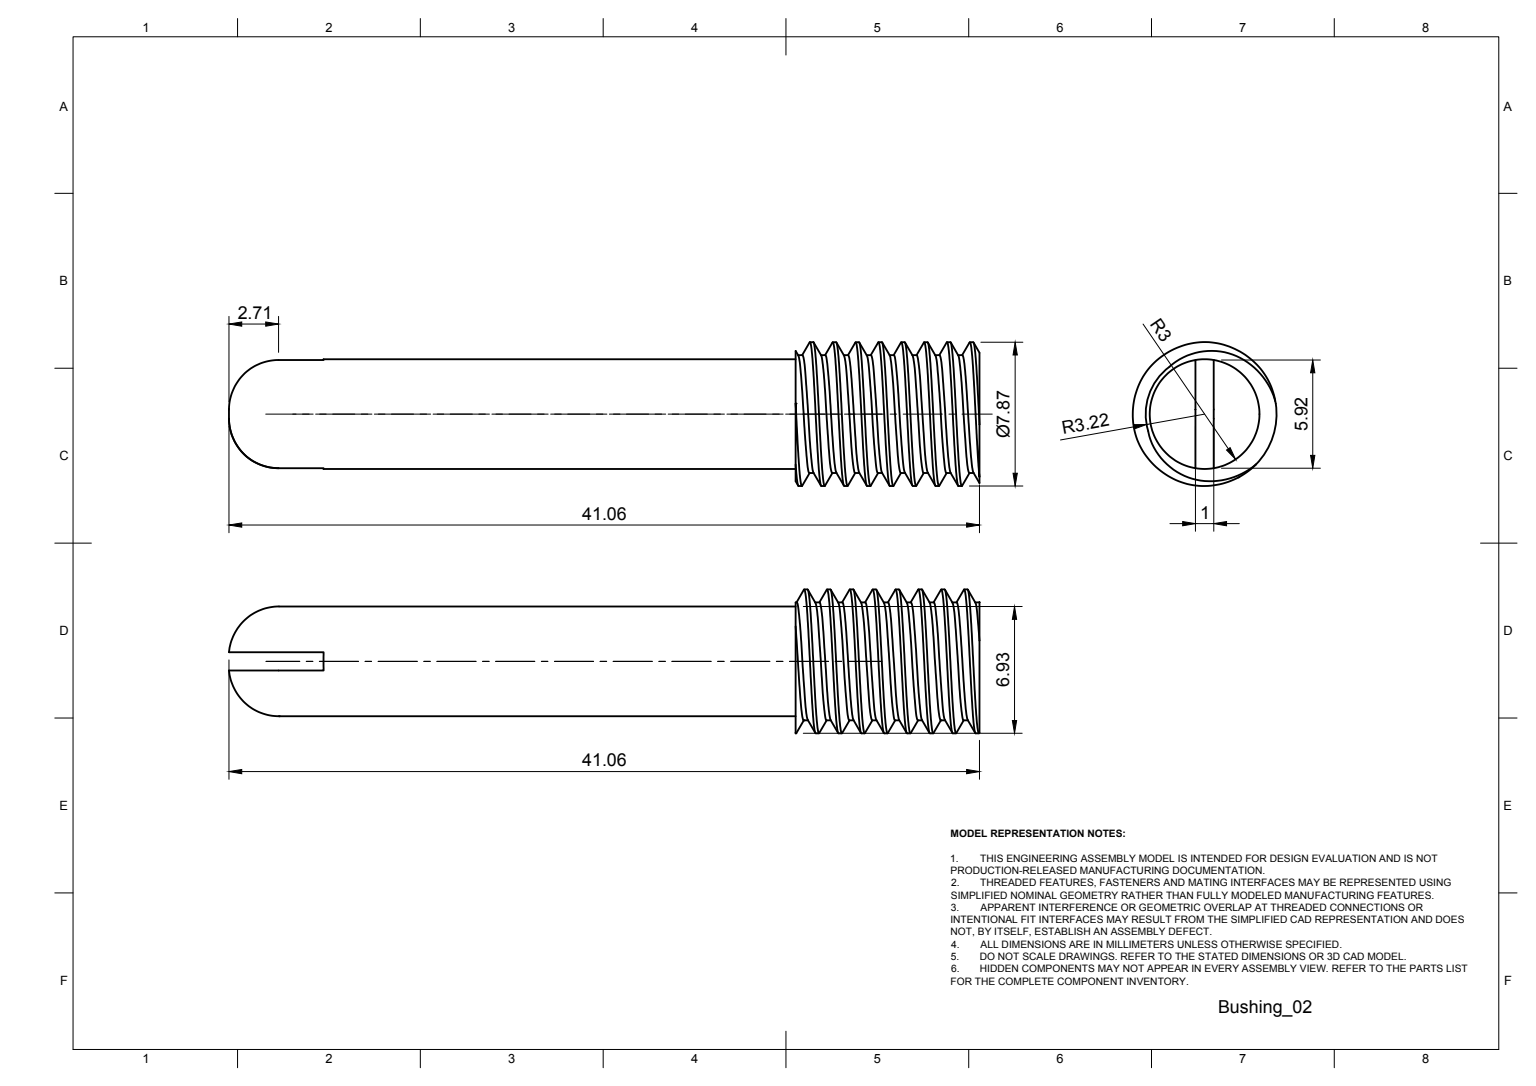
ISO-10303-21;
HEADER;
/* Generated by software containing ST-Developer
 * from STEP Tools, Inc. (www.steptools.com) 
 */

FILE_DESCRIPTION(
/* description */ (''),
/* implementation_level */ '2;1');

FILE_NAME(
/* name */ 'Bushing_02.step',
/* time_stamp */ '2026-10-06T12:52:28-07:00',
/* author */ (''),
/* organization */ (''),
/* preprocessor_version */ 'ST-DEVELOPER v20.2',
/* originating_system */ 'Autodesk Translation Framework v15.15.0.0',
/* authorisation */ '');

FILE_SCHEMA (('AUTOMOTIVE_DESIGN { 1 0 10303 214 3 1 1 }'));
ENDSEC;

DATA;
#10=MECHANICAL_DESIGN_GEOMETRIC_PRESENTATION_REPRESENTATION('',(#78),#34403);
#51=B_SPLINE_SURFACE_WITH_KNOTS('',3,3,((#24901,#24902,#24903,#24904,#24905,
#24906,#24907,#24908,#24909),(#24910,#24911,#24912,#24913,#24914,#24915,
#24916,#24917,#24918),(#24919,#24920,#24921,#24922,#24923,#24924,#24925,
#24926,#24927),(#24928,#24929,#24930,#24931,#24932,#24933,#24934,#24935,
#24936),(#24937,#24938,#24939,#24940,#24941,#24942,#24943,#24944,#24945)),
 .UNSPECIFIED.,.F.,.F.,.F.,(4,1,4),(4,1,1,1,1,1,4),(-2.3129491492736E-5,
0.571428571428571,1.),(-0.0392722361364195,-0.0280568820761978,-0.00562617395575443,
0.00558918010446727,0.016804534164689,0.0280198882249107,0.0392352422851324),
 .UNSPECIFIED.);
#52=B_SPLINE_SURFACE_WITH_KNOTS('',3,3,((#25116,#25117,#25118,#25119,#25120,
#25121,#25122,#25123,#25124,#25125),(#25126,#25127,#25128,#25129,#25130,
#25131,#25132,#25133,#25134,#25135),(#25136,#25137,#25138,#25139,#25140,
#25141,#25142,#25143,#25144,#25145),(#25146,#25147,#25148,#25149,#25150,
#25151,#25152,#25153,#25154,#25155),(#25156,#25157,#25158,#25159,#25160,
#25161,#25162,#25163,#25164,#25165)),.UNSPECIFIED.,.F.,.F.,.F.,(4,1,4),
(4,1,1,1,1,1,1,4),(-2.35337502838191E-5,0.571428571428571,1.),(-0.0392722361364195,
-0.0280568820761979,-0.0168415280159762,-0.00562617395575452,0.00558918010446715,
0.0168045341646888,0.0280198882249105,0.0392352422851322),.UNSPECIFIED.);
#53=B_SPLINE_SURFACE_WITH_KNOTS('',3,3,((#25200,#25201,#25202,#25203,#25204,
#25205,#25206,#25207,#25208,#25209,#25210,#25211,#25212,#25213,#25214,#25215,
#25216,#25217,#25218,#25219,#25220,#25221,#25222,#25223,#25224,#25225,#25226,
#25227,#25228,#25229,#25230,#25231,#25232,#25233,#25234,#25235,#25236,#25237,
#25238,#25239,#25240,#25241,#25242,#25243,#25244,#25245,#25246,#25247,#25248,
#25249,#25250,#25251,#25252,#25253,#25254,#25255),(#25256,#25257,#25258,
#25259,#25260,#25261,#25262,#25263,#25264,#25265,#25266,#25267,#25268,#25269,
#25270,#25271,#25272,#25273,#25274,#25275,#25276,#25277,#25278,#25279,#25280,
#25281,#25282,#25283,#25284,#25285,#25286,#25287,#25288,#25289,#25290,#25291,
#25292,#25293,#25294,#25295,#25296,#25297,#25298,#25299,#25300,#25301,#25302,
#25303,#25304,#25305,#25306,#25307,#25308,#25309,#25310,#25311),(#25312,
#25313,#25314,#25315,#25316,#25317,#25318,#25319,#25320,#25321,#25322,#25323,
#25324,#25325,#25326,#25327,#25328,#25329,#25330,#25331,#25332,#25333,#25334,
#25335,#25336,#25337,#25338,#25339,#25340,#25341,#25342,#25343,#25344,#25345,
#25346,#25347,#25348,#25349,#25350,#25351,#25352,#25353,#25354,#25355,#25356,
#25357,#25358,#25359,#25360,#25361,#25362,#25363,#25364,#25365,#25366,#25367),
(#25368,#25369,#25370,#25371,#25372,#25373,#25374,#25375,#25376,#25377,
#25378,#25379,#25380,#25381,#25382,#25383,#25384,#25385,#25386,#25387,#25388,
#25389,#25390,#25391,#25392,#25393,#25394,#25395,#25396,#25397,#25398,#25399,
#25400,#25401,#25402,#25403,#25404,#25405,#25406,#25407,#25408,#25409,#25410,
#25411,#25412,#25413,#25414,#25415,#25416,#25417,#25418,#25419,#25420,#25421,
#25422,#25423)),.UNSPECIFIED.,.F.,.F.,.F.,(4,4),(4,1,1,1,1,1,1,1,1,1,1,
1,1,1,1,1,1,1,1,1,1,1,1,1,1,1,1,1,1,1,1,1,1,1,1,1,1,1,1,1,1,1,1,1,1,1,1,
1,1,1,1,1,1,4),(-0.000662226835936772,0.0823162805313219),(-97.5343202090122,
-96.5415235325365,-95.5487268560609,-94.5559301795852,-93.5631335031096,
-92.570336826634,-91.5775401501583,-90.5847434736827,-89.591946797207,-88.5991501207314,
-87.6063534442557,-86.6135567677801,-85.6207600913045,-84.6279634148288,
-83.6351667383532,-82.6423700618775,-81.6495733854019,-80.6567767089262,
-79.6639800324506,-78.671183355975,-77.6783866794993,-76.6855900030237,
-75.692793326548,-74.6999966500724,-73.7071999735967,-72.7144032971211,
-71.7216066206455,-70.7288099441698,-69.7360132676942,-68.7432165912185,
-67.7504199147429,-66.7576232382672,-65.7648265617916,-64.772029885316,
-63.7792332088403,-62.7864365323647,-61.793639855889,-60.8008431794134,
-59.8080465029377,-58.8152498264621,-57.8224531499865,-56.8296564735108,
-55.8368597970352,-54.8440631205595,-53.8512664440839,-52.8584697676082,
-51.8656730911326,-50.872876414657,-49.8800797381813,-48.8872830617057,
-47.89448638523,-46.9016897087544,-45.9088930322787,-44.9154341289673),
 .UNSPECIFIED.);
#54=B_SPLINE_SURFACE_WITH_KNOTS('',3,3,((#25626,#25627,#25628,#25629,#25630,
#25631,#25632,#25633,#25634,#25635,#25636,#25637,#25638,#25639,#25640,#25641,
#25642,#25643,#25644,#25645,#25646,#25647,#25648,#25649,#25650,#25651,#25652,
#25653,#25654,#25655,#25656,#25657,#25658,#25659,#25660,#25661,#25662,#25663,
#25664,#25665,#25666,#25667,#25668,#25669,#25670,#25671,#25672,#25673,#25674,
#25675,#25676,#25677,#25678,#25679,#25680,#25681),(#25682,#25683,#25684,
#25685,#25686,#25687,#25688,#25689,#25690,#25691,#25692,#25693,#25694,#25695,
#25696,#25697,#25698,#25699,#25700,#25701,#25702,#25703,#25704,#25705,#25706,
#25707,#25708,#25709,#25710,#25711,#25712,#25713,#25714,#25715,#25716,#25717,
#25718,#25719,#25720,#25721,#25722,#25723,#25724,#25725,#25726,#25727,#25728,
#25729,#25730,#25731,#25732,#25733,#25734,#25735,#25736,#25737),(#25738,
#25739,#25740,#25741,#25742,#25743,#25744,#25745,#25746,#25747,#25748,#25749,
#25750,#25751,#25752,#25753,#25754,#25755,#25756,#25757,#25758,#25759,#25760,
#25761,#25762,#25763,#25764,#25765,#25766,#25767,#25768,#25769,#25770,#25771,
#25772,#25773,#25774,#25775,#25776,#25777,#25778,#25779,#25780,#25781,#25782,
#25783,#25784,#25785,#25786,#25787,#25788,#25789,#25790,#25791,#25792,#25793),
(#25794,#25795,#25796,#25797,#25798,#25799,#25800,#25801,#25802,#25803,
#25804,#25805,#25806,#25807,#25808,#25809,#25810,#25811,#25812,#25813,#25814,
#25815,#25816,#25817,#25818,#25819,#25820,#25821,#25822,#25823,#25824,#25825,
#25826,#25827,#25828,#25829,#25830,#25831,#25832,#25833,#25834,#25835,#25836,
#25837,#25838,#25839,#25840,#25841,#25842,#25843,#25844,#25845,#25846,#25847,
#25848,#25849)),.UNSPECIFIED.,.F.,.F.,.F.,(4,4),(4,1,1,1,1,1,1,1,1,1,1,
1,1,1,1,1,1,1,1,1,1,1,1,1,1,1,1,1,1,1,1,1,1,1,1,1,1,1,1,1,1,1,1,1,1,1,1,
1,1,1,1,1,1,4),(-0.000307057037193035,0.0826748885905267),(-94.2345010139676,
-93.2410420546399,-92.2482453781643,-91.2554487016887,-90.2626520252132,
-89.2698553487376,-88.277058672262,-87.2842619957864,-86.2914653193108,
-85.2986686428353,-84.3058719663597,-83.3130752898841,-82.3202786134085,
-81.327481936933,-80.3346852604574,-79.3418885839818,-78.3490919075062,
-77.3562952310307,-76.3634985545551,-75.3707018780795,-74.3779052016039,
-73.3851085251283,-72.3923118486528,-71.3995151721772,-70.4067184957016,
-69.413921819226,-68.4211251427505,-67.4283284662749,-66.4355317897993,
-65.4427351133237,-64.4499384368482,-63.4571417603726,-62.464345083897,
-61.4715484074214,-60.4787517309458,-59.4859550544703,-58.4931583779947,
-57.5003617015191,-56.5075650250435,-55.514768348568,-54.5219716720924,
-53.5291749956168,-52.5363783191412,-51.5435816426657,-50.5507849661901,
-49.5579882897145,-48.5651916132389,-47.5723949367633,-46.5795982602878,
-45.5868015838122,-44.5940049073366,-43.601208230861,-42.6084115543855,
-41.6156148779099),.UNSPECIFIED.);
#62=SHAPE_REPRESENTATION_RELATIONSHIP('SRR','None',#34440,#70);
#70=ADVANCED_BREP_SHAPE_REPRESENTATION('',(#86),#34400);
#78=STYLED_ITEM('',(#34484),#86);
#86=MANIFOLD_SOLID_BREP('Body1',#4387);
#101=FACE_BOUND('',#839,.T.);
#139=PLANE('',#4595);
#140=PLANE('',#4601);
#141=PLANE('',#4602);
#142=PLANE('',#4603);
#199=CIRCLE('',#4581,3.22275);
#200=CIRCLE('',#4590,3.933);
#201=CIRCLE('',#4591,3.94307276060078);
#202=CIRCLE('',#4592,3.933);
#203=CIRCLE('',#4594,3.22275);
#204=CIRCLE('',#4596,24.5);
#205=CIRCLE('',#4598,3.);
#206=CIRCLE('',#4600,24.5);
#577=FACE_OUTER_BOUND('',#820,.T.);
#578=FACE_OUTER_BOUND('',#821,.T.);
#579=FACE_OUTER_BOUND('',#822,.T.);
#580=FACE_OUTER_BOUND('',#823,.T.);
#581=FACE_OUTER_BOUND('',#824,.T.);
#582=FACE_OUTER_BOUND('',#825,.T.);
#583=FACE_OUTER_BOUND('',#826,.T.);
#584=FACE_OUTER_BOUND('',#827,.T.);
#585=FACE_OUTER_BOUND('',#828,.T.);
#586=FACE_OUTER_BOUND('',#829,.T.);
#587=FACE_OUTER_BOUND('',#830,.T.);
#588=FACE_OUTER_BOUND('',#831,.T.);
#589=FACE_OUTER_BOUND('',#832,.T.);
#590=FACE_OUTER_BOUND('',#833,.T.);
#591=FACE_OUTER_BOUND('',#834,.T.);
#592=FACE_OUTER_BOUND('',#835,.T.);
#593=FACE_OUTER_BOUND('',#836,.T.);
#594=FACE_OUTER_BOUND('',#837,.T.);
#595=FACE_OUTER_BOUND('',#838,.T.);
#596=FACE_OUTER_BOUND('',#840,.T.);
#820=EDGE_LOOP('',(#3083,#3084,#3085,#3086));
#821=EDGE_LOOP('',(#3087,#3088,#3089,#3090,#3091));
#822=EDGE_LOOP('',(#3092,#3093,#3094,#3095,#3096,#3097));
#823=EDGE_LOOP('',(#3098,#3099,#3100,#3101));
#824=EDGE_LOOP('',(#3102,#3103,#3104,#3105,#3106,#3107));
#825=EDGE_LOOP('',(#3108,#3109,#3110,#3111));
#826=EDGE_LOOP('',(#3112,#3113,#3114,#3115,#3116,#3117));
#827=EDGE_LOOP('',(#3118,#3119,#3120,#3121,#3122));
#828=EDGE_LOOP('',(#3123,#3124,#3125,#3126,#3127,#3128,#3129,#3130,#3131,
#3132,#3133,#3134,#3135,#3136,#3137,#3138,#3139,#3140,#3141,#3142,#3143));
#829=EDGE_LOOP('',(#3144,#3145,#3146,#3147,#3148));
#830=EDGE_LOOP('',(#3149,#3150,#3151,#3152));
#831=EDGE_LOOP('',(#3153,#3154,#3155,#3156,#3157,#3158));
#832=EDGE_LOOP('',(#3159,#3160,#3161,#3162,#3163,#3164,#3165,#3166,#3167,
#3168,#3169,#3170));
#833=EDGE_LOOP('',(#3171,#3172,#3173,#3174,#3175));
#834=EDGE_LOOP('',(#3176,#3177,#3178,#3179));
#835=EDGE_LOOP('',(#3180,#3181,#3182,#3183,#3184,#3185));
#836=EDGE_LOOP('',(#3186,#3187,#3188,#3189,#3190,#3191,#3192,#3193,#3194,
#3195,#3196,#3197,#3198,#3199,#3200,#3201,#3202,#3203,#3204,#3205,#3206,
#3207,#3208,#3209,#3210,#3211));
#837=EDGE_LOOP('',(#3212,#3213,#3214,#3215,#3216,#3217,#3218,#3219,#3220,
#3221,#3222,#3223,#3224,#3225,#3226,#3227,#3228,#3229,#3230,#3231,#3232,
#3233,#3234,#3235,#3236,#3237));
#838=EDGE_LOOP('',(#3238,#3239,#3240,#3241,#3242));
#839=EDGE_LOOP('',(#3243));
#840=EDGE_LOOP('',(#3244,#3245,#3246,#3247,#3248));
#1053=LINE('',#19195,#1190);
#1054=LINE('',#19338,#1191);
#1055=LINE('',#19566,#1192);
#1056=LINE('',#19867,#1193);
#1057=LINE('',#20213,#1194);
#1058=LINE('',#20565,#1195);
#1059=LINE('',#20897,#1196);
#1060=LINE('',#21274,#1197);
#1061=LINE('',#24987,#1198);
#1062=LINE('',#24990,#1199);
#1063=LINE('',#24993,#1200);
#1064=LINE('',#25047,#1201);
#1065=LINE('',#25063,#1202);
#1066=LINE('',#25114,#1203);
#1067=LINE('',#25196,#1204);
#1190=VECTOR('',#5246,3.22275);
#1191=VECTOR('',#5251,3.22275);
#1192=VECTOR('',#5254,3.22275);
#1193=VECTOR('',#5257,3.22275);
#1194=VECTOR('',#5260,3.22275);
#1195=VECTOR('',#5263,3.22275);
#1196=VECTOR('',#5266,3.22275);
#1197=VECTOR('',#5269,3.22275);
#1198=VECTOR('',#5282,10.);
#1199=VECTOR('',#5285,10.);
#1200=VECTOR('',#5288,10.);
#1201=VECTOR('',#5291,10.);
#1202=VECTOR('',#5292,10.);
#1203=VECTOR('',#5293,3.);
#1204=VECTOR('',#5296,10.);
#1410=B_SPLINE_CURVE_WITH_KNOTS('',3,(#19197,#19198,#19199,#19200,#19201,
#19202,#19203,#19204,#19205,#19206,#19207,#19208,#19209,#19210,#19211,#19212,
#19213,#19214,#19215,#19216,#19217,#19218,#19219,#19220,#19221,#19222,#19223,
#19224,#19225,#19226,#19227,#19228,#19229,#19230,#19231,#19232,#19233,#19234,
#19235,#19236,#19237,#19238,#19239,#19240,#19241,#19242,#19243,#19244,#19245,
#19246,#19247,#19248,#19249,#19250,#19251,#19252,#19253,#19254,#19255,#19256,
#19257,#19258,#19259,#19260,#19261,#19262,#19263,#19264,#19265,#19266,#19267,
#19268,#19269,#19270,#19271,#19272,#19273,#19274),.UNSPECIFIED.,.F.,.F.,
(4,2,2,2,2,2,2,2,2,2,2,2,2,2,2,2,2,2,2,2,2,2,2,2,2,2,2,2,2,2,2,2,2,2,2,
2,2,2,4),(-0.953586899306873,-0.946224083901339,-0.939681248602814,-0.933646614330381,
-0.924287213729251,-0.88833783922987,-0.804035161913967,-0.788327368237523,
-0.778740839088327,-0.768154224228326,-0.752801038121388,-0.691121741172027,
-0.635518435315854,-0.624462413541429,-0.618082999395715,-0.611911752838689,
-0.60200076655729,-0.589720784215698,-0.562242711762516,-0.486315971197755,
-0.46886052902349,-0.457800984209137,-0.447137732981836,-0.431855739492939,
-0.37573088153337,-0.313542424627404,-0.30302882313823,-0.296702133009702,
-0.290241676772455,-0.279315169359953,-0.265353516421564,-0.230988909071748,
-0.168154569303192,-0.151167359383941,-0.140141098841724,-0.129305786003328,
-0.11338295845748,-0.0538958793772908,-0.00526464879914939),
 .UNSPECIFIED.);
#1411=B_SPLINE_CURVE_WITH_KNOTS('',3,(#19277,#19278,#19279,#19280,#19281,
#19282,#19283,#19284,#19285,#19286,#19287,#19288,#19289,#19290,#19291,#19292,
#19293,#19294,#19295,#19296,#19297,#19298,#19299,#19300,#19301,#19302,#19303,
#19304,#19305,#19306,#19307,#19308,#19309,#19310,#19311,#19312,#19313,#19314,
#19315,#19316,#19317,#19318,#19319,#19320,#19321,#19322,#19323,#19324,#19325,
#19326,#19327,#19328,#19329,#19330,#19331,#19332,#19333,#19334),
 .UNSPECIFIED.,.F.,.F.,(4,3,3,3,3,3,3,3,3,3,3,3,3,3,3,3,3,3,3,4),(-94.2338387311155,
-94.1386227061935,-94.0434628204143,-93.9483368145334,-93.853196460553,
-93.7580426009854,-93.6628550280585,-93.567613507008,-93.4722330639492,
-93.376774672444,-93.2811517509658,-93.2410420546399,-93.1487193791218,
-93.0565224071019,-92.9644252665555,-92.8724021885971,-92.7804134444312,
-92.6884474321017,-92.5964417156794,-92.5246180830661),.UNSPECIFIED.);
#1412=B_SPLINE_CURVE_WITH_KNOTS('',3,(#19339,#19340,#19341,#19342,#19343,
#19344,#19345,#19346,#19347,#19348,#19349,#19350,#19351,#19352,#19353,#19354,
#19355,#19356,#19357,#19358,#19359,#19360,#19361,#19362,#19363,#19364,#19365,
#19366,#19367,#19368,#19369,#19370,#19371,#19372,#19373,#19374,#19375,#19376,
#19377,#19378,#19379,#19380,#19381,#19382,#19383,#19384,#19385,#19386,#19387,
#19388,#19389,#19390,#19391,#19392,#19393,#19394,#19395,#19396,#19397,#19398,
#19399,#19400,#19401,#19402,#19403,#19404,#19405,#19406,#19407,#19408,#19409,
#19410,#19411,#19412,#19413,#19414,#19415,#19416,#19417,#19418,#19419,#19420,
#19421,#19422,#19423,#19424,#19425,#19426,#19427,#19428,#19429,#19430,#19431,
#19432,#19433,#19434,#19435,#19436,#19437,#19438,#19439,#19440,#19441,#19442,
#19443,#19444,#19445,#19446,#19447,#19448,#19449,#19450,#19451,#19452,#19453,
#19454,#19455,#19456,#19457,#19458,#19459,#19460,#19461,#19462,#19463,#19464,
#19465,#19466,#19467,#19468,#19469,#19470,#19471,#19472,#19473,#19474,#19475,
#19476,#19477,#19478,#19479,#19480,#19481,#19482,#19483,#19484,#19485,#19486,
#19487,#19488,#19489,#19490,#19491,#19492,#19493,#19494,#19495,#19496,#19497,
#19498,#19499,#19500,#19501,#19502,#19503,#19504,#19505,#19506),
 .UNSPECIFIED.,.F.,.F.,(4,2,2,2,2,2,2,2,2,2,2,2,2,2,2,2,2,2,2,2,2,2,2,2,
2,2,2,2,2,2,2,2,2,2,2,2,2,2,2,2,2,2,2,2,2,2,2,2,2,2,2,2,2,2,2,2,2,2,2,2,
2,2,2,2,2,2,2,2,2,2,2,2,2,2,2,2,2,2,2,2,2,2,2,4),(-2.98314948647837,-2.92931927299001,
-2.87847831664238,-2.86854692686803,-2.86238048863821,-2.85598188384405,
-2.84491835823975,-2.78906969762543,-2.72775918925124,-2.71234213768023,
-2.70169927312789,-2.69075927697716,-2.67371484620561,-2.60849645012846,
-2.55783247712985,-2.54788253120033,-2.54171277534183,-2.53531903720203,
-2.52428009071603,-2.46776648675201,-2.42715250362434,-2.40830069600736,
-2.39233125418358,-2.38158948252091,-2.37076866644709,-2.35436708268367,
-2.28314135391068,-2.25155038995474,-2.23824842378604,-2.22773649064595,
-2.22145110781181,-2.21594582391548,-2.20632739871659,-2.16701154076078,
-2.11294395468491,-2.0912376827486,-2.07353264494282,-2.06246402564764,
-2.05201402271332,-2.0394863417041,-2.0061953134929,-1.99990582558898,-1.94050245591194,
-1.92231800668791,-1.90911550001101,-1.90229003981063,-1.89634126079205,
-1.88902652801476,-1.86895400933939,-1.80951506282857,-1.77897954822343,
-1.75649112348816,-1.74453409286566,-1.73422264512113,-1.72122725251755,
-1.69233732141656,-1.64649274907083,-1.59931226565268,-1.58749550650159,
-1.58094516716533,-1.57487942726118,-1.5654739075449,-1.52927851683261,
-1.44595504899421,-1.43008910319921,-1.42043269512404,-1.4097841233922,
-1.39436252007387,-1.33286583781343,-1.27719596698061,-1.26611968641952,
-1.25971350417248,-1.25352405459038,-1.24354070919542,-1.23113688245437,
-1.20315529593337,-1.12441168013372,-1.10911634905808,-1.09858349711662,
-1.08760467199154,-1.07043920126136,-1.02023819202142,-0.957986996023974,
-0.953586899306873),.UNSPECIFIED.);
#1413=B_SPLINE_CURVE_WITH_KNOTS('',3,(#19508,#19509,#19510,#19511,#19512,
#19513,#19514,#19515,#19516,#19517,#19518,#19519,#19520,#19521,#19522,#19523,
#19524,#19525,#19526,#19527,#19528,#19529,#19530,#19531,#19532,#19533,#19534,
#19535,#19536,#19537,#19538,#19539,#19540,#19541,#19542,#19543,#19544,#19545,
#19546,#19547,#19548,#19549,#19550,#19551,#19552,#19553),.UNSPECIFIED.,
 .F.,.F.,(4,3,3,3,3,3,3,3,3,3,3,3,3,3,3,4),(-92.5246180830661,-92.4325102353362,
-92.3402421939541,-92.2482453781643,-92.1550137134133,-92.0619070601935,
-91.9688980138682,-91.8759565736399,-91.78305006345,-91.6901538610218,-91.5972433592587,
-91.5042366896818,-91.4111786089953,-91.3179720140179,-91.2554487016887,
-91.106186954104),.UNSPECIFIED.);
#1414=B_SPLINE_CURVE_WITH_KNOTS('',3,(#19554,#19555,#19556,#19557,#19558,
#19559,#19560,#19561,#19562),.UNSPECIFIED.,.F.,.F.,(4,1,1,1,1,1,4),(-91.1061804086756,
-90.2626520252132,-89.2698553487376,-88.277058672262,-87.2842619957864,
-86.2914653193108,-86.2406734486321),.UNSPECIFIED.);
#1415=B_SPLINE_CURVE_WITH_KNOTS('',3,(#19568,#19569,#19570,#19571,#19572,
#19573,#19574,#19575,#19576,#19577,#19578,#19579,#19580,#19581,#19582,#19583,
#19584,#19585,#19586,#19587,#19588,#19589,#19590,#19591,#19592,#19593,#19594,
#19595,#19596,#19597,#19598,#19599,#19600,#19601,#19602,#19603,#19604,#19605,
#19606,#19607,#19608,#19609,#19610,#19611,#19612,#19613,#19614,#19615,#19616,
#19617,#19618,#19619,#19620,#19621,#19622,#19623,#19624,#19625,#19626,#19627,
#19628,#19629,#19630,#19631,#19632,#19633,#19634,#19635,#19636,#19637,#19638,
#19639,#19640,#19641,#19642,#19643,#19644,#19645,#19646,#19647,#19648,#19649,
#19650,#19651,#19652,#19653,#19654,#19655,#19656,#19657,#19658,#19659,#19660,
#19661,#19662,#19663,#19664,#19665,#19666,#19667,#19668,#19669,#19670,#19671,
#19672,#19673,#19674,#19675,#19676,#19677,#19678,#19679,#19680,#19681,#19682,
#19683,#19684,#19685,#19686,#19687,#19688,#19689,#19690,#19691,#19692,#19693,
#19694,#19695),.UNSPECIFIED.,.F.,.F.,(4,2,2,2,2,2,2,2,2,2,2,2,2,2,2,2,2,
2,2,2,2,2,2,2,2,2,2,2,2,2,2,2,2,2,2,2,2,2,2,2,2,2,2,2,2,2,2,2,2,2,2,2,2,
2,2,2,2,2,2,2,2,2,2,4),(-1.57226653739125,-1.5335777974379,-1.51749976800245,
-1.50781260533011,-1.49720443964807,-1.48199362716857,-1.4271100079384,
-1.36376233553656,-1.35299538353744,-1.34665765102371,-1.34044105870802,
-1.33026081848513,-1.28036678994184,-1.21482587221898,-1.19781359925106,
-1.18687887704712,-1.17623012667664,-1.16078436208362,-1.09877281757955,
-1.04367999968674,-1.03258103848034,-1.02617467754542,-1.02001319481398,
-1.01010791778992,-0.958953801785455,-0.894272784649096,-0.877190705715183,
-0.866242485531937,-0.855602583965498,-0.840209857332201,-0.778575631347056,
-0.722936048969459,-0.711861685957521,-0.70546020493503,-0.699294513098806,
-0.689369054767423,-0.677054035431794,-0.649392216624609,-0.572613580933394,
-0.555994727226221,-0.545133285484477,-0.53442622969633,-0.518652195275346,
-0.459429796640774,-0.402070705637716,-0.391076790872994,-0.384691797229376,
-0.378513281994944,-0.368523491494722,-0.356101632547016,-0.328031571970327,
-0.24906421527631,-0.233758461195957,-0.223238986692471,-0.212293433018225,
-0.195226494574182,-0.145648423230977,-0.0814618760384713,-0.070400689902343,
-0.0640018345987939,-0.0578339732759233,-0.0513639077985467,-0.0362287903919722,
-0.000931521656303621),.UNSPECIFIED.);
#1416=B_SPLINE_CURVE_WITH_KNOTS('',3,(#19696,#19697,#19698,#19699,#19700,
#19701,#19702,#19703,#19704,#19705,#19706,#19707,#19708,#19709,#19710,#19711,
#19712,#19713,#19714,#19715,#19716,#19717,#19718,#19719,#19720,#19721,#19722,
#19723,#19724,#19725,#19726,#19727,#19728,#19729,#19730,#19731,#19732,#19733),
 .UNSPECIFIED.,.F.,.F.,(4,2,2,2,2,2,2,2,2,2,2,2,2,2,2,2,2,2,4),(-3.44144283943813,
-3.36915521246843,-3.35372024630458,-3.34307352431673,-3.33213640148464,
-3.31511101176518,-3.24965355552941,-3.19915704516472,-3.18922333268155,
-3.18305637047153,-3.17665726842006,-3.1655942456309,-3.10972609818714,
-3.04842654583021,-3.03301632354937,-3.02237360197422,-3.01142989848601,
-2.99437110190186,-2.98314948647837),.UNSPECIFIED.);
#1417=B_SPLINE_CURVE_WITH_KNOTS('',3,(#19735,#19736,#19737,#19738,#19739),
 .UNSPECIFIED.,.F.,.F.,(4,1,4),(-86.2406734486321,-85.2986686428353,-84.8230031757796),
 .UNSPECIFIED.);
#1418=B_SPLINE_CURVE_WITH_KNOTS('',3,(#19740,#19741,#19742,#19743,#19744,
#19745,#19746,#19747,#19748,#19749,#19750,#19751,#19752,#19753,#19754,#19755,
#19756,#19757,#19758,#19759,#19760,#19761,#19762,#19763,#19764,#19765,#19766,
#19767,#19768,#19769,#19770,#19771,#19772,#19773,#19774,#19775,#19776,#19777,
#19778,#19779,#19780,#19781,#19782,#19783,#19784,#19785,#19786,#19787,#19788,
#19789,#19790,#19791,#19792,#19793,#19794,#19795,#19796,#19797,#19798,#19799,
#19800,#19801,#19802,#19803,#19804,#19805,#19806,#19807,#19808,#19809,#19810,
#19811,#19812,#19813,#19814,#19815,#19816,#19817,#19818,#19819,#19820,#19821,
#19822,#19823,#19824,#19825,#19826,#19827,#19828,#19829,#19830,#19831,#19832,
#19833,#19834,#19835,#19836,#19837,#19838,#19839,#19840,#19841,#19842,#19843,
#19844,#19845,#19846,#19847,#19848,#19849,#19850,#19851,#19852,#19853,#19854,
#19855,#19856,#19857,#19858,#19859,#19860,#19861,#19862,#19863),
 .UNSPECIFIED.,.F.,.F.,(4,2,2,2,2,2,2,2,2,2,2,2,2,2,2,2,2,2,2,2,2,2,2,2,
2,2,2,2,2,2,2,2,2,2,2,2,2,2,2,2,2,2,2,2,2,2,2,2,2,2,2,2,2,2,2,2,2,2,2,2,
2,4),(-4.05949121043388,-4.05121437145667,-4.04065847954402,-4.02381103819477,
-3.95897828953223,-3.90811934396657,-3.89820260742545,-3.8920396257056,
-3.88563807260872,-3.87455861457586,-3.81920431913373,-3.75742003728717,
-3.74201743687854,-3.7313777449435,-3.72043543181097,-3.70337527512879,
-3.63838157000884,-3.58749127890204,-3.5775671792347,-3.57140291795658,
-3.56500278009261,-3.55393200139329,-3.49833852441203,-3.4368258288365,
-3.42140106480513,-3.41075658377407,-3.39981778691892,-3.38278102810115,
-3.31749947334804,-3.26754902845121,-3.25726826635629,-3.25103138547184,
-3.24471713356767,-3.23406214171634,-3.17336971297882,-3.13494613533587,
-3.11665137224682,-3.10103194361361,-3.09035352395009,-3.07946036874197,
-3.06266587013177,-2.99480056759295,-2.94745285384507,-2.93689327516753,
-2.93059879932187,-2.92434353568057,-2.91397336918307,-2.85079466441326,
-2.81356101937502,-2.79557917663882,-2.78015734987967,-2.76951317962702,
-2.75857335392659,-2.74153221996127,-2.67627961911833,-2.62565067878737,
-2.61570117934235,-2.60953128798207,-2.60313694386948,-2.59209545593267,
-2.53566520876919,-2.48818497945327),.UNSPECIFIED.);
#1419=B_SPLINE_CURVE_WITH_KNOTS('',3,(#19868,#19869,#19870,#19871,#19872,
#19873,#19874,#19875,#19876,#19877,#19878,#19879,#19880,#19881,#19882,#19883,
#19884,#19885,#19886,#19887,#19888,#19889,#19890,#19891,#19892,#19893,#19894,
#19895,#19896,#19897,#19898,#19899,#19900,#19901,#19902,#19903,#19904,#19905,
#19906,#19907,#19908,#19909,#19910,#19911,#19912,#19913,#19914,#19915,#19916,
#19917,#19918,#19919,#19920,#19921,#19922,#19923,#19924,#19925,#19926,#19927,
#19928,#19929,#19930,#19931,#19932,#19933,#19934,#19935,#19936,#19937,#19938,
#19939,#19940,#19941,#19942,#19943,#19944,#19945,#19946,#19947,#19948,#19949,
#19950,#19951,#19952,#19953,#19954,#19955,#19956,#19957,#19958,#19959,#19960,
#19961,#19962,#19963,#19964,#19965,#19966,#19967,#19968,#19969,#19970,#19971,
#19972,#19973,#19974,#19975,#19976,#19977,#19978,#19979,#19980,#19981,#19982,
#19983,#19984,#19985,#19986,#19987,#19988,#19989,#19990,#19991,#19992,#19993,
#19994,#19995,#19996,#19997,#19998,#19999,#20000,#20001,#20002,#20003,#20004,
#20005,#20006,#20007,#20008,#20009,#20010,#20011,#20012,#20013,#20014,#20015,
#20016,#20017,#20018,#20019,#20020,#20021,#20022,#20023,#20024,#20025,#20026,
#20027,#20028,#20029,#20030,#20031,#20032,#20033,#20034,#20035,#20036,#20037,
#20038,#20039,#20040,#20041),.UNSPECIFIED.,.F.,.F.,(4,2,2,2,2,2,2,2,2,2,
2,2,2,2,2,2,2,2,2,2,2,2,2,2,2,2,2,2,2,2,2,2,2,2,2,2,2,2,2,2,2,2,2,2,2,2,
2,2,2,2,2,2,2,2,2,2,2,2,2,2,2,2,2,2,2,2,2,2,2,2,2,2,2,2,2,2,2,2,2,2,2,2,
2,2,2,2,4),(-3.60148803627134,-3.59726790795439,-3.59098685437188,-3.58471907313518,
-3.57428766404847,-3.51164348509371,-3.45559099116675,-3.44034678171266,
-3.42973359074539,-3.41875011562731,-3.40147579935169,-3.34043366880226,
-3.30310540362232,-3.28205654415774,-3.27398152357135,-3.26810771974208,
-3.26090656586411,-3.2456415178696,-3.18703553787276,-3.13855425810496,
-3.1216363120744,-3.11072040881662,-3.10018385387515,-3.0847683875459,-3.00651772233112,
-2.97812444519445,-2.96561919642675,-2.95558062126107,-2.94939320865812,
-2.94302219732592,-2.93209232466705,-2.87403556224324,-2.83428541792364,
-2.81565086864161,-2.79981791455114,-2.78910164548746,-2.77825485553291,
-2.76170816630454,-2.69166204680768,-2.65949146606953,-2.64605245758614,
-2.63546067061529,-2.6291595684875,-2.62291078291482,-2.61257177018778,
-2.54912091334469,-2.5120150754806,-2.49406737179312,-2.47866721537971,
-2.46802690006783,-2.45708201518327,-2.4400135557156,-2.37510334330683,
-2.32419385495604,-2.31423984884152,-2.30806912114555,-2.30167618897554,
-2.29064106146257,-2.22197476329415,-2.18871569735013,-2.16492129885298,
-2.15273109663306,-2.1424291067809,-2.12971584634897,-2.10273105378269,
-2.02998606678719,-2.0016293028606,-1.99260960515907,-1.98667066811743,
-1.97999954768792,-1.96758725489158,-1.95090337602745,-1.90211662187695,
-1.85194585632104,-1.8369121508399,-1.82643866908472,-1.81542316901591,
-1.79798287416363,-1.74547920414441,-1.68411033096761,-1.67352430836737,
-1.66722415648816,-1.66097373936419,-1.65062802104306,-1.63760890563595,
-1.60717731235625,-1.57226653739125),.UNSPECIFIED.);
#1420=B_SPLINE_CURVE_WITH_KNOTS('',3,(#20042,#20043,#20044,#20045,#20046,
#20047,#20048,#20049,#20050,#20051,#20052,#20053,#20054,#20055,#20056,#20057,
#20058,#20059,#20060,#20061,#20062,#20063,#20064,#20065,#20066,#20067,#20068,
#20069,#20070,#20071,#20072,#20073,#20074,#20075,#20076,#20077,#20078,#20079,
#20080,#20081,#20082,#20083,#20084,#20085,#20086,#20087,#20088,#20089,#20090,
#20091,#20092,#20093,#20094,#20095,#20096,#20097,#20098,#20099,#20100,#20101,
#20102,#20103,#20104,#20105,#20106,#20107,#20108,#20109,#20110,#20111,#20112,
#20113,#20114,#20115,#20116,#20117,#20118,#20119,#20120,#20121,#20122,#20123,
#20124,#20125,#20126,#20127,#20128,#20129,#20130,#20131,#20132,#20133,#20134,
#20135,#20136,#20137,#20138,#20139,#20140,#20141,#20142,#20143,#20144,#20145,
#20146,#20147,#20148,#20149,#20150,#20151,#20152,#20153,#20154,#20155,#20156,
#20157,#20158,#20159,#20160,#20161,#20162,#20163,#20164,#20165,#20166,#20167,
#20168,#20169,#20170,#20171,#20172,#20173,#20174,#20175,#20176,#20177,#20178,
#20179,#20180,#20181,#20182,#20183,#20184,#20185,#20186,#20187,#20188,#20189,
#20190,#20191,#20192,#20193,#20194,#20195,#20196,#20197,#20198,#20199,#20200,
#20201,#20202,#20203,#20204,#20205,#20206,#20207,#20208,#20209),
 .UNSPECIFIED.,.F.,.F.,(4,2,2,2,2,2,2,2,2,2,2,2,2,2,2,2,2,2,2,2,2,2,2,2,
2,2,2,2,2,2,2,2,2,2,2,2,2,2,2,2,2,2,2,2,2,2,2,2,2,2,2,2,2,2,2,2,2,2,2,2,
2,2,2,2,2,2,2,2,2,2,2,2,2,2,2,2,2,2,2,2,2,2,2,4),(-2.48818497945327,-2.47661569284377,
-2.46041249231985,-2.44962867574266,-2.43885292257533,-2.42269402150062,
-2.34963196044359,-2.31891957880817,-2.30583089242212,-2.29544489121947,
-2.28918621756621,-2.28289464564112,-2.27235029868863,-2.21067864367937,
-2.15559329660223,-2.13955930085061,-2.12880625929744,-2.11799874145444,
-2.10166705448592,-2.02990196306529,-1.98730851207629,-1.97573932437658,
-1.96923692158684,-1.96314080965402,-1.95357264272231,-1.91386818576171,
-1.83704171514185,-1.81996554507048,-1.80901875051122,-1.79837854665767,
-1.78298224522728,-1.76503910564669,-1.72795555566859,-1.66437608378914,
-1.6540447671092,-1.64779725241036,-1.64149351545674,-1.63089127738814,
-1.61743622842379,-1.58519570479033,-1.51535388396843,-1.49878885307633,
-1.48793790926569,-1.47722314628574,-1.46140326307786,-1.40103999361036,
-1.3450610657836,-1.33399883001431,-1.32760001200728,-1.32143274143006,
-1.31149835160373,-1.26082229040495,-1.19564760626722,-1.17860471563187,
-1.16766389105049,-1.15701870553694,-1.14159547110918,-1.1236100980696,
-1.08636972622046,-1.02311542409142,-1.01274592372879,-1.00649036762245,
-1.00019460847225,-0.989631608162483,-0.941721342655347,-0.874629750026393,
-0.857760383650131,-0.846852232066049,-0.836182940761279,-0.820621411802712,
-0.761154441683342,-0.703549270177194,-0.692574275383058,-0.686193266407756,
-0.680011710962549,-0.670006535853517,-0.657558990906142,-0.629389598384432,
-0.550666233097892,-0.535325340491625,-0.524799982685431,-0.513863175707245,
-0.496842297440668,-0.458703963070235),.UNSPECIFIED.);
#1421=B_SPLINE_CURVE_WITH_KNOTS('',3,(#20215,#20216,#20217,#20218,#20219,
#20220,#20221,#20222,#20223,#20224,#20225,#20226,#20227,#20228,#20229,#20230,
#20231,#20232,#20233,#20234,#20235,#20236,#20237,#20238,#20239,#20240,#20241,
#20242,#20243,#20244,#20245,#20246,#20247,#20248,#20249,#20250,#20251,#20252,
#20253,#20254,#20255,#20256,#20257,#20258,#20259,#20260,#20261,#20262,#20263,
#20264,#20265,#20266,#20267,#20268,#20269,#20270,#20271,#20272,#20273,#20274,
#20275,#20276,#20277,#20278,#20279,#20280,#20281,#20282,#20283,#20284,#20285,
#20286,#20287,#20288,#20289,#20290,#20291,#20292,#20293,#20294,#20295,#20296,
#20297,#20298,#20299,#20300,#20301,#20302,#20303,#20304,#20305,#20306,#20307,
#20308,#20309,#20310,#20311,#20312,#20313,#20314,#20315,#20316,#20317,#20318,
#20319,#20320,#20321,#20322,#20323,#20324,#20325,#20326,#20327,#20328,#20329,
#20330,#20331,#20332,#20333,#20334,#20335,#20336,#20337,#20338,#20339,#20340,
#20341,#20342,#20343,#20344,#20345,#20346,#20347,#20348),.UNSPECIFIED.,
 .F.,.F.,(4,2,2,2,2,2,2,2,2,2,2,2,2,2,2,2,2,2,2,2,2,2,2,2,2,2,2,2,2,2,2,
2,2,2,2,2,2,2,2,2,2,2,2,2,2,2,2,2,2,2,2,2,2,2,2,2,2,2,2,2,2,2,2,2,2,2,4),
(-1.57270504429441,-1.57198597895571,-1.53184015506289,-1.4744178950004,
-1.46342781057866,-1.45704342558984,-1.4508638651289,-1.44086999371776,
-1.42844156890585,-1.40034729366256,-1.32143087815656,-1.30611622816268,
-1.29559480540958,-1.28465062268848,-1.26759324916272,-1.21809184782572,
-1.15729158777298,-1.14419135132274,-1.13738539355418,-1.13142607440303,
-1.12265609486979,-1.09531100949502,-1.03125066260997,-0.997509615877714,
-0.98493246552515,-0.974472652709664,-0.963426589679085,-0.945834993848146,
-0.924318436015176,-0.871329842578893,-0.830426302826506,-0.820785203293156,
-0.815276889046202,-0.808998247382131,-0.798520016701879,-0.785277148103801,
-0.753931042657932,-0.682243191223101,-0.665904305115668,-0.655094053629165,
-0.64433973007818,-0.628306893505015,-0.574149269053255,-0.511174379321276,
-0.500769824530627,-0.494506480797386,-0.488217178586173,-0.477687892439614,
-0.428977275730074,-0.362775320398643,-0.345817247349719,-0.334891381242875,
-0.324232895492104,-0.308739200514757,-0.290643425545204,-0.252992014084021,
-0.190575699323686,-0.180106656871352,-0.173829923488554,-0.167554150248785,
-0.157090098128878,-0.109028173875831,-0.0418274175576785,-0.0252966452826552,
-0.0143328742967741,-0.00723065120931022,-0.000931044346426293),
 .UNSPECIFIED.);
#1422=B_SPLINE_CURVE_WITH_KNOTS('',3,(#20349,#20350,#20351,#20352,#20353,
#20354,#20355,#20356,#20357,#20358,#20359,#20360,#20361,#20362,#20363,#20364,
#20365,#20366,#20367,#20368,#20369,#20370,#20371,#20372,#20373,#20374,#20375,
#20376,#20377,#20378,#20379,#20380,#20381,#20382,#20383,#20384,#20385,#20386),
 .UNSPECIFIED.,.F.,.F.,(4,2,2,2,2,2,2,2,2,2,2,2,2,2,2,2,2,2,4),(-4.05940163546454,
-4.0513614597985,-4.03929124303463,-3.97799719175202,-3.92748437027949,
-3.91747126369622,-3.91128897983749,-3.90491163882794,-3.89395098991898,
-3.83625920142476,-3.7778835028167,-3.76189126289714,-3.75114653873282,
-3.74033227188704,-3.72395993843194,-3.6525226917305,-3.62103886952059,
-3.60776360891426,-3.60148803627134),.UNSPECIFIED.);
#1423=B_SPLINE_CURVE_WITH_KNOTS('',3,(#20388,#20389,#20390,#20391,#20392,
#20393,#20394,#20395,#20396,#20397,#20398,#20399,#20400,#20401,#20402,#20403,
#20404,#20405,#20406,#20407,#20408,#20409,#20410,#20411,#20412,#20413,#20414,
#20415,#20416,#20417,#20418,#20419,#20420,#20421,#20422,#20423,#20424,#20425,
#20426,#20427,#20428,#20429,#20430,#20431,#20432,#20433),.UNSPECIFIED.,
 .F.,.F.,(4,2,2,2,2,2,2,2,2,2,2,2,2,2,2,2,2,2,2,2,2,2,4),(-0.458703963070235,
-0.4476103789344,-0.387390603287348,-0.373726897302928,-0.36681426866366,
-0.36088624078785,-0.352333693779791,-0.32719823278997,-0.274608647504632,
-0.229055324726366,-0.214134235080965,-0.203677569512926,-0.19262737818266,
-0.175011958392165,-0.153454737042513,-0.140085221830007,-0.0719338954249617,
-0.0547956271046257,-0.0472815868163417,-0.0414267321571205,-0.0356813677969033,
-0.0279552207881814,-0.000930590274443855),.UNSPECIFIED.);
#1424=B_SPLINE_CURVE_WITH_KNOTS('',3,(#20434,#20435,#20436,#20437,#20438,
#20439,#20440,#20441,#20442,#20443,#20444,#20445,#20446,#20447,#20448,#20449,
#20450,#20451,#20452,#20453,#20454,#20455,#20456,#20457,#20458,#20459,#20460,
#20461,#20462,#20463,#20464,#20465,#20466,#20467,#20468,#20469,#20470,#20471,
#20472,#20473,#20474,#20475,#20476,#20477,#20478,#20479,#20480,#20481,#20482,
#20483,#20484,#20485,#20486,#20487,#20488,#20489,#20490,#20491,#20492,#20493,
#20494,#20495,#20496,#20497,#20498,#20499,#20500,#20501,#20502,#20503,#20504,
#20505,#20506,#20507,#20508,#20509,#20510,#20511,#20512,#20513,#20514,#20515,
#20516,#20517,#20518,#20519,#20520,#20521,#20522,#20523,#20524,#20525,#20526,
#20527,#20528,#20529,#20530,#20531,#20532,#20533,#20534,#20535,#20536,#20537,
#20538,#20539,#20540,#20541,#20542,#20543,#20544,#20545,#20546,#20547,#20548,
#20549,#20550,#20551,#20552,#20553,#20554,#20555,#20556,#20557,#20558,#20559,
#20560,#20561),.UNSPECIFIED.,.F.,.F.,(4,2,2,2,2,2,2,2,2,2,2,2,2,2,2,2,2,
2,2,2,2,2,2,2,2,2,2,2,2,2,2,2,2,2,2,2,2,2,2,2,2,2,2,2,2,2,2,2,2,2,2,2,2,
2,2,2,2,2,2,2,2,2,2,4),(-4.06048203363518,-4.03025455645395,-3.9691349538326,
-3.95369424520963,-3.94304683352945,-3.9321116200381,-3.91509476425701,
-3.84955218125704,-3.79933143232759,-3.78929737786332,-3.78311059686391,
-3.77673781623578,-3.76580068005654,-3.70782017083285,-3.64915364962081,
-3.63340707851152,-3.62270589410659,-3.61184022793493,-3.59519396745887,
-3.51842926964027,-3.49076501195105,-3.47844946162652,-3.46852477553194,
-3.46235979182168,-3.45595900217838,-3.44488608818992,-3.3893318418027,
-3.32767918035704,-3.31229691148376,-3.30165956012622,-3.29071002293352,
-3.27361754916669,-3.19683072234816,-3.16975298762487,-3.15243990351045,
-3.14489903546282,-3.13962441374937,-3.13230314338034,-3.11633927545952,
-3.05838609218079,-3.0101994379,-2.99332016806537,-2.98241057334082,-2.97186714936823,
-2.95641724351904,-2.87838180616511,-2.83655159525338,-2.82690302107234,
-2.82079166632169,-2.81431345858978,-2.80286356868832,-2.75024228454491,
-2.68747732350124,-2.67156813817421,-2.66083741428753,-2.65000483326521,
-2.63353877133443,-2.55649529326159,-2.52876569107145,-2.51643269276606,
-2.50649735215666,-2.50033001830562,-2.49393150688731,-2.48879418648611),
 .UNSPECIFIED.);
#1425=B_SPLINE_CURVE_WITH_KNOTS('',3,(#20566,#20567,#20568,#20569,#20570,
#20571,#20572,#20573,#20574,#20575,#20576,#20577,#20578,#20579,#20580,#20581,
#20582,#20583,#20584,#20585,#20586,#20587,#20588,#20589,#20590,#20591,#20592,
#20593,#20594,#20595,#20596,#20597,#20598,#20599,#20600,#20601,#20602,#20603,
#20604,#20605,#20606,#20607,#20608,#20609,#20610,#20611,#20612,#20613,#20614,
#20615,#20616,#20617,#20618,#20619,#20620,#20621,#20622,#20623,#20624,#20625,
#20626,#20627,#20628,#20629,#20630,#20631,#20632,#20633,#20634,#20635,#20636,
#20637,#20638,#20639,#20640,#20641,#20642,#20643,#20644,#20645,#20646,#20647,
#20648,#20649,#20650,#20651,#20652,#20653,#20654,#20655,#20656,#20657,#20658,
#20659,#20660,#20661,#20662,#20663,#20664,#20665,#20666,#20667,#20668,#20669,
#20670,#20671,#20672,#20673,#20674,#20675,#20676,#20677,#20678,#20679,#20680,
#20681,#20682,#20683,#20684,#20685,#20686,#20687,#20688,#20689,#20690,#20691,
#20692,#20693,#20694,#20695,#20696,#20697,#20698,#20699,#20700,#20701,#20702,
#20703,#20704,#20705,#20706,#20707,#20708,#20709,#20710,#20711,#20712,#20713,
#20714,#20715,#20716,#20717,#20718,#20719,#20720,#20721,#20722,#20723,#20724,
#20725,#20726,#20727),.UNSPECIFIED.,.F.,.F.,(4,2,2,2,2,2,2,2,2,2,2,2,2,
2,2,2,2,2,2,2,2,2,2,2,2,2,2,2,2,2,2,2,2,2,2,2,2,2,2,2,2,2,2,2,2,2,2,2,2,
2,2,2,2,2,2,2,2,2,2,2,2,2,2,2,2,2,2,2,2,2,2,2,2,2,2,2,2,2,2,2,4),(-3.60242287809638,
-3.56721784695233,-3.55156189813843,-3.54087604581589,-3.52998929297132,
-3.51323412204218,-3.44497013969903,-3.39791346110271,-3.38735473125302,
-3.38105987829509,-3.37480333375927,-3.36442970316565,-3.30125673265392,
-3.26400908284791,-3.2460223081981,-3.23059678410155,-3.21995088869975,
-3.20900998526235,-3.19196872439598,-3.12667495572608,-3.07633231876972,
-3.06624290939729,-3.060044392539,-3.05368405300464,-3.04281000897509,-2.98411981411094,
-2.92597258491712,-2.91024653188731,-2.89954788321163,-2.88867582073824,
-2.87200116277746,-2.79526113514378,-2.7676005695254,-2.75528520035583,
-2.74536024613777,-2.73919461687122,-2.73279268291657,-2.72171705169384,
-2.66617790190046,-2.6045148723875,-2.58911903845016,-2.5784782235403,-2.56752998187024,
-2.55045013455705,-2.4856433040347,-2.43459781081709,-2.42465866485077,
-2.4184902403953,-2.41209205800306,-2.40103454940899,-2.34495831573944,
-2.2838783420997,-2.26844777215121,-2.25780098835939,-2.24686128134125,
-2.22982643444661,-2.15269523980569,-2.11311651180288,-2.1035514946851,
-2.09745561068995,-2.09095128173895,-2.07937494247329,-2.03104486686402,
-1.96667113596343,-1.94956534772693,-1.93861223520825,-1.92797478084316,
-1.9125987156333,-1.84933732086722,-1.79562684674695,-1.78435791261974,
-1.77791627132938,-1.77177925894983,-1.76200059891485,-1.71521190961271,
-1.64467016553331,-1.62818656919652,-1.6173497828642,-1.60662021642605,
-1.59072325636642,-1.57270504429441),.UNSPECIFIED.);
#1426=B_SPLINE_CURVE_WITH_KNOTS('',3,(#20728,#20729,#20730,#20731,#20732,
#20733,#20734,#20735,#20736,#20737,#20738,#20739,#20740,#20741,#20742,#20743,
#20744,#20745,#20746,#20747,#20748,#20749,#20750,#20751,#20752,#20753,#20754,
#20755,#20756,#20757,#20758,#20759,#20760,#20761,#20762,#20763,#20764,#20765,
#20766,#20767,#20768,#20769,#20770,#20771,#20772,#20773,#20774,#20775,#20776,
#20777,#20778,#20779,#20780,#20781,#20782,#20783,#20784,#20785,#20786,#20787,
#20788,#20789,#20790,#20791,#20792,#20793,#20794,#20795,#20796,#20797,#20798,
#20799,#20800,#20801,#20802,#20803,#20804,#20805,#20806,#20807,#20808,#20809,
#20810,#20811,#20812,#20813,#20814,#20815,#20816,#20817,#20818,#20819,#20820,
#20821,#20822,#20823,#20824,#20825,#20826,#20827,#20828,#20829,#20830,#20831,
#20832,#20833,#20834,#20835,#20836,#20837,#20838,#20839,#20840,#20841,#20842,
#20843,#20844,#20845,#20846,#20847,#20848,#20849,#20850,#20851,#20852,#20853,
#20854,#20855,#20856,#20857,#20858,#20859,#20860,#20861,#20862,#20863,#20864,
#20865,#20866,#20867,#20868,#20869,#20870,#20871,#20872,#20873,#20874,#20875,
#20876,#20877,#20878,#20879,#20880,#20881,#20882,#20883,#20884,#20885,#20886,
#20887,#20888,#20889,#20890,#20891,#20892,#20893),.UNSPECIFIED.,.F.,.F.,
(4,2,2,2,2,2,2,2,2,2,2,2,2,2,2,2,2,2,2,2,2,2,2,2,2,2,2,2,2,2,2,2,2,2,2,
2,2,2,2,2,2,2,2,2,2,2,2,2,2,2,2,2,2,2,2,2,2,2,2,2,2,2,2,2,2,2,2,2,2,2,2,
2,2,2,2,2,2,2,2,2,2,2,4),(-2.48879418648611,-2.482870786226,-2.42692956343107,
-2.36600785850896,-2.35045675318813,-2.33978959585287,-2.33016094885262,
-2.31444582835103,-2.23821710940245,-2.19523975059826,-2.1855542992085,
-2.17943580816656,-2.17296831262753,-2.16157124617673,-2.11118827433854,
-2.06704068844034,-2.04734877497841,-2.0308590398503,-2.02002175028717,
-2.00929425375571,-1.99340524118733,-1.97468006647316,-1.93457908581669,
-1.87709109853615,-1.86610750722511,-1.85972480069881,-1.85354479225751,
-1.84354696670865,-1.79297932372389,-1.72782025145022,-1.71077564213425,
-1.69983433429665,-1.6891891139229,-1.67376662544518,-1.65578255957856,
-1.61854770167534,-1.55527893663139,-1.54491074496027,-1.53865537392209,
-1.53235915546231,-1.52179434822374,-1.47368194101312,-1.40684450290551,
-1.38994962777,-1.37903651957945,-1.36837058921596,-1.3528291953071,-1.29288180784992,
-1.2357731213652,-1.2247627523323,-1.21837436650977,-1.21219837856251,-1.20222149130216,
-1.18982109384957,-1.16183326387008,-1.08267697612122,-1.06740015276224,
-1.05688543352747,-1.0459323793008,-1.02882628372556,-0.978950224072073,
-0.917329280997904,-0.905017534155332,-0.898365664895021,-0.892347412696423,
-0.883212145366521,-0.851369147050279,-0.8063673714056,-0.761177170046655,
-0.74626846473054,-0.735813488995268,-0.724759123042586,-0.707123289176841,
-0.685531949518534,-0.632133201827475,-0.591798795701873,-0.582163133943164,
-0.576655828465875,-0.570375876223591,-0.559890990576539,-0.546636681512379,
-0.51524224622991,-0.45931701754657),.UNSPECIFIED.);
#1427=B_SPLINE_CURVE_WITH_KNOTS('',3,(#20899,#20900,#20901,#20902,#20903,
#20904,#20905,#20906,#20907,#20908,#20909,#20910,#20911,#20912,#20913,#20914,
#20915,#20916,#20917,#20918,#20919,#20920,#20921,#20922,#20923,#20924,#20925,
#20926,#20927,#20928,#20929,#20930,#20931,#20932,#20933,#20934,#20935,#20936,
#20937,#20938,#20939,#20940,#20941,#20942,#20943,#20944,#20945,#20946,#20947,
#20948,#20949,#20950,#20951,#20952,#20953,#20954,#20955,#20956,#20957,#20958,
#20959,#20960,#20961,#20962,#20963,#20964,#20965,#20966,#20967,#20968,#20969,
#20970,#20971,#20972,#20973,#20974,#20975,#20976,#20977,#20978,#20979,#20980,
#20981,#20982,#20983,#20984,#20985,#20986,#20987,#20988,#20989,#20990,#20991,
#20992,#20993,#20994,#20995,#20996,#20997,#20998,#20999,#21000,#21001,#21002,
#21003,#21004,#21005,#21006,#21007,#21008,#21009,#21010,#21011,#21012,#21013,
#21014,#21015,#21016,#21017,#21018,#21019,#21020,#21021,#21022,#21023,#21024),
 .UNSPECIFIED.,.F.,.F.,(4,2,2,2,2,2,2,2,2,2,2,2,2,2,2,2,2,2,2,2,2,2,2,2,
2,2,2,2,2,2,2,2,2,2,2,2,2,2,2,2,2,2,2,2,2,2,2,2,2,2,2,2,2,2,2,2,2,2,2,2,
2,2,4),(-1.57273988019061,-1.56691346024312,-1.56072898385932,-1.55070573887629,
-1.50842406317083,-1.43222502173132,-1.41651494897745,-1.4068881047619,
-1.39622185106329,-1.38067029519754,-1.31828553824896,-1.26392823496632,
-1.25275991015442,-1.24633978848889,-1.24018924744267,-1.23033879598207,
-1.1760008817155,-1.11477371714702,-1.09750587349208,-1.08652241989586,
-1.07590625961537,-1.06065247806019,-1.00441058913554,-0.941945479199864,
-0.931484916050102,-0.925210316360724,-0.918933749330253,-0.90846320995488,
-0.895232867586938,-0.863935841053784,-0.792164412777069,-0.775839821530913,
-0.765033207159675,-0.754278155395765,-0.738235749766936,-0.682680727504737,
-0.621535654361532,-0.610922418914989,-0.604616329925545,-0.598370659077198,
-0.588049362231943,-0.575071819605588,-0.544810450900195,-0.470830069515804,
-0.454802593626465,-0.445123229273891,-0.434506544974243,-0.419248850028895,
-0.362877812031364,-0.300576688829507,-0.290096385595649,-0.283817819462706,
-0.277545348773213,-0.26709499646107,-0.253899067128589,-0.222745178504822,
-0.150669428219029,-0.134383624062453,-0.123583848906434,-0.112821487766765,
-0.0967404810140852,-0.0777076763684024,-0.000936417546807567),
 .UNSPECIFIED.);
#1428=B_SPLINE_CURVE_WITH_KNOTS('',3,(#21025,#21026,#21027,#21028,#21029,
#21030,#21031,#21032,#21033,#21034,#21035,#21036,#21037,#21038,#21039,#21040,
#21041,#21042,#21043,#21044,#21045,#21046,#21047,#21048,#21049,#21050,#21051,
#21052,#21053,#21054,#21055,#21056,#21057,#21058,#21059,#21060,#21061,#21062,
#21063,#21064,#21065,#21066),.UNSPECIFIED.,.F.,.F.,(4,2,2,2,2,2,2,2,2,2,
2,2,2,2,2,2,2,2,2,2,4),(-4.06024511832612,-4.04416917649443,-4.03341342658371,
-4.02723973391658,-4.02172518011229,-4.01522137623075,-4.00364660759717,
-3.94883815801512,-3.88741519438322,-3.87198632035072,-3.86134018065844,
-3.85040070853188,-3.83336531020972,-3.76801068386381,-3.71745087900611,
-3.70750155272622,-3.70133131022163,-3.69493621368035,-3.68389271615082,
-3.62747426988344,-3.60242287809638),.UNSPECIFIED.);
#1429=B_SPLINE_CURVE_WITH_KNOTS('',3,(#21068,#21069,#21070,#21071,#21072,
#21073,#21074,#21075,#21076,#21077,#21078,#21079,#21080,#21081,#21082,#21083,
#21084,#21085,#21086,#21087,#21088,#21089,#21090,#21091,#21092,#21093,#21094,
#21095,#21096,#21097,#21098,#21099,#21100,#21101,#21102,#21103,#21104,#21105,
#21106,#21107),.UNSPECIFIED.,.F.,.F.,(4,2,2,2,2,2,2,2,2,2,2,2,2,2,2,2,2,
2,2,4),(-0.45931701754657,-0.443662955116037,-0.427311208082828,-0.416498713796264,
-0.405746798310332,-0.389726540866301,-0.331854426135855,-0.273525442235887,
-0.262610494918398,-0.256241478612075,-0.250049205834386,-0.239992621745995,
-0.227459807822531,-0.198962724177927,-0.121968714348891,-0.106068905204749,
-0.0964095104727434,-0.0857712360881861,-0.0703931358704458,-0.000931723441433497),
 .UNSPECIFIED.);
#1430=B_SPLINE_CURVE_WITH_KNOTS('',3,(#21108,#21109,#21110,#21111,#21112,
#21113,#21114,#21115,#21116,#21117,#21118,#21119,#21120,#21121,#21122,#21123,
#21124,#21125,#21126,#21127,#21128,#21129,#21130,#21131,#21132,#21133,#21134,
#21135,#21136,#21137,#21138,#21139,#21140,#21141,#21142,#21143,#21144,#21145,
#21146,#21147,#21148,#21149,#21150,#21151,#21152,#21153,#21154,#21155,#21156,
#21157,#21158,#21159,#21160,#21161,#21162,#21163,#21164,#21165,#21166,#21167,
#21168,#21169,#21170,#21171,#21172,#21173,#21174,#21175,#21176,#21177,#21178,
#21179,#21180,#21181,#21182,#21183,#21184,#21185,#21186,#21187,#21188,#21189,
#21190,#21191,#21192,#21193,#21194,#21195,#21196,#21197,#21198,#21199,#21200,
#21201,#21202,#21203,#21204,#21205,#21206,#21207,#21208,#21209,#21210,#21211,
#21212,#21213,#21214,#21215,#21216,#21217,#21218,#21219,#21220,#21221,#21222,
#21223,#21224,#21225,#21226,#21227,#21228,#21229,#21230,#21231,#21232,#21233,
#21234,#21235,#21236,#21237,#21238,#21239,#21240,#21241,#21242,#21243,#21244,
#21245,#21246,#21247,#21248,#21249,#21250,#21251,#21252,#21253,#21254,#21255,
#21256,#21257,#21258,#21259,#21260,#21261,#21262,#21263,#21264,#21265,#21266,
#21267,#21268,#21269,#21270),.UNSPECIFIED.,.F.,.F.,(4,3,3,3,3,3,3,3,3,3,
3,3,3,3,3,3,3,3,3,3,3,3,3,3,3,3,3,3,3,3,3,3,3,3,3,3,3,3,3,3,3,3,3,3,3,3,
3,3,3,3,3,3,3,3,4),(-59.6902604182061,-59.5594237704194,-59.4859550544703,
-59.3928003674027,-59.2997701461022,-59.2068368787636,-59.1139699001593,
-59.0211370084654,-58.9283134841204,-58.83547462196,-58.7425375299053,-58.6495479743784,
-58.5564074989373,-58.4931583779947,-58.4000037272726,-58.3069735423544,
-58.2140403113874,-58.1211733689893,-58.0283405133873,-57.9355170249773,
-57.842678198552,-57.7497411417073,-57.6567516211492,-57.563611179937,-57.5003617015191,
-57.4072070142344,-57.3141767929645,-57.2212435259009,-57.1283765479317,
-57.0355436570937,-56.9427201338232,-56.8498812729533,-56.7569441825103,
-56.663954628777,-56.5708141554015,-56.5075650250435,-56.4144102728466,
-56.3213799860577,-56.2284466529631,-56.1355796084747,-56.0427466508417,
-55.9499230605827,-55.8570841326131,-55.7641469753148,-55.6711573547634,
-55.5780168153083,-55.514768348568,-55.4216338866632,-55.3286149917671,
-55.2356867536879,-55.1428243459392,-55.0499907232509,-54.957173946929,
-54.8643241540367,-54.8255493545477),.UNSPECIFIED.);
#1431=B_SPLINE_CURVE_WITH_KNOTS('',3,(#21275,#21276,#21277,#21278,#21279,
#21280,#21281,#21282,#21283,#21284,#21285,#21286,#21287,#21288,#21289,#21290,
#21291,#21292,#21293,#21294,#21295,#21296,#21297,#21298,#21299,#21300,#21301,
#21302,#21303,#21304,#21305,#21306,#21307,#21308,#21309,#21310,#21311,#21312,
#21313,#21314,#21315,#21316,#21317,#21318,#21319,#21320,#21321,#21322,#21323,
#21324,#21325,#21326,#21327,#21328,#21329,#21330,#21331,#21332,#21333,#21334,
#21335,#21336,#21337,#21338,#21339,#21340,#21341,#21342,#21343,#21344,#21345,
#21346,#21347,#21348,#21349,#21350,#21351,#21352,#21353,#21354,#21355,#21356,
#21357,#21358,#21359,#21360,#21361,#21362,#21363,#21364,#21365,#21366,#21367,
#21368,#21369,#21370,#21371,#21372,#21373,#21374,#21375,#21376,#21377,#21378,
#21379,#21380,#21381,#21382,#21383,#21384,#21385,#21386,#21387,#21388,#21389,
#21390,#21391,#21392,#21393,#21394,#21395,#21396,#21397,#21398,#21399,#21400,
#21401,#21402,#21403,#21404,#21405,#21406,#21407,#21408,#21409,#21410,#21411,
#21412,#21413,#21414,#21415,#21416,#21417,#21418,#21419,#21420,#21421,#21422,
#21423,#21424,#21425,#21426,#21427,#21428,#21429,#21430,#21431,#21432,#21433,
#21434,#21435,#21436),.UNSPECIFIED.,.F.,.F.,(4,2,2,2,2,2,2,2,2,2,2,2,2,
2,2,2,2,2,2,2,2,2,2,2,2,2,2,2,2,2,2,2,2,2,2,2,2,2,2,2,2,2,2,2,2,2,2,2,2,
2,2,2,2,2,2,2,2,2,2,2,2,2,2,2,2,2,2,2,2,2,2,2,2,2,2,2,2,2,2,2,4),(-3.60215374024631,
-3.55832024003365,-3.50705427008981,-3.4968341398854,-3.49059980699694,
-3.48507404412005,-3.47524953380503,-3.42545216512038,-3.36226836082976,
-3.34368290842291,-3.33249220157644,-3.32208238891058,-3.30781403324334,
-3.27108441733982,-3.21701855398476,-3.18394106025523,-3.17475410044726,
-3.16875045340127,-3.16214969449917,-3.15009518988101,-3.088210951477,-3.03819078612893,
-3.02105122816739,-3.01007851977686,-2.99954428438166,-2.9842337455252,
-2.90556246335392,-2.877528358283,-2.86511103438098,-2.85512072802792,-2.84893056883329,
-2.84252743093647,-2.83146332856961,-2.77555745219184,-2.71436471944647,
-2.69894454545784,-2.68829726882711,-2.67735044329871,-2.66028994445742,
-2.59511047468227,-2.54430720742812,-2.53437679428667,-2.52821091969801,
-2.52181660033448,-2.5107625946858,-2.45471757638087,-2.39362961337755,
-2.37820211010528,-2.36756281426864,-2.35663583530306,-2.33963333278813,
-2.27391475522454,-2.22361545056843,-2.21367491641689,-2.20750981472791,
-2.20111571714163,-2.19007639515179,-2.12142788152226,-2.08815716591305,
-2.06435557855792,-2.05216201634104,-2.04288922286891,-2.03065362175129,
-2.00660710569097,-1.97279945159265,-1.90547789764357,-1.89420888679343,
-1.88776616735981,-1.88162833803431,-1.87184546381257,-1.82478818754195,
-1.7546494918005,-1.73812119283216,-1.72727711461282,-1.71655653511475,
-1.70070403385726,-1.6820371535432,-1.64216857823805,-1.58423694395074,
-1.57328848970991,-1.57273988019061),.UNSPECIFIED.);
#1432=B_SPLINE_CURVE_WITH_KNOTS('',3,(#21438,#21439,#21440,#21441,#21442,
#21443,#21444,#21445,#21446,#21447,#21448,#21449,#21450,#21451,#21452,#21453,
#21454,#21455,#21456,#21457,#21458,#21459,#21460,#21461,#21462,#21463,#21464,
#21465,#21466,#21467,#21468,#21469,#21470,#21471,#21472,#21473,#21474,#21475,
#21476,#21477,#21478,#21479,#21480,#21481,#21482,#21483,#21484,#21485,#21486),
 .UNSPECIFIED.,.F.,.F.,(4,3,3,3,3,3,3,3,3,3,3,3,3,3,3,3,4),(-54.8255493545477,
-54.7325933049784,-54.6395755236503,-54.5464177867358,-54.5219716720924,
-54.4288168396936,-54.3357864745466,-54.2428530650123,-54.1499859472367,
-54.0571529182782,-53.9643292587279,-53.8714902635756,-53.7785530427219,
-53.6855633605477,-53.5924227631797,-53.5291749956168,-53.4070751110265),
 .UNSPECIFIED.);
#1433=B_SPLINE_CURVE_WITH_KNOTS('',3,(#21487,#21488,#21489,#21490,#21491,
#21492,#21493,#21494,#21495,#21496,#21497,#21498,#21499,#21500,#21501,#21502,
#21503,#21504,#21505,#21506,#21507,#21508,#21509,#21510,#21511,#21512,#21513,
#21514,#21515,#21516,#21517,#21518,#21519,#21520,#21521,#21522,#21523,#21524,
#21525,#21526,#21527,#21528,#21529,#21530,#21531,#21532,#21533,#21534,#21535,
#21536,#21537,#21538,#21539,#21540,#21541,#21542,#21543,#21544,#21545,#21546,
#21547,#21548,#21549,#21550,#21551,#21552,#21553,#21554,#21555,#21556,#21557,
#21558,#21559,#21560,#21561,#21562,#21563,#21564,#21565,#21566,#21567,#21568,
#21569,#21570,#21571,#21572,#21573,#21574,#21575,#21576,#21577,#21578,#21579,
#21580,#21581,#21582,#21583,#21584,#21585,#21586,#21587,#21588,#21589,#21590,
#21591,#21592,#21593,#21594,#21595,#21596,#21597,#21598,#21599,#21600,#21601,
#21602,#21603,#21604,#21605,#21606,#21607,#21608,#21609,#21610,#21611,#21612,
#21613,#21614,#21615,#21616),.UNSPECIFIED.,.F.,.F.,(4,2,2,2,2,2,2,2,2,2,
2,2,2,2,2,2,2,2,2,2,2,2,2,2,2,2,2,2,2,2,2,2,2,2,2,2,2,2,2,2,2,2,2,2,2,2,
2,2,2,2,2,2,2,2,2,2,2,2,2,2,2,2,2,2,4),(1.57246993836349,1.57255871975661,
1.57912898874073,1.58518286264246,1.59453433753174,1.62982177800544,1.6838845987573,
1.71828614481204,1.73092565126013,1.74139304571477,1.75240101115234,1.76982543540094,
1.82223034169457,1.88375253025013,1.89431647517552,1.90060935312462,1.90686298322144,
1.9172215182081,1.93026301994996,1.96077944471626,2.03428548587652,2.05039027237552,
2.06008452998516,2.07069376960653,2.08589349044519,2.14045811894018,2.20324430260467,
2.21444992277198,2.22088009460053,2.22702782231185,2.23685967261981,2.28727759474377,
2.35307275814114,2.37006985100011,2.38100242008193,2.3916543689042,2.40711469823814,
2.4251562826882,2.4626094056295,2.52535635003071,2.53577911681293,2.54204558594937,
2.54832907345374,2.5588350906938,2.5721275374578,2.60368083522067,2.6749914601101,
2.69138269714049,2.70220098702464,2.71294337437566,2.72891972722895,2.78831623300196,
2.84490980446916,2.85594447347385,2.86233734383786,2.86850877892949,2.8784642278196,
2.92941239254775,2.99428247378257,3.01135593775882,3.0223027976203,3.03294423964134,
3.04834472225774,3.1101328671186,3.14415938148886),.UNSPECIFIED.);
#1434=B_SPLINE_CURVE_WITH_KNOTS('',3,(#21620,#21621,#21622,#21623,#21624,
#21625,#21626,#21627,#21628,#21629,#21630,#21631,#21632,#21633,#21634,#21635,
#21636,#21637,#21638,#21639,#21640,#21641,#21642,#21643,#21644,#21645,#21646,
#21647,#21648,#21649,#21650,#21651,#21652,#21653,#21654,#21655,#21656),
 .UNSPECIFIED.,.F.,.F.,(4,3,3,3,3,3,3,3,3,3,3,3,4),(102.721401181859,102.870662929443,
102.958378318029,103.045982635166,103.133500549336,103.220958859954,103.308386983301,
103.395807072386,103.483241269198,103.570759547802,103.658325393878,103.746016067803,
103.787441035706),.UNSPECIFIED.);
#1435=B_SPLINE_CURVE_WITH_KNOTS('',3,(#21662,#21663,#21664,#21665,#21666,
#21667,#21668,#21669,#21670,#21671),.UNSPECIFIED.,.F.,.F.,(4,1,1,1,1,1,
1,4),(-105.704105011142,-104.856256282395,-103.863459605919,-102.870662929443,
-101.877866252968,-100.885069576492,-99.8922729000164,-99.4209215138263),
 .UNSPECIFIED.);
#1436=B_SPLINE_CURVE_WITH_KNOTS('',3,(#21673,#21674,#21675,#21676,#21677,
#21678,#21679,#21680,#21681,#21682,#21683,#21684,#21685,#21686,#21687,#21688,
#21689,#21690,#21691,#21692,#21693,#21694,#21695,#21696,#21697,#21698,#21699,
#21700,#21701,#21702,#21703,#21704,#21705,#21706,#21707,#21708,#21709,#21710,
#21711,#21712,#21713,#21714,#21715,#21716,#21717,#21718,#21719,#21720,#21721,
#21722,#21723,#21724,#21725,#21726,#21727,#21728,#21729,#21730,#21731,#21732,
#21733,#21734,#21735,#21736,#21737,#21738,#21739,#21740,#21741,#21742,#21743,
#21744,#21745,#21746,#21747,#21748,#21749,#21750,#21751,#21752,#21753,#21754,
#21755,#21756,#21757,#21758,#21759,#21760,#21761,#21762,#21763,#21764,#21765,
#21766,#21767,#21768,#21769,#21770,#21771,#21772,#21773,#21774,#21775,#21776,
#21777,#21778,#21779,#21780,#21781,#21782,#21783,#21784,#21785,#21786,#21787,
#21788,#21789,#21790,#21791,#21792,#21793,#21794,#21795,#21796,#21797,#21798,
#21799,#21800,#21801,#21802,#21803,#21804,#21805,#21806,#21807,#21808,#21809,
#21810,#21811,#21812,#21813,#21814,#21815,#21816,#21817,#21818,#21819,#21820,
#21821,#21822,#21823,#21824,#21825,#21826,#21827,#21828,#21829,#21830,#21831,
#21832,#21833,#21834,#21835,#21836,#21837,#21838,#21839,#21840,#21841,#21842,
#21843,#21844,#21845,#21846,#21847,#21848,#21849,#21850,#21851,#21852,#21853,
#21854,#21855,#21856,#21857,#21858,#21859,#21860,#21861,#21862,#21863,#21864,
#21865,#21866,#21867,#21868,#21869,#21870,#21871,#21872,#21873,#21874,#21875,
#21876,#21877,#21878,#21879,#21880,#21881,#21882,#21883,#21884,#21885,#21886,
#21887,#21888,#21889,#21890,#21891,#21892,#21893,#21894,#21895,#21896,#21897,
#21898),.UNSPECIFIED.,.F.,.F.,(4,3,3,3,3,3,3,3,3,3,3,3,3,3,3,3,3,3,3,3,
3,3,3,3,3,3,3,3,3,3,3,3,3,3,3,3,3,3,3,3,3,3,3,3,3,3,3,3,3,3,3,3,3,3,3,3,
3,3,3,3,3,3,3,3,3,3,3,3,3,3,3,3,3,3,3,4),(-99.4209197039621,-99.3293208753837,
-99.2376279663801,-99.1457470587024,-99.05376624967,-98.9615873900447,-98.8994762235407,
-98.8108583933232,-98.7223539962568,-98.6339393192582,-98.5430318477341,
-98.4547169969307,-98.3664149889373,-98.2781045317982,-98.1852482856149,
-98.0968062954329,-98.0083035049247,-97.9196751481056,-97.9066795470651,
-97.8180467295868,-97.7295271647582,-97.6410971592762,-97.5501953731904,
-97.4618648930757,-97.3735471711978,-97.2852209326452,-97.1923864171312,
-97.1039286208209,-97.0154100174652,-96.9267659333002,-96.9138828705894,
-96.825251508294,-96.7367333851373,-96.6483048060602,-96.5574024795669,
-96.4690733781967,-96.3807570148084,-96.2924321128727,-96.199595633183,
-96.1111391054233,-96.0226217469349,-95.9339788663736,-95.9210861941138,
-95.8324578037414,-95.74394270537,-95.6555171999199,-95.5646137396346,-95.476287813751,
-95.3879746582396,-95.2996529931624,-95.2068121242814,-95.1183588768868,
-95.0298448134196,-94.9412052289657,-94.9282895176381,-94.8396591330816,
-94.7511420149651,-94.662714466852,-94.5718117636408,-94.4834837512752,
-94.3951684966289,-94.3068447220381,-94.2140067518192,-94.125551388185,
-94.0370352064011,-93.9483935134071,-93.9354928411625,-93.8481338474163,
-93.7593339161101,-93.672189012311,-93.5850984288973,-93.498039699971,-93.40796337422,
-93.320869528771,-93.229301962869,-93.137734396967),.UNSPECIFIED.);
#1437=B_SPLINE_CURVE_WITH_KNOTS('',3,(#21900,#21901,#21902,#21903,#21904,
#21905,#21906,#21907,#21908,#21909,#21910,#21911,#21912,#21913,#21914,#21915,
#21916,#21917,#21918,#21919,#21920,#21921,#21922,#21923,#21924,#21925,#21926,
#21927,#21928,#21929,#21930,#21931,#21932,#21933,#21934,#21935,#21936,#21937,
#21938,#21939,#21940,#21941,#21942,#21943,#21944,#21945,#21946,#21947,#21948,
#21949,#21950,#21951,#21952,#21953,#21954,#21955,#21956,#21957,#21958,#21959,
#21960,#21961,#21962,#21963,#21964,#21965,#21966,#21967,#21968,#21969,#21970,
#21971,#21972,#21973,#21974,#21975,#21976,#21977,#21978,#21979,#21980,#21981,
#21982,#21983,#21984,#21985,#21986,#21987,#21988,#21989,#21990,#21991,#21992,
#21993,#21994,#21995,#21996,#21997,#21998,#21999,#22000,#22001,#22002,#22003,
#22004,#22005,#22006,#22007,#22008,#22009,#22010,#22011,#22012,#22013,#22014,
#22015,#22016,#22017,#22018,#22019,#22020,#22021,#22022,#22023,#22024,#22025,
#22026,#22027,#22028,#22029,#22030,#22031,#22032,#22033,#22034,#22035,#22036,
#22037,#22038,#22039,#22040,#22041,#22042,#22043,#22044,#22045,#22046,#22047,
#22048,#22049,#22050,#22051,#22052,#22053,#22054,#22055,#22056,#22057,#22058,
#22059,#22060,#22061,#22062,#22063,#22064,#22065,#22066,#22067,#22068,#22069,
#22070,#22071,#22072,#22073,#22074,#22075,#22076,#22077,#22078,#22079,#22080,
#22081,#22082,#22083,#22084,#22085,#22086,#22087,#22088,#22089,#22090,#22091,
#22092,#22093,#22094,#22095,#22096,#22097,#22098,#22099,#22100,#22101,#22102,
#22103,#22104,#22105,#22106,#22107,#22108,#22109,#22110,#22111,#22112,#22113,
#22114,#22115,#22116,#22117,#22118,#22119,#22120,#22121,#22122,#22123,#22124,
#22125),.UNSPECIFIED.,.F.,.F.,(4,3,3,3,3,3,3,3,3,3,3,3,3,3,3,3,3,3,3,3,
3,3,3,3,3,3,3,3,3,3,3,3,3,3,3,3,3,3,3,3,3,3,3,3,3,3,3,3,3,3,3,3,3,3,3,3,
3,3,3,3,3,3,3,3,3,3,3,3,3,3,3,3,3,3,3,4),(-93.1377343967825,-93.0103943584027,
-92.9426961646869,-92.8540664377197,-92.7655499839449,-92.6771231060632,
-92.5862201538317,-92.4978928219952,-92.4095782505129,-92.321255160973,
-92.2284162427826,-92.1399615626117,-92.0514460636615,-91.9628050484979,
-91.9498994882112,-91.8612695033504,-91.772752788195,-91.6843256457884,
-91.5934227915318,-91.5050951890547,-91.4167803451294,-91.3284569816384,
-91.2356184391627,-91.1471634837603,-91.0586477091683,-90.9700064194352,
-90.9571028117356,-90.8684728896893,-90.7799562377415,-90.6915291588546,
-90.6006262809053,-90.5122987423081,-90.4239839622835,-90.335660662643,
-90.2428220307972,-90.1543671385224,-90.0658514268007,-89.9772101991928,
-89.9643061352599,-89.8756762436412,-89.7871596227823,-89.698732575604,
-89.6078296860015,-89.5195021804533,-89.4311874339195,-89.3428641681764,
-89.2500254908284,-89.1615706331691,-89.0730549563071,-88.9844137636974,
-88.9715094587843,-88.8828795346996,-88.7943628809135,-88.7059358003901,
-88.6150329231299,-88.5267053834115,-88.4383906024603,-88.3500673020895,
-88.2572286721443,-88.1687737796457,-88.0802580678753,-87.9916168404687,
-87.9787127823086,-87.890082868362,-87.8015662248006,-87.7131391545749,
-87.6222362734821,-87.5339087441764,-87.4455939736623,-87.3572706837416,
-87.2644320392645,-87.1759771571514,-87.087461455743,-86.9988202386023,
-86.985916105833,-86.8545490896029),.UNSPECIFIED.);
#1438=B_SPLINE_CURVE_WITH_KNOTS('',3,(#22127,#22128,#22129,#22130,#22131,
#22132,#22133,#22134,#22135,#22136,#22137,#22138,#22139,#22140,#22141,#22142,
#22143,#22144,#22145,#22146,#22147,#22148,#22149,#22150,#22151,#22152,#22153,
#22154,#22155,#22156,#22157,#22158,#22159,#22160,#22161,#22162,#22163,#22164,
#22165,#22166,#22167,#22168,#22169,#22170,#22171,#22172,#22173,#22174,#22175,
#22176,#22177,#22178,#22179,#22180,#22181,#22182,#22183,#22184,#22185,#22186,
#22187,#22188,#22189,#22190,#22191,#22192,#22193,#22194,#22195,#22196,#22197,
#22198,#22199,#22200,#22201,#22202,#22203,#22204,#22205,#22206,#22207,#22208,
#22209,#22210,#22211,#22212,#22213,#22214,#22215,#22216,#22217,#22218,#22219,
#22220,#22221,#22222,#22223,#22224,#22225,#22226,#22227,#22228,#22229,#22230,
#22231,#22232,#22233,#22234,#22235,#22236,#22237,#22238,#22239,#22240,#22241,
#22242,#22243,#22244,#22245,#22246,#22247,#22248,#22249,#22250,#22251,#22252,
#22253,#22254,#22255,#22256,#22257,#22258,#22259,#22260,#22261,#22262,#22263,
#22264,#22265,#22266,#22267,#22268,#22269,#22270,#22271,#22272,#22273,#22274,
#22275,#22276,#22277,#22278,#22279,#22280,#22281,#22282,#22283,#22284,#22285,
#22286,#22287,#22288,#22289,#22290,#22291,#22292,#22293,#22294,#22295,#22296,
#22297,#22298,#22299,#22300,#22301,#22302,#22303,#22304,#22305,#22306,#22307,
#22308,#22309,#22310,#22311,#22312,#22313,#22314,#22315,#22316,#22317,#22318,
#22319,#22320,#22321,#22322,#22323,#22324,#22325,#22326,#22327,#22328,#22329,
#22330,#22331,#22332,#22333,#22334,#22335,#22336,#22337,#22338,#22339,#22340,
#22341,#22342,#22343,#22344,#22345,#22346,#22347,#22348,#22349,#22350,#22351,
#22352),.UNSPECIFIED.,.F.,.F.,(4,3,3,3,3,3,3,3,3,3,3,3,3,3,3,3,3,3,3,3,
3,3,3,3,3,3,3,3,3,3,3,3,3,3,3,3,3,3,3,3,3,3,3,3,3,3,3,3,3,3,3,3,3,3,3,3,
3,3,3,3,3,3,3,3,3,3,3,3,3,3,3,3,3,3,3,4),(-86.8545490893979,-86.7672499901414,
-86.6800454109648,-86.5929101898395,-86.5058118038681,-86.4187278319951,
-86.3316358695655,-86.2444597005961,-86.1572411555414,-86.0698827457749,
-85.9931194293573,-85.9044895140403,-85.8159728691177,-85.7275457975421,
-85.6366429169596,-85.5483153863403,-85.4600006145283,-85.3716773233271,
-85.2788386807158,-85.1903837973786,-85.1018680947656,-85.0132268764558,
-85.0003227528817,-84.9116928390893,-84.8231761957068,-84.7347491256843,
-84.6438462445245,-84.5555187154812,-84.4672039452513,-84.378880655636,
-84.2860420108285,-84.1975871290725,-84.1090714280394,-84.0204302112969,
-84.0075260764061,-83.9188961627797,-83.8303795195696,-83.7419524497257,
-83.6510495685013,-83.5627220396514,-83.4744072696198,-83.386083980208,
-83.2932453351386,-83.2047904535967,-83.1162747527811,-83.0276335362603,
-83.0147293999304,-82.926099485826,-82.8375828421303,-82.7491557717945,
-82.658252890752,-82.5699253613962,-82.4816105908546,-82.3932873009289,
-82.3004486565604,-82.2119937745,-82.1234780731646,-82.0348368561247,-82.0219327234548,
-81.9333028095752,-81.8447861661066,-81.7563590960003,-81.6654562148727,
-81.5771286857499,-81.4888139154421,-81.4004906257509,-81.307651981058,
-81.2191970992323,-81.1306813981307,-81.0420401813238,-81.0291360469791,
-80.9342373457995,-80.8396305779098,-80.7452006727478,-80.6510359595392,
-80.571363782615),.UNSPECIFIED.);
#1439=B_SPLINE_CURVE_WITH_KNOTS('',3,(#22354,#22355,#22356,#22357,#22358,
#22359,#22360,#22361,#22362,#22363,#22364,#22365,#22366,#22367,#22368,#22369,
#22370,#22371,#22372,#22373,#22374,#22375,#22376,#22377,#22378,#22379,#22380,
#22381,#22382,#22383,#22384,#22385,#22386,#22387,#22388,#22389,#22390,#22391,
#22392,#22393,#22394,#22395,#22396,#22397,#22398,#22399,#22400,#22401,#22402,
#22403,#22404,#22405,#22406,#22407,#22408,#22409,#22410,#22411,#22412,#22413,
#22414,#22415,#22416,#22417,#22418,#22419,#22420,#22421,#22422,#22423,#22424,
#22425,#22426,#22427,#22428,#22429,#22430,#22431,#22432,#22433,#22434,#22435,
#22436,#22437,#22438,#22439,#22440,#22441,#22442,#22443,#22444,#22445,#22446,
#22447,#22448,#22449,#22450,#22451,#22452,#22453,#22454,#22455,#22456,#22457,
#22458,#22459,#22460,#22461,#22462,#22463,#22464,#22465,#22466,#22467,#22468,
#22469,#22470,#22471,#22472,#22473,#22474,#22475,#22476,#22477,#22478,#22479,
#22480,#22481,#22482,#22483,#22484,#22485,#22486,#22487,#22488,#22489,#22490,
#22491,#22492,#22493,#22494,#22495,#22496,#22497,#22498,#22499,#22500,#22501,
#22502,#22503,#22504,#22505,#22506,#22507,#22508,#22509,#22510,#22511,#22512,
#22513,#22514,#22515,#22516,#22517,#22518,#22519,#22520,#22521,#22522,#22523,
#22524,#22525,#22526,#22527,#22528,#22529,#22530,#22531,#22532,#22533,#22534,
#22535,#22536,#22537,#22538,#22539,#22540,#22541,#22542,#22543,#22544,#22545,
#22546,#22547,#22548,#22549,#22550,#22551,#22552,#22553,#22554,#22555,#22556,
#22557,#22558,#22559,#22560,#22561,#22562,#22563,#22564,#22565,#22566,#22567,
#22568,#22569,#22570,#22571,#22572,#22573,#22574,#22575,#22576,#22577,#22578,
#22579),.UNSPECIFIED.,.F.,.F.,(4,3,3,3,3,3,3,3,3,3,3,3,3,3,3,3,3,3,3,3,
3,3,3,3,3,3,3,3,3,3,3,3,3,3,3,3,3,3,3,3,3,3,3,3,3,3,3,3,3,3,3,3,3,3,3,3,
3,3,3,3,3,3,3,3,3,3,3,3,3,3,3,3,3,3,3,4),(-80.5713637824232,-80.4802388382001,
-80.3890358883964,-80.2976607708068,-80.2061965706322,-80.1145367878468,
-80.0363393705035,-79.9477094565397,-79.8591928129868,-79.7707657427952,
-79.6798628616993,-79.5915353324914,-79.5032205620988,-79.414897272323,
-79.3220586277492,-79.23360374584,-79.1450880446554,-79.0564468277664,-79.0435426940279,
-78.9549127801537,-78.8663961366907,-78.7779690665895,-78.6870661854598,
-78.5987386563421,-78.5104238860394,-78.4221005963534,-78.3292619516531,
-78.2408070698319,-78.152291368735,-78.0636501519321,-78.0507460175522,
-77.9621161036702,-77.8735994601996,-77.7851723900913,-77.6942695089645,
-77.6059419798413,-77.5176272095339,-77.4293039198435,-77.3364652751518,
-77.2480103933277,-77.1594946922283,-77.0708534754237,-77.0579493410766,
-76.9693194269626,-76.8808027832593,-76.792375712917,-76.7014728318775,
-76.6131453025204,-76.5248305319791,-76.4365072420554,-76.3436685976918,
-76.2552137156379,-76.16669801431,-76.0780567972801,-76.0651526646009,-75.9765227510041,
-75.8880061078176,-75.7995790379919,-75.7086761567586,-75.6203486279128,
-75.5320338578802,-75.4437105684623,-75.350871923378,-75.2624170418168,
-75.1739013409774,-75.0852601244265,-75.0723559881253,-74.9849531892148,
-74.8976869217581,-74.8104984384445,-74.7233652466618,-74.6362649091503,
-74.5491421323337,-74.4620121544108,-74.3747943755378,-74.2881784754821),
 .UNSPECIFIED.);
#1440=B_SPLINE_CURVE_WITH_KNOTS('',3,(#22581,#22582,#22583,#22584,#22585,
#22586,#22587,#22588,#22589,#22590,#22591,#22592,#22593,#22594,#22595,#22596,
#22597,#22598,#22599,#22600,#22601,#22602,#22603,#22604,#22605,#22606,#22607,
#22608,#22609,#22610,#22611,#22612,#22613,#22614,#22615,#22616,#22617,#22618,
#22619,#22620,#22621,#22622,#22623,#22624,#22625,#22626,#22627,#22628,#22629,
#22630,#22631,#22632,#22633,#22634,#22635,#22636,#22637,#22638,#22639,#22640,
#22641,#22642,#22643,#22644,#22645,#22646,#22647,#22648,#22649,#22650,#22651,
#22652,#22653,#22654,#22655,#22656,#22657,#22658,#22659,#22660,#22661,#22662,
#22663,#22664,#22665,#22666,#22667,#22668,#22669,#22670,#22671,#22672,#22673,
#22674,#22675,#22676,#22677,#22678,#22679,#22680,#22681,#22682,#22683,#22684,
#22685,#22686,#22687,#22688,#22689,#22690,#22691,#22692,#22693,#22694,#22695,
#22696,#22697,#22698,#22699,#22700,#22701,#22702,#22703,#22704,#22705,#22706,
#22707,#22708,#22709,#22710,#22711,#22712,#22713,#22714,#22715,#22716,#22717,
#22718,#22719,#22720,#22721,#22722,#22723,#22724,#22725,#22726,#22727,#22728,
#22729,#22730,#22731,#22732,#22733,#22734,#22735,#22736,#22737,#22738,#22739,
#22740,#22741,#22742,#22743,#22744,#22745,#22746,#22747,#22748,#22749,#22750,
#22751,#22752,#22753,#22754,#22755,#22756,#22757,#22758,#22759,#22760,#22761,
#22762,#22763,#22764,#22765,#22766,#22767,#22768,#22769,#22770,#22771,#22772,
#22773,#22774,#22775,#22776,#22777,#22778,#22779,#22780,#22781,#22782,#22783,
#22784,#22785,#22786,#22787,#22788,#22789,#22790,#22791,#22792,#22793,#22794,
#22795,#22796,#22797,#22798,#22799,#22800,#22801,#22802,#22803,#22804,#22805,
#22806),.UNSPECIFIED.,.F.,.F.,(4,3,3,3,3,3,3,3,3,3,3,3,3,3,3,3,3,3,3,3,
3,3,3,3,3,3,3,3,3,3,3,3,3,3,3,3,3,3,3,3,3,3,3,3,3,3,3,3,3,3,3,3,3,3,3,3,
3,3,3,3,3,3,3,3,3,3,3,3,3,3,3,3,3,3,3,4),(-74.2881784752437,-74.1649193736331,
-74.0795593116496,-73.9909293962694,-73.9024127512956,-73.8139856796808,
-73.7230827991175,-73.6347552684894,-73.5464404966801,-73.4581172054929,
-73.3652785629132,-73.2768236796181,-73.188307977057,-73.0996667588124,
-73.086762635174,-72.9981327240733,-72.9096160833806,-72.8211890160432,
-72.7302861338751,-72.6419586074888,-72.5536438399008,-72.4653205529098,
-72.3724819043569,-72.2840270251565,-72.1955113266547,-72.106870112395,
-72.0939659586983,-72.0053360444867,-71.9168194007111,-71.8283923303221,
-71.7374894493097,-71.6491619199673,-71.5608471494635,-71.4725238596003,
-71.3796852152559,-71.291230333318,-71.2027146321253,-71.1140734152566,
-71.1011692822227,-71.0125393577712,-70.9240227036889,-70.8355956229393,
-70.7446927457903,-70.6563652060211,-70.5680504250841,-70.4797271247928,
-70.3868884950313,-70.2984336027753,-70.2099178913036,-70.1212766642732,
-70.108372605747,-70.0197427159813,-69.9312260966195,-69.8427990505834,
-69.7518961604194,-69.6635686551279,-69.5752539085218,-69.4869306423774,
-69.3940919641009,-69.3056371052161,-69.2171214268451,-69.1284802323341,
-69.1155759292714,-69.0269460046457,-68.9384293506142,-68.8500022701374,
-68.7590993929697,-68.6707718540151,-68.5824570740912,-68.4941337750091,
-68.4012951444558,-68.3128402538869,-68.224324544266,-68.1356833193045,
-68.1227792527958,-68.0049931680641),.UNSPECIFIED.);
#1441=B_SPLINE_CURVE_WITH_KNOTS('',3,(#22808,#22809,#22810,#22811,#22812,
#22813,#22814,#22815,#22816,#22817,#22818,#22819,#22820,#22821,#22822,#22823,
#22824,#22825,#22826,#22827,#22828,#22829,#22830,#22831,#22832,#22833,#22834,
#22835,#22836,#22837,#22838,#22839,#22840,#22841,#22842,#22843,#22844,#22845,
#22846,#22847,#22848,#22849,#22850,#22851,#22852,#22853,#22854,#22855,#22856,
#22857,#22858,#22859,#22860,#22861,#22862,#22863,#22864,#22865,#22866,#22867,
#22868,#22869,#22870,#22871,#22872,#22873,#22874,#22875,#22876,#22877,#22878,
#22879,#22880,#22881,#22882,#22883,#22884,#22885,#22886,#22887,#22888,#22889,
#22890,#22891,#22892,#22893,#22894,#22895,#22896,#22897,#22898,#22899,#22900,
#22901,#22902,#22903,#22904,#22905,#22906,#22907,#22908,#22909,#22910,#22911,
#22912,#22913,#22914,#22915,#22916,#22917,#22918,#22919,#22920,#22921,#22922,
#22923,#22924,#22925,#22926,#22927,#22928,#22929,#22930,#22931,#22932,#22933,
#22934,#22935,#22936,#22937,#22938,#22939,#22940,#22941,#22942,#22943,#22944,
#22945,#22946,#22947,#22948,#22949,#22950,#22951,#22952,#22953,#22954,#22955,
#22956,#22957,#22958,#22959,#22960,#22961,#22962,#22963,#22964,#22965,#22966,
#22967,#22968,#22969,#22970,#22971,#22972,#22973,#22974,#22975,#22976,#22977,
#22978,#22979,#22980,#22981,#22982,#22983,#22984,#22985,#22986,#22987,#22988,
#22989,#22990,#22991,#22992,#22993,#22994,#22995,#22996,#22997,#22998,#22999,
#23000,#23001,#23002,#23003,#23004,#23005,#23006,#23007,#23008,#23009,#23010,
#23011,#23012,#23013,#23014,#23015,#23016,#23017,#23018,#23019,#23020,#23021,
#23022,#23023,#23024,#23025,#23026,#23027,#23028,#23029,#23030,#23031,#23032,
#23033),.UNSPECIFIED.,.F.,.F.,(4,3,3,3,3,3,3,3,3,3,3,3,3,3,3,3,3,3,3,3,
3,3,3,3,3,3,3,3,3,3,3,3,3,3,3,3,3,3,3,3,3,3,3,3,3,3,3,3,3,3,3,3,3,3,3,3,
3,3,3,3,3,3,3,3,3,3,3,3,3,3,3,3,3,3,3,4),(-68.0049931678491,-67.9176272364039,
-67.8303590125715,-67.7428119580401,-67.6556573987918,-67.5685201374423,
-67.4813778063888,-67.3935289988716,-67.306263955284,-67.2181232658021,
-67.1299825763201,-67.0413528634227,-66.9528364210138,-66.8644095518054,
-66.7735065953103,-66.6851792654233,-66.5968646933924,-66.5085416008059,
-66.4157026755656,-66.3272479860896,-66.2387324756828,-66.150091446084,
-66.1371858998445,-66.0485558370061,-65.9600390458805,-65.8716118295741,
-65.7807090037984,-65.6923813329701,-65.6040664228603,-65.5157429954148,
-65.4229045524033,-65.3344495392061,-65.2459337089372,-65.1572923668465,
-65.1443892233688,-65.0557588345089,-64.9672417129162,-64.8788141621505,
-64.7879114602434,-64.6995834472815,-64.6112681928031,-64.5229444191439,
-64.4301064510812,-64.3416510902931,-64.2531349120133,-64.1644932234347,
-64.1515925468932,-64.0629642601545,-63.9744492455001,-63.8860238039323,
-63.7951203122429,-63.70679440072,-63.6184812411673,-63.5301595536508,-63.4373186328424,
-63.3488653169106,-63.2603511690565,-63.1717114782792,-63.1587958704175,
-63.0701642993288,-62.9816460075068,-62.8932172997264,-62.8023150365033,
-62.7139859062041,-62.6256695509626,-62.5373446942416,-62.4445083191667,
-62.3560519294957,-62.2675347410291,-62.1788920746855,-62.1659991939419,
-62.0703971982959,-61.9751094420689,-61.8800163865857,-61.7852175910644,
-61.7218081198968),.UNSPECIFIED.);
#1442=B_SPLINE_CURVE_WITH_KNOTS('',3,(#23035,#23036,#23037,#23038,#23039,
#23040,#23041,#23042,#23043,#23044),.UNSPECIFIED.,.F.,.F.,(4,1,1,1,1,1,
1,4),(-61.7218078608845,-61.1732025174663,-60.1804058409906,-59.187609164515,
-58.1948124880393,-57.2020158115637,-56.209219135088,-55.4386448475283),
 .UNSPECIFIED.);
#1443=B_SPLINE_CURVE_WITH_KNOTS('',3,(#23046,#23047,#23048,#23049,#23050,
#23051),.UNSPECIFIED.,.F.,.F.,(4,2,4),(0.00013759178667376,0.0288396991503689,
0.0579150026494099),.UNSPECIFIED.);
#1444=B_SPLINE_CURVE_WITH_KNOTS('',3,(#23055,#23056,#23057,#23058,#23059,
#23060,#23061,#23062,#23063),.UNSPECIFIED.,.F.,.F.,(4,1,1,1,1,1,4),(53.2308291056646,
54.2236257821402,55.2164224586157,56.2092191350913,57.2020158115669,58.1948124880425,
58.7391040316016),.UNSPECIFIED.);
#1445=B_SPLINE_CURVE_WITH_KNOTS('',3,(#23065,#23066,#23067,#23068,#23069,
#23070,#23071,#23072,#23073,#23074,#23075,#23076,#23077,#23078,#23079,#23080,
#23081,#23082,#23083,#23084,#23085,#23086,#23087,#23088,#23089,#23090,#23091,
#23092,#23093,#23094,#23095,#23096,#23097,#23098,#23099,#23100,#23101,#23102,
#23103,#23104,#23105,#23106,#23107,#23108,#23109,#23110,#23111,#23112,#23113,
#23114,#23115,#23116,#23117,#23118,#23119,#23120,#23121,#23122,#23123,#23124,
#23125,#23126,#23127,#23128,#23129,#23130,#23131,#23132,#23133,#23134,#23135,
#23136,#23137,#23138,#23139,#23140,#23141,#23142,#23143,#23144,#23145,#23146,
#23147,#23148,#23149,#23150,#23151,#23152,#23153,#23154,#23155,#23156,#23157,
#23158,#23159,#23160,#23161,#23162,#23163,#23164,#23165,#23166,#23167,#23168,
#23169,#23170,#23171,#23172,#23173,#23174,#23175,#23176,#23177,#23178,#23179,
#23180,#23181,#23182,#23183,#23184,#23185,#23186,#23187,#23188,#23189,#23190,
#23191,#23192,#23193,#23194,#23195,#23196,#23197,#23198,#23199,#23200,#23201,
#23202,#23203,#23204,#23205,#23206,#23207,#23208,#23209,#23210,#23211,#23212,
#23213,#23214,#23215,#23216,#23217,#23218,#23219,#23220,#23221,#23222,#23223,
#23224,#23225,#23226,#23227,#23228,#23229,#23230,#23231,#23232,#23233,#23234,
#23235,#23236,#23237,#23238,#23239,#23240,#23241,#23242,#23243,#23244,#23245,
#23246,#23247,#23248,#23249,#23250,#23251,#23252,#23253,#23254,#23255,#23256,
#23257,#23258,#23259,#23260,#23261,#23262,#23263,#23264,#23265,#23266,#23267,
#23268,#23269,#23270,#23271,#23272,#23273,#23274,#23275,#23276,#23277,#23278,
#23279,#23280,#23281,#23282,#23283,#23284,#23285,#23286,#23287,#23288,#23289,
#23290),.UNSPECIFIED.,.F.,.F.,(4,3,3,3,3,3,3,3,3,3,3,3,3,3,3,3,3,3,3,3,
3,3,3,3,3,3,3,3,3,3,3,3,3,3,3,3,3,3,3,3,3,3,3,3,3,3,3,3,3,3,3,3,3,3,3,3,
3,3,3,3,3,3,3,3,3,3,3,3,3,3,3,3,3,3,3,4),(58.7391042641703,58.8335838703561,
58.9284005420665,59.0233890466834,59.118661083167,59.1876091645181,59.2762538660009,
59.3647855821298,59.4532279897729,59.5441252211755,59.6324686487407,59.7207994986245,
59.8091390319831,59.9019557342358,59.9904271252048,60.0789594252534,60.167617269212,
60.1804058409936,60.2690236889587,60.3575281040159,60.445942799225,60.5368502640056,
60.6251651334518,60.7134671602168,60.8017776362361,60.8946338565443,60.9830758657094,
61.0715786752344,61.1602070510044,61.1732025174692,61.2618353276175,61.3503548850479,
61.4387848830728,61.5296866719318,61.6180171444911,61.7063348587903,61.7946610897492,
61.8874956157981,61.9759534045469,62.064472000353,62.1531160770312,62.1659991939448,
62.2546305549895,62.3431486768587,62.4315772546133,62.5224795815892,62.6108086815575,
62.6991250435169,62.7874499439978,62.8802864256034,62.9687429518561,63.0572603088198,
63.1459031878398,63.1587958704204,63.2474242637227,63.3359393650657,63.4243648735262,
63.5152683326974,63.6035942616666,63.6919074202865,63.7802290884916,63.8730699530927,
63.961523203636,64.0500372702589,64.1386768578591,64.1515925468959,64.23900867765,
64.3263123945337,64.4135197963484,64.500673816494,64.5877968757005,64.674911363053,
64.7620861803452,64.849289012654,64.9366137069396,65.0222893385667),
 .UNSPECIFIED.);
#1446=B_SPLINE_CURVE_WITH_KNOTS('',3,(#23292,#23293,#23294,#23295,#23296,
#23297,#23298,#23299,#23300,#23301,#23302,#23303,#23304,#23305,#23306,#23307,
#23308,#23309,#23310,#23311,#23312,#23313,#23314,#23315,#23316,#23317,#23318,
#23319,#23320,#23321,#23322,#23323,#23324,#23325,#23326,#23327,#23328,#23329,
#23330,#23331,#23332,#23333,#23334,#23335,#23336,#23337,#23338,#23339,#23340,
#23341,#23342,#23343,#23344,#23345,#23346,#23347,#23348,#23349,#23350,#23351,
#23352,#23353,#23354,#23355,#23356,#23357,#23358,#23359,#23360,#23361,#23362,
#23363,#23364,#23365,#23366,#23367,#23368,#23369,#23370,#23371,#23372,#23373,
#23374,#23375,#23376,#23377,#23378,#23379,#23380,#23381,#23382,#23383,#23384,
#23385,#23386,#23387,#23388,#23389,#23390,#23391,#23392,#23393,#23394,#23395,
#23396,#23397,#23398,#23399,#23400,#23401,#23402,#23403,#23404,#23405,#23406,
#23407,#23408,#23409,#23410,#23411,#23412,#23413,#23414,#23415,#23416,#23417,
#23418,#23419,#23420,#23421,#23422,#23423,#23424,#23425,#23426,#23427,#23428,
#23429,#23430,#23431,#23432,#23433,#23434,#23435,#23436,#23437,#23438,#23439,
#23440,#23441,#23442,#23443,#23444,#23445,#23446,#23447,#23448,#23449,#23450,
#23451,#23452,#23453,#23454,#23455,#23456,#23457,#23458,#23459,#23460,#23461,
#23462,#23463,#23464,#23465,#23466,#23467,#23468,#23469,#23470,#23471,#23472,
#23473,#23474,#23475,#23476,#23477,#23478,#23479,#23480,#23481,#23482,#23483,
#23484,#23485,#23486,#23487,#23488,#23489,#23490,#23491,#23492,#23493,#23494,
#23495,#23496,#23497,#23498,#23499,#23500,#23501,#23502,#23503,#23504,#23505,
#23506,#23507,#23508,#23509,#23510,#23511,#23512,#23513,#23514,#23515,#23516,
#23517),.UNSPECIFIED.,.F.,.F.,(4,3,3,3,3,3,3,3,3,3,3,3,3,3,3,3,3,3,3,3,
3,3,3,3,3,3,3,3,3,3,3,3,3,3,3,3,3,3,3,3,3,3,3,3,3,3,3,3,3,3,3,3,3,3,3,3,
3,3,3,3,3,3,3,3,3,3,3,3,3,3,3,3,3,3,3,4),(65.0222893387811,65.1443892233715,
65.2330192623953,65.3215360342572,65.4099632358317,65.5008660688337,65.5891937362466,
65.6775086471462,65.7658320795859,65.8586705346512,65.9471255633786,66.0356414128,
66.1242827790579,66.1371858998471,66.2258156272582,66.3143320814836,66.402758959822,
66.4936619118846,66.58198924419,66.670303816145,66.7586269061608,66.8514658237013,
66.9399205043519,67.028436003783,67.1170770194266,67.1299825763227,67.2186125609608,
67.3071292758913,67.3955564180708,67.4864592724117,67.5747868746579,67.6631017183513,
67.7514250816097,67.8442636244069,67.9327185795769,68.0212343539367,68.1098756434391,
68.1227792527983,68.2114091748451,68.2999258267928,68.3883529056791,68.4792557836284,
68.5675833222237,68.6558981022458,68.7442214018833,68.8370600337309,68.9255149260015,
69.0140306377185,69.1026718653213,69.1155759292738,69.2042058209554,69.2927224418782,
69.3811494891212,69.4720523786998,69.5603798843147,69.6486946309156,69.7370178967264,
69.8298565739821,69.9183114317098,70.0068271086403,70.0954683013184,70.1083726057494,
70.1970025297981,70.2855191835478,70.3739462640343,70.4648491413082,70.5531766809891,
70.6414914619027,70.7298147622357,70.822653392233,70.9111082846938,70.9996239964263,
71.0882652237953,71.101169282225,71.2256508576449,71.3054746459608),
 .UNSPECIFIED.);
#1447=B_SPLINE_CURVE_WITH_KNOTS('',3,(#23519,#23520,#23521,#23522,#23523,
#23524,#23525,#23526,#23527,#23528,#23529,#23530,#23531,#23532,#23533,#23534,
#23535,#23536,#23537,#23538,#23539,#23540,#23541,#23542,#23543,#23544,#23545,
#23546,#23547,#23548,#23549,#23550,#23551,#23552,#23553,#23554,#23555,#23556,
#23557,#23558,#23559,#23560,#23561,#23562,#23563,#23564,#23565,#23566,#23567,
#23568,#23569,#23570,#23571,#23572,#23573,#23574,#23575,#23576,#23577,#23578,
#23579,#23580,#23581,#23582,#23583,#23584,#23585,#23586,#23587,#23588,#23589,
#23590,#23591,#23592,#23593,#23594,#23595,#23596,#23597,#23598,#23599,#23600,
#23601,#23602,#23603,#23604,#23605,#23606,#23607,#23608,#23609,#23610,#23611,
#23612,#23613,#23614,#23615,#23616,#23617,#23618,#23619,#23620,#23621,#23622,
#23623,#23624,#23625,#23626,#23627,#23628,#23629,#23630,#23631,#23632,#23633,
#23634,#23635,#23636,#23637,#23638,#23639,#23640,#23641,#23642,#23643,#23644,
#23645,#23646,#23647,#23648,#23649,#23650,#23651,#23652,#23653,#23654,#23655,
#23656,#23657,#23658,#23659,#23660,#23661,#23662,#23663,#23664,#23665,#23666,
#23667,#23668,#23669,#23670,#23671,#23672,#23673,#23674,#23675,#23676,#23677,
#23678,#23679,#23680,#23681,#23682,#23683,#23684,#23685,#23686,#23687,#23688,
#23689,#23690,#23691,#23692,#23693,#23694,#23695,#23696,#23697,#23698,#23699,
#23700,#23701,#23702,#23703,#23704,#23705,#23706,#23707,#23708,#23709,#23710,
#23711,#23712,#23713,#23714,#23715,#23716,#23717,#23718,#23719,#23720,#23721,
#23722,#23723,#23724,#23725,#23726,#23727,#23728,#23729,#23730,#23731,#23732,
#23733,#23734,#23735,#23736,#23737,#23738,#23739,#23740,#23741,#23742,#23743,
#23744),.UNSPECIFIED.,.F.,.F.,(4,3,3,3,3,3,3,3,3,3,3,3,3,3,3,3,3,3,3,3,
3,3,3,3,3,3,3,3,3,3,3,3,3,3,3,3,3,3,3,3,3,3,3,3,3,3,3,3,3,3,3,3,3,3,3,3,
3,3,3,3,3,3,3,3,3,3,3,3,3,3,3,3,3,3,3,4),(71.3054746461005,71.3926937178224,
71.4803527479322,71.56745629258,71.654541925881,71.7416320525193,71.8297155290647,
71.9169275868896,72.0054467727951,72.0939659587006,72.1825958700471,72.27111251094,
72.3595395784323,72.4504424605253,72.5387699869533,72.6270847545411,72.7154080414897,
72.8082466899113,72.8967015689638,72.9852172672815,73.0738584813068,73.0867626351761,
73.1753925504875,73.2639091954045,73.3523362669747,73.4432391475593,73.5315666781729,
73.619881449979,73.7082047411741,73.8010433837935,73.8894982671248,73.9780139697316,
74.0666551880355,74.0795593116517,74.1681892254449,74.2567058688284,74.3451329388519,
74.4360358200113,74.5243633490555,74.6126781192865,74.7010014089025,74.7938400537087,
74.8822949354655,74.9708106365,75.0594518532432,75.0723559881273,75.1609859017548,
75.2495025449661,75.3379296148109,75.4288324960349,75.5171600248858,75.6054747949184,
75.6937980843313,75.7866367293992,75.8750916109423,75.9636073117593,76.0522485282809,
76.0651526646029,76.1537825787065,76.242299222401,76.330726292736,76.4216291737788,
76.5099567031338,76.5982714736746,76.6865947635996,76.7794334079693,76.8678882900288,
76.9564039913636,77.0450452084028,77.0579493410785,77.149780829808,77.2414655319119,
77.3329735006271,77.424377476035,77.5156633354471,77.5886599531404),
 .UNSPECIFIED.);
#1448=B_SPLINE_CURVE_WITH_KNOTS('',3,(#23746,#23747,#23748,#23749,#23750,
#23751,#23752,#23753,#23754,#23755,#23756,#23757,#23758,#23759,#23760,#23761,
#23762,#23763,#23764,#23765,#23766,#23767,#23768,#23769,#23770,#23771,#23772,
#23773,#23774,#23775,#23776,#23777,#23778,#23779,#23780,#23781,#23782,#23783,
#23784,#23785,#23786,#23787,#23788,#23789,#23790,#23791,#23792,#23793,#23794,
#23795,#23796,#23797,#23798,#23799,#23800,#23801,#23802,#23803,#23804,#23805,
#23806,#23807,#23808,#23809,#23810,#23811,#23812,#23813,#23814,#23815,#23816,
#23817,#23818,#23819,#23820,#23821,#23822,#23823,#23824,#23825,#23826,#23827,
#23828,#23829,#23830,#23831,#23832,#23833,#23834,#23835,#23836,#23837,#23838,
#23839,#23840,#23841,#23842,#23843,#23844,#23845,#23846,#23847,#23848,#23849,
#23850,#23851,#23852,#23853,#23854,#23855,#23856,#23857,#23858,#23859,#23860,
#23861,#23862,#23863,#23864,#23865,#23866,#23867,#23868,#23869,#23870,#23871,
#23872,#23873,#23874,#23875,#23876,#23877,#23878,#23879,#23880,#23881,#23882,
#23883,#23884,#23885,#23886,#23887,#23888,#23889,#23890,#23891,#23892,#23893,
#23894,#23895,#23896,#23897,#23898,#23899,#23900,#23901,#23902,#23903,#23904,
#23905,#23906,#23907,#23908,#23909,#23910,#23911,#23912,#23913,#23914,#23915,
#23916,#23917,#23918,#23919,#23920,#23921,#23922,#23923,#23924,#23925,#23926,
#23927,#23928,#23929,#23930,#23931,#23932,#23933,#23934,#23935,#23936,#23937,
#23938,#23939,#23940,#23941,#23942,#23943,#23944,#23945,#23946,#23947,#23948,
#23949,#23950,#23951,#23952,#23953,#23954,#23955,#23956,#23957,#23958,#23959,
#23960,#23961,#23962,#23963,#23964,#23965,#23966,#23967,#23968,#23969,#23970,
#23971),.UNSPECIFIED.,.F.,.F.,(4,3,3,3,3,3,3,3,3,3,3,3,3,3,3,3,3,3,3,3,
3,3,3,3,3,3,3,3,3,3,3,3,3,3,3,3,3,3,3,3,3,3,3,3,3,3,3,3,3,3,3,3,3,3,3,3,
3,3,3,3,3,3,3,3,3,3,3,3,3,3,3,3,3,3,3,4),(77.5886599533119,77.6825471555259,
77.7767398883194,77.8710860075021,77.9657069232752,78.050746017554,78.1393759314319,
78.227892574898,78.3163196450021,78.4072225261305,78.495550055249,78.5838648255518,
78.6721881152372,78.7650267599353,78.8534816417544,78.9419973428485,79.0306385596478,
79.0435426940296,79.1321726079931,79.2206892515459,79.3091163217373,79.4000192028333,
79.4883467320409,79.5766615024333,79.6649847922087,79.7578234367828,79.8462783186919,
79.9347940198762,80.0234352367649,80.0363393705052,80.1249692843794,80.2134859278426,
80.3019129979443,80.3928158790738,80.4811434081918,80.5694581784947,80.6577814681809,
80.7506201128808,80.8390749947023,80.9275906957994,81.0162319126024,81.0291360469808,
81.117765960863,81.2062826043335,81.294709674442,81.3856125555688,81.4739400846921,
81.5622548549999,81.6505781446904,81.7434167893819,81.8318716712063,81.9203873723059,
82.0090285891106,82.0219327234563,82.1105626375695,82.199079281272,82.2875063516133,
82.3784092326531,82.4667367620094,82.5550515325498,82.6433748224724,82.7362134668373,
82.8246683488902,82.913184050217,83.0018252672459,83.0147293999319,83.1020973209263,
83.1893527800484,83.2765115668103,83.3636169079208,83.4506912588376,83.5377570429396,
83.6248803500429,83.7120318592111,83.7992975896713,83.8718452601179),
 .UNSPECIFIED.);
#1449=B_SPLINE_CURVE_WITH_KNOTS('',3,(#23973,#23974,#23975,#23976,#23977,
#23978,#23979,#23980,#23981,#23982,#23983,#23984,#23985,#23986,#23987,#23988,
#23989,#23990,#23991,#23992,#23993,#23994,#23995,#23996,#23997,#23998,#23999,
#24000,#24001,#24002,#24003,#24004,#24005,#24006,#24007,#24008,#24009,#24010,
#24011,#24012,#24013,#24014,#24015,#24016,#24017,#24018,#24019,#24020,#24021,
#24022,#24023,#24024,#24025,#24026,#24027,#24028,#24029,#24030,#24031,#24032,
#24033,#24034,#24035,#24036,#24037,#24038,#24039,#24040,#24041,#24042,#24043,
#24044,#24045,#24046,#24047,#24048,#24049,#24050,#24051,#24052,#24053,#24054,
#24055,#24056,#24057,#24058,#24059,#24060,#24061,#24062,#24063,#24064,#24065,
#24066,#24067,#24068,#24069,#24070,#24071,#24072,#24073,#24074,#24075,#24076,
#24077,#24078,#24079,#24080,#24081,#24082,#24083,#24084,#24085,#24086,#24087,
#24088,#24089,#24090,#24091,#24092,#24093,#24094,#24095,#24096,#24097,#24098,
#24099,#24100,#24101,#24102,#24103,#24104,#24105,#24106,#24107,#24108,#24109,
#24110,#24111,#24112,#24113,#24114,#24115,#24116,#24117,#24118,#24119,#24120,
#24121,#24122,#24123,#24124,#24125,#24126,#24127,#24128,#24129,#24130,#24131,
#24132,#24133,#24134,#24135,#24136,#24137,#24138,#24139,#24140,#24141,#24142,
#24143,#24144,#24145,#24146,#24147,#24148,#24149,#24150,#24151,#24152,#24153,
#24154,#24155,#24156,#24157,#24158,#24159,#24160,#24161,#24162,#24163,#24164,
#24165,#24166,#24167,#24168,#24169,#24170,#24171,#24172,#24173,#24174,#24175,
#24176,#24177,#24178,#24179,#24180,#24181,#24182,#24183,#24184,#24185,#24186,
#24187,#24188,#24189,#24190,#24191,#24192,#24193,#24194,#24195,#24196,#24197,
#24198),.UNSPECIFIED.,.F.,.F.,(4,3,3,3,3,3,3,3,3,3,3,3,3,3,3,3,3,3,3,3,
3,3,3,3,3,3,3,3,3,3,3,3,3,3,3,3,3,3,3,3,3,3,3,3,3,3,3,3,3,3,3,3,3,3,3,3,
3,3,3,3,3,3,3,3,3,3,3,3,3,3,3,3,3,3,3,4),(83.87184526032,84.0075260764075,
84.0961559902256,84.1846726336294,84.2730997036684,84.3640025848202,84.452330113868,
84.540644884098,84.6289681737088,84.7218068185024,84.8102617002428,84.8987774012569,
84.9874186179747,85.0003227528831,85.0889526682576,85.1774693132255,85.2658963848344,
85.3567992654,85.4451267960223,85.5334415678257,85.621764859007,85.7146035015949,
85.8030583848844,85.8915740874398,85.980215305679,85.9931194293586,86.0817493404684,
86.1702659811702,86.2586930485167,86.3495959306814,86.4379234570766,86.5262382246736,
86.6145615116734,86.7074001602136,86.7958550394226,86.884370737933,86.973011952201,
86.9859161058342,87.074546020048,87.163062663826,87.2514897342175,87.342392615229,
87.4307201445741,87.5190349150805,87.6073582049465,87.7001968492873,87.7886517312281,
87.8771674324237,87.9658086492954,87.9787127823098,88.0673427067238,88.1558593607685,
88.2442864414803,88.3351893186435,88.423516858375,88.5118316392743,88.6001549395281,
88.6929935693425,88.7814484615617,88.8699641729969,88.9586053999911,88.9715094587854,
89.0601393486193,89.1486559680495,89.2370830141535,89.3279859042919,89.4163134096509,
89.504628156324,89.5929514225349,89.6857901007164,89.7742449596661,89.8627606381013,
89.9514018326752,89.964306135261,90.0930929644909,90.1550305674995),
 .UNSPECIFIED.);
#1450=B_SPLINE_CURVE_WITH_KNOTS('',3,(#24200,#24201,#24202,#24203,#24204,
#24205,#24206,#24207,#24208,#24209,#24210,#24211,#24212,#24213,#24214,#24215,
#24216,#24217,#24218,#24219,#24220,#24221,#24222,#24223,#24224,#24225,#24226,
#24227,#24228,#24229,#24230,#24231,#24232,#24233,#24234,#24235,#24236,#24237,
#24238,#24239,#24240,#24241,#24242,#24243,#24244,#24245,#24246,#24247,#24248,
#24249,#24250,#24251,#24252,#24253,#24254,#24255,#24256,#24257,#24258,#24259,
#24260,#24261,#24262,#24263,#24264,#24265,#24266,#24267,#24268,#24269,#24270,
#24271,#24272,#24273,#24274,#24275,#24276,#24277,#24278,#24279,#24280,#24281,
#24282,#24283,#24284,#24285,#24286,#24287,#24288,#24289,#24290,#24291,#24292,
#24293,#24294,#24295,#24296,#24297,#24298,#24299,#24300,#24301,#24302,#24303,
#24304,#24305,#24306,#24307,#24308,#24309,#24310,#24311,#24312,#24313,#24314,
#24315,#24316,#24317,#24318,#24319,#24320,#24321,#24322,#24323,#24324,#24325,
#24326,#24327,#24328,#24329,#24330,#24331,#24332,#24333,#24334,#24335,#24336,
#24337,#24338,#24339,#24340,#24341,#24342,#24343,#24344,#24345,#24346,#24347,
#24348,#24349,#24350,#24351,#24352,#24353,#24354,#24355,#24356,#24357,#24358,
#24359,#24360,#24361,#24362,#24363,#24364,#24365,#24366,#24367,#24368,#24369,
#24370,#24371,#24372,#24373,#24374,#24375,#24376,#24377,#24378,#24379,#24380,
#24381,#24382,#24383,#24384,#24385,#24386,#24387,#24388,#24389,#24390,#24391,
#24392,#24393,#24394,#24395,#24396,#24397,#24398,#24399,#24400,#24401,#24402,
#24403,#24404,#24405,#24406,#24407,#24408,#24409,#24410,#24411,#24412,#24413,
#24414,#24415,#24416,#24417,#24418,#24419,#24420,#24421,#24422,#24423,#24424,
#24425,#24426,#24427,#24428),.UNSPECIFIED.,.F.,.F.,(4,3,3,3,3,3,3,3,3,3,
3,3,3,3,3,3,3,3,3,3,3,3,3,3,3,3,3,3,3,3,3,3,3,3,3,3,3,3,3,3,3,3,3,3,3,3,
3,3,3,3,3,3,3,3,3,3,3,3,3,3,3,3,3,3,3,3,3,3,3,3,3,3,3,3,3,3,4),(90.1550305677032,
90.2422286500628,90.331587920272,90.4186598142627,90.5057103608812,90.5927619928027,
90.6838471975362,90.7710171033747,90.8582443197431,90.9455937102727,90.9571028117365,
91.0457327981164,91.1342495144537,91.2226766577066,91.3135795115198,91.4019071140074,
91.4902219576328,91.578545320514,91.6713838624385,91.7598388164566,91.8483545893981,
91.9369958771135,91.9498994882121,92.0385292015879,92.1270456444749,92.2154725141616,
92.3063754704774,92.394702800838,92.4830173733404,92.5713404663955,92.6641793909685,
92.7526340809014,92.8411495917615,92.929790621805,92.9426961646877,93.0313262273738,
93.1198430183502,93.2082702345105,93.2991730603421,93.3875007310339,93.4758156410106,
93.5641390683264,93.6569775115356,93.745432524614,93.8339483547674,93.9225896967489,
93.9354928411633,94.02412322868,94.1126403489231,94.2010678983342,94.2919706007473,
94.3802986123506,94.4686138654714,94.5569376377754,94.6497756077413,94.7382309671927,
94.8267471441431,94.9153888314088,94.9282895176388,95.0169178075138,95.1054328253063,
95.1938582700114,95.2847617605242,95.3730876751616,95.461400837815,95.5497225284144,
95.6425634448394,95.7310167637837,95.8195309146251,95.9081706083371,95.9210861941144,
96.0134105729702,96.1055811446663,96.1975615385315,96.2894289573287,96.3811619125729,
96.4382158746791),.UNSPECIFIED.);
#1451=B_SPLINE_CURVE_WITH_KNOTS('',3,(#24429,#24430,#24431,#24432,#24433,
#24434,#24435,#24436,#24437,#24438,#24439,#24440,#24441,#24442,#24443,#24444,
#24445,#24446,#24447,#24448,#24449,#24450,#24451,#24452,#24453,#24454,#24455,
#24456,#24457,#24458,#24459,#24460,#24461,#24462,#24463,#24464,#24465,#24466,
#24467,#24468,#24469,#24470,#24471,#24472,#24473,#24474,#24475,#24476,#24477,
#24478,#24479,#24480,#24481,#24482,#24483,#24484,#24485,#24486,#24487,#24488,
#24489,#24490,#24491,#24492,#24493,#24494,#24495,#24496,#24497,#24498,#24499,
#24500,#24501,#24502,#24503,#24504,#24505,#24506,#24507,#24508,#24509,#24510,
#24511,#24512,#24513,#24514,#24515,#24516,#24517,#24518,#24519,#24520,#24521,
#24522,#24523,#24524,#24525,#24526,#24527,#24528,#24529,#24530,#24531,#24532,
#24533,#24534,#24535,#24536,#24537,#24538,#24539,#24540,#24541,#24542,#24543,
#24544,#24545,#24546,#24547,#24548,#24549,#24550,#24551,#24552,#24553,#24554,
#24555,#24556,#24557,#24558,#24559,#24560,#24561,#24562,#24563,#24564,#24565,
#24566,#24567,#24568,#24569,#24570,#24571,#24572,#24573,#24574,#24575,#24576,
#24577,#24578,#24579,#24580,#24581,#24582,#24583,#24584,#24585,#24586,#24587,
#24588,#24589,#24590,#24591,#24592,#24593,#24594,#24595,#24596,#24597,#24598,
#24599,#24600,#24601,#24602,#24603,#24604,#24605,#24606,#24607,#24608,#24609,
#24610,#24611,#24612,#24613,#24614,#24615,#24616,#24617,#24618,#24619,#24620,
#24621,#24622,#24623,#24624,#24625,#24626,#24627,#24628,#24629,#24630,#24631,
#24632,#24633,#24634,#24635,#24636,#24637,#24638,#24639,#24640,#24641,#24642,
#24643,#24644,#24645,#24646,#24647,#24648,#24649,#24650,#24651,#24652,#24653,
#24654),.UNSPECIFIED.,.F.,.F.,(4,3,3,3,3,3,3,3,3,3,3,3,3,3,3,3,3,3,3,3,
3,3,3,3,3,3,3,3,3,3,3,3,3,3,3,3,3,3,3,3,3,3,3,3,3,3,3,3,3,3,3,3,3,3,3,3,
3,3,3,3,3,3,3,3,3,3,3,3,3,3,3,3,3,3,3,4),(96.43821587489,96.5315094285364,
96.6271027890498,96.7208092089047,96.8173460397473,96.91388287059,97.0025156379104,
97.0910351607441,97.1794651323696,97.2703669342066,97.3586974008322,97.447015116803,
97.5353413570371,97.6281759045442,97.7166337216183,97.8051523522997,97.8937964729189,
97.9066795470656,97.9952966599497,98.0838004811807,98.1722147232329,98.2631224107714,
98.3514371783157,98.4397392336869,98.5280498687933,98.6209064574802,98.7093489527241,
98.7978523607349,98.8864814906074,98.8994762235411,98.9881227028305,99.0766558550366,
99.1650993584394,99.2559960511365,99.3443397248907,99.4326705052216,99.5210096533517,
99.613825465018,99.7022956800214,99.7908265321604,99.8794825519452,99.8922729000167,
99.9809176811722,100.069449400606,100.157891734552,100.248788964794,100.337132121611,
100.425462626552,100.513801739934,100.606618699073,100.695089479045,100.783621101387,
100.872278175145,100.885069576492,100.973601443402,101.062019817221,101.150348512407,
101.241288229977,101.329517737987,101.417734784873,101.505960752869,101.594217025517,
101.682573743482,101.770990913672,101.859536359584,101.877866252968,101.965380714648,
102.052782232462,102.14008559453,102.227334731498,102.314552007684,102.401759755091,
102.489020034314,102.576307694746,102.663699300999,102.721401181691),
 .UNSPECIFIED.);
#1452=B_SPLINE_CURVE_WITH_KNOTS('',3,(#24657,#24658,#24659,#24660,#24661,
#24662,#24663,#24664,#24665,#24666,#24667,#24668,#24669,#24670,#24671,#24672,
#24673,#24674,#24675,#24676,#24677,#24678,#24679,#24680,#24681,#24682,#24683,
#24684,#24685,#24686,#24687,#24688,#24689,#24690,#24691,#24692,#24693,#24694,
#24695,#24696,#24697,#24698,#24699,#24700,#24701,#24702,#24703,#24704,#24705,
#24706,#24707,#24708,#24709,#24710,#24711,#24712,#24713,#24714,#24715,#24716,
#24717,#24718,#24719,#24720,#24721,#24722,#24723,#24724,#24725,#24726,#24727,
#24728,#24729,#24730,#24731,#24732,#24733,#24734,#24735,#24736,#24737,#24738,
#24739,#24740,#24741,#24742,#24743,#24744,#24745,#24746,#24747,#24748,#24749,
#24750,#24751,#24752,#24753,#24754,#24755,#24756,#24757,#24758,#24759,#24760,
#24761,#24762,#24763,#24764,#24765,#24766,#24767,#24768,#24769,#24770,#24771,
#24772,#24773,#24774,#24775,#24776,#24777,#24778,#24779,#24780,#24781,#24782,
#24783,#24784),.UNSPECIFIED.,.F.,.F.,(4,2,2,2,2,2,2,2,2,2,2,2,2,2,2,2,2,
2,2,2,2,2,2,2,2,2,2,2,2,2,2,2,2,2,2,2,2,2,2,2,2,2,2,2,2,2,2,2,2,2,2,2,2,
2,2,2,2,2,2,2,2,2,2,4),(0.00539620386092574,0.0581762748395569,0.0959465799780152,
0.114155907866814,0.129776929780304,0.14055985506542,0.150346261073067,
0.16647834135212,0.237291353387592,0.267515101724101,0.280511188113101,
0.290873769283408,0.297218081100971,0.303663604114955,0.314768974021879,
0.370321305386931,0.424463887562305,0.443465444336362,0.454819404756714,
0.465338872506723,0.479704411904614,0.516399202169655,0.57761423998528,
0.604512541065404,0.61325634689013,0.619213408423627,0.626006074952694,
0.639135832994514,0.699879326694402,0.753414703569547,0.76852834728937,
0.779073894490983,0.790001188858396,0.807203307949951,0.870090824473551,
0.923376749124762,0.933196757388839,0.939316960334243,0.945722527967118,
0.956813247809548,1.01214832155096,1.05354584725591,1.07260368326006,1.08870839604174,
1.09948989162646,1.11031322198308,1.12664871539946,1.19803286914717,1.22931305578496,
1.24254347292066,1.25301844025526,1.25930840592584,1.26559972502294,1.27612086586066,
1.33807763094068,1.39465125576289,1.40991623036985,1.42053776130304,1.43152512354768,
1.4487957670082,1.50163948973854,1.54490804705874,1.56065504609305,1.57246993836349),
 .UNSPECIFIED.);
#1453=B_SPLINE_CURVE_WITH_KNOTS('',3,(#24788,#24789,#24790,#24791,#24792,
#24793,#24794,#24795,#24796,#24797,#24798,#24799,#24800,#24801,#24802,#24803,
#24804,#24805,#24806,#24807,#24808,#24809,#24810,#24811,#24812,#24813,#24814,
#24815,#24816,#24817,#24818,#24819,#24820,#24821,#24822,#24823,#24824,#24825,
#24826,#24827,#24828,#24829,#24830,#24831,#24832,#24833,#24834,#24835,#24836,
#24837,#24838,#24839,#24840,#24841,#24842,#24843,#24844,#24845,#24846,#24847,
#24848,#24849,#24850,#24851,#24852,#24853,#24854,#24855,#24856,#24857,#24858,
#24859,#24860),.UNSPECIFIED.,.F.,.F.,(4,3,3,3,3,3,3,3,3,3,3,3,3,3,3,3,3,
3,3,3,3,3,3,3,4),(-47.1238898038469,-46.9950727644704,-46.9016897087544,
-46.8093989437482,-46.717232941916,-46.6251631638475,-46.5331552357951,
-46.4411785207822,-46.3492073946448,-46.2572162437137,-46.1651145240901,
-46.0729548859248,-45.9806268533618,-45.9088930322787,-45.8132628505972,
-45.71777443611,-45.6175646760721,-45.5223118547511,-45.4271236077411,-45.3319796663271,
-45.2368598072655,-45.1417182743927,-45.046565882262,-44.9513501488818,
-44.9160963558065),.UNSPECIFIED.);
#1454=B_SPLINE_CURVE_WITH_KNOTS('',3,(#24861,#24862,#24863,#24864,#24865,
#24866,#24867,#24868,#24869,#24870,#24871,#24872,#24873,#24874,#24875,#24876,
#24877,#24878,#24879,#24880,#24881,#24882,#24883,#24884,#24885,#24886,#24887,
#24888,#24889,#24890,#24891,#24892,#24893,#24894,#24895,#24896,#24897,#24898,
#24899,#24900),.UNSPECIFIED.,.F.,.F.,(4,2,2,2,2,2,2,2,2,2,2,2,2,2,2,2,2,
2,2,4),(-4.06042171078719,-3.99441154909979,-3.97878930540769,-3.96800786165842,
-3.95822415119664,-3.94210020820236,-3.87130478593638,-3.84103412307938,
-3.8280268247646,-3.81765891600555,-3.81131440486851,-3.80487196973302,
-3.79377772423557,-3.73802395486263,-3.67705048918811,-3.66158326588681,
-3.65088958922245,-3.63987943928295,-3.62267948655661,-3.60215374024631),
 .UNSPECIFIED.);
#1455=B_SPLINE_CURVE_WITH_KNOTS('',3,(#24948,#24949,#24950,#24951,#24952,
#24953,#24954,#24955,#24956,#24957,#24958,#24959,#24960,#24961),
 .UNSPECIFIED.,.F.,.F.,(4,2,2,2,2,2,4),(-0.361085602979245,-0.357000077685616,
-0.27844614120804,-0.199252098686416,-0.109491424797441,-0.0546153104605399,
-1.74415845322073E-7),.UNSPECIFIED.);
#1456=B_SPLINE_CURVE_WITH_KNOTS('',3,(#24963,#24964,#24965,#24966,#24967,
#24968,#24969,#24970,#24971),.UNSPECIFIED.,.F.,.F.,(4,1,1,1,1,1,4),(-0.0350009483246411,
-0.0280198882249107,-0.016804534164689,-0.00558918010446727,0.00562617395575443,
0.0280568820761978,0.0350536140949925),.UNSPECIFIED.);
#1457=B_SPLINE_CURVE_WITH_KNOTS('',3,(#24973,#24974,#24975,#24976,#24977,
#24978,#24979,#24980,#24981,#24982,#24983,#24984,#24985,#24986),
 .UNSPECIFIED.,.F.,.F.,(4,2,2,2,2,2,4),(-0.469080395753844,-0.397348524872784,
-0.325269326748868,-0.207248260222546,-0.103131005525517,0.,0.00535949284075881),
 .UNSPECIFIED.);
#1458=B_SPLINE_CURVE_WITH_KNOTS('',3,(#24997,#24998,#24999,#25000,#25001,
#25002,#25003,#25004,#25005,#25006,#25007,#25008,#25009,#25010,#25011,#25012,
#25013,#25014,#25015,#25016,#25017,#25018,#25019,#25020,#25021,#25022,#25023,
#25024,#25025,#25026,#25027,#25028,#25029,#25030,#25031,#25032,#25033,#25034,
#25035,#25036,#25037,#25038,#25039,#25040,#25041,#25042,#25043,#25044,#25045),
 .UNSPECIFIED.,.F.,.F.,(4,3,3,3,3,3,3,3,3,3,3,3,3,3,3,3,4),(-0.0350029095584539,
-0.0326784650318294,-0.03034917662837,-0.0280198882249105,-0.0254680596894552,
-0.0229200914464411,-0.0203748859852383,-0.0178336153267085,-0.0168045341646888,
-0.0144744152626023,-0.0121456081055165,-0.00981763332868959,-0.00748893840388418,
-0.00558918010446715,-0.00301830868335975,-0.000444599004916765,-5.90823278986403E-12),
 .UNSPECIFIED.);
#1459=B_SPLINE_CURVE_WITH_KNOTS('',3,(#25048,#25049,#25050,#25051,#25052,
#25053),.UNSPECIFIED.,.F.,.F.,(4,2,4),(-0.954074778386004,-0.905023768660029,
-0.855972758934053),.UNSPECIFIED.);
#1460=B_SPLINE_CURVE_WITH_KNOTS('',3,(#25055,#25056,#25057,#25058,#25059,
#25060,#25061),.UNSPECIFIED.,.F.,.F.,(4,3,4),(-0.0490510097259763,0.,0.0490510097259751),
 .UNSPECIFIED.);
#1461=B_SPLINE_CURVE_WITH_KNOTS('',3,(#25064,#25065,#25066,#25067,#25068,
#25069,#25070,#25071,#25072,#25073,#25074,#25075,#25076,#25077,#25078,#25079,
#25080,#25081,#25082,#25083,#25084,#25085,#25086,#25087,#25088,#25089,#25090,
#25091,#25092,#25093,#25094,#25095,#25096,#25097,#25098,#25099,#25100,#25101,
#25102,#25103,#25104,#25105,#25106,#25107,#25108,#25109,#25110,#25111,#25112),
 .UNSPECIFIED.,.F.,.F.,(4,3,3,3,3,3,3,3,3,3,3,3,3,3,3,3,4),(3.46944695195361E-18,
0.00256903169244048,0.00514025006054238,0.00562617395575452,0.00815140445096736,
0.0106763863582272,0.0132007974759858,0.0157247394590576,0.0168415280159762,
0.0191777755034903,0.0215148133424174,0.0238521887988676,0.0261921437071731,
0.0280568820761979,0.0305976323694871,0.033145591663878,0.0350439246442522),
 .UNSPECIFIED.);
#1462=B_SPLINE_CURVE_WITH_KNOTS('',3,(#25167,#25168,#25169,#25170,#25171,
#25172,#25173,#25174,#25175,#25176,#25177,#25178,#25179,#25180),
 .UNSPECIFIED.,.F.,.F.,(4,2,2,2,2,2,4),(-0.00536726751032349,-9.33357504392246E-9,
0.103199017039813,0.207237213246338,0.325156745312053,0.39724917198956,
0.468998855549633),.UNSPECIFIED.);
#1463=B_SPLINE_CURVE_WITH_KNOTS('',3,(#25182,#25183,#25184,#25185,#25186,
#25187,#25188,#25189,#25190,#25191,#25192,#25193,#25194,#25195),
 .UNSPECIFIED.,.F.,.F.,(4,2,2,2,2,2,4),(1.29845166431681E-6,0.0546083462055371,
0.109479711095743,0.199263575998483,0.278476799071752,0.357016538590781,
0.361096115615465),.UNSPECIFIED.);
#1464=B_SPLINE_CURVE_WITH_KNOTS('',3,(#25424,#25425,#25426,#25427,#25428,
#25429,#25430,#25431,#25432,#25433,#25434,#25435,#25436,#25437,#25438,#25439,
#25440,#25441,#25442,#25443,#25444,#25445,#25446,#25447,#25448,#25449,#25450,
#25451,#25452,#25453,#25454,#25455,#25456,#25457,#25458,#25459,#25460,#25461,
#25462,#25463,#25464,#25465,#25466,#25467,#25468,#25469,#25470,#25471,#25472,
#25473,#25474,#25475,#25476,#25477,#25478,#25479,#25480,#25481,#25482,#25483,
#25484,#25485,#25486,#25487,#25488,#25489,#25490,#25491,#25492,#25493,#25494,
#25495,#25496,#25497,#25498,#25499,#25500,#25501,#25502,#25503,#25504,#25505,
#25506,#25507,#25508,#25509,#25510,#25511,#25512,#25513,#25514,#25515,#25516,
#25517,#25518,#25519,#25520,#25521,#25522,#25523),.UNSPECIFIED.,.F.,.F.,
(4,3,3,3,3,3,3,3,3,3,3,3,3,3,3,3,3,3,3,3,3,3,3,3,3,3,3,3,3,3,3,3,3,4),(-2.19769548978374,
-2.16996208153018,-2.13535871400152,-2.10082245618501,-2.09476556787962,
-2.08923073045232,-2.0551999841314,-2.02127001257704,-1.99454552012076,
-1.98991819571071,-1.95669919080343,-1.92379392379268,-1.89175881298667,
-1.87244139578649,-1.86490525090243,-1.85913416106667,-1.85495455874982,
-1.82334168177451,-1.81899725957887,-1.78691133993479,-1.75455244345232,
-1.73856969434239,-1.73229684856998,-1.72680262056442,-1.69537207398216,
-1.66392310425677,-1.63300450698346,-1.61621134169549,-1.60686948326227,
-1.60236537222576,-1.57213504949349,-1.54232837915983,-1.51334659517059,
-1.49894425059128),.UNSPECIFIED.);
#1465=B_SPLINE_CURVE_WITH_KNOTS('',3,(#25525,#25526,#25527,#25528,#25529,
#25530,#25531,#25532,#25533,#25534,#25535,#25536,#25537,#25538,#25539,#25540,
#25541,#25542,#25543,#25544,#25545,#25546,#25547,#25548,#25549,#25550,#25551,
#25552,#25553,#25554,#25555,#25556,#25557,#25558,#25559,#25560,#25561,#25562,
#25563,#25564,#25565,#25566,#25567,#25568,#25569,#25570,#25571,#25572,#25573,
#25574,#25575,#25576,#25577,#25578,#25579,#25580,#25581,#25582,#25583,#25584,
#25585,#25586,#25587,#25588,#25589,#25590,#25591,#25592,#25593,#25594,#25595,
#25596,#25597,#25598,#25599,#25600,#25601,#25602,#25603,#25604,#25605,#25606,
#25607,#25608,#25609,#25610,#25611,#25612,#25613,#25614,#25615,#25616,#25617,
#25618,#25619,#25620,#25621),.UNSPECIFIED.,.F.,.F.,(4,3,3,3,3,3,3,3,3,3,
3,3,3,3,3,3,3,3,3,3,3,3,3,3,3,3,3,3,3,3,3,3,4),(-2.19794260024569,-2.16379459538134,
-2.12909478229254,-2.09474478574741,-2.0892597211607,-2.05520722562912,
-2.02140659959258,-1.99927981030521,-1.99390270623858,-1.98887593211283,
-1.95581388327196,-1.92314427933987,-1.89138524127318,-1.86791965517696,
-1.8605499603638,-1.85650011315063,-1.84464664343001,-1.81269774603171,
-1.78035895899146,-1.74810662597683,-1.73375644174792,-1.72933691089787,
-1.69753405795295,-1.66620981151358,-1.63416765531588,-1.61814657721703,
-1.61003028450692,-1.60438481581443,-1.60212549911818,-1.57201964467436,
-1.5426911199921,-1.52221163485995,-1.49894425059015),.UNSPECIFIED.);
#1466=B_SPLINE_CURVE_WITH_KNOTS('',3,(#25622,#25623,#25624,#25625),
 .UNSPECIFIED.,.F.,.F.,(4,4),(-0.0136507999019738,0.),.UNSPECIFIED.);
#1467=B_SPLINE_CURVE_WITH_KNOTS('',3,(#25851,#25852,#25853,#25854,#25855,
#25856,#25857,#25858,#25859,#25860,#25861,#25862,#25863,#25864,#25865,#25866,
#25867,#25868,#25869,#25870,#25871,#25872,#25873,#25874,#25875,#25876,#25877,
#25878,#25879,#25880,#25881,#25882,#25883,#25884,#25885,#25886,#25887,#25888,
#25889,#25890,#25891,#25892,#25893,#25894,#25895,#25896,#25897,#25898,#25899,
#25900,#25901,#25902,#25903,#25904,#25905,#25906,#25907,#25908,#25909,#25910,
#25911,#25912,#25913,#25914,#25915,#25916,#25917,#25918,#25919,#25920,#25921,
#25922,#25923,#25924,#25925,#25926,#25927,#25928,#25929,#25930,#25931,#25932,
#25933,#25934,#25935,#25936,#25937,#25938,#25939,#25940,#25941,#25942,#25943,
#25944),.UNSPECIFIED.,.F.,.F.,(4,3,3,3,3,3,3,3,3,3,3,3,3,3,3,3,3,3,3,3,
3,3,3,3,3,3,3,3,3,3,3,4),(-232.946686419845,-232.920698623695,-232.888128466004,
-232.854634003,-232.836299126277,-232.828986333775,-232.82374876418,-232.789594601998,
-232.753900834196,-232.718207066393,-232.707936860927,-232.703263378653,
-232.667316137156,-232.631177781828,-232.595515553508,-232.577842315535,
-232.562697236381,-232.560080409211,-232.524280232497,-232.488406293369,
-232.451648585627,-232.416879702357,-232.409368374264,-232.371464878899,
-232.333481887168,-232.295618139985,-232.276686266394,-232.264081625322,
-232.257754392803,-232.218756617189,-232.179856440503,-232.164324022216),
 .UNSPECIFIED.);
#1468=B_SPLINE_CURVE_WITH_KNOTS('',3,(#25945,#25946,#25947,#25948),
 .UNSPECIFIED.,.F.,.F.,(4,4),(0.,0.0138563661205195),.UNSPECIFIED.);
#1469=B_SPLINE_CURVE_WITH_KNOTS('',3,(#25949,#25950,#25951,#25952,#25953,
#25954,#25955,#25956,#25957,#25958,#25959,#25960,#25961,#25962,#25963,#25964,
#25965,#25966,#25967,#25968,#25969,#25970,#25971,#25972,#25973,#25974,#25975,
#25976,#25977,#25978,#25979,#25980,#25981,#25982,#25983,#25984,#25985,#25986,
#25987,#25988,#25989,#25990,#25991,#25992,#25993,#25994,#25995,#25996,#25997,
#25998,#25999,#26000,#26001,#26002,#26003,#26004,#26005,#26006,#26007,#26008,
#26009,#26010,#26011,#26012,#26013,#26014,#26015,#26016,#26017,#26018,#26019,
#26020,#26021,#26022,#26023,#26024,#26025,#26026,#26027,#26028,#26029,#26030,
#26031,#26032,#26033,#26034,#26035,#26036,#26037,#26038,#26039),
 .UNSPECIFIED.,.F.,.F.,(4,3,3,3,3,3,3,3,3,3,3,3,3,3,3,3,3,3,3,3,3,3,3,3,
3,3,3,3,3,3,4),(-482.256901778709,-482.224225803402,-482.190525587978,-482.156852378964,
-482.150327631204,-482.144056954824,-482.109513167315,-482.074286620043,
-482.051899343887,-482.039111838982,-482.033818937828,-481.99768233578,
-481.961478406429,-481.925962153481,-481.896304483897,-481.891074900579,
-481.855343675935,-481.819332394006,-481.782400925057,-481.748150002002,
-481.740976721928,-481.703311159677,-481.665167855225,-481.62701437128,
-481.595344288617,-481.589293307268,-481.584346741121,-481.545122580121,
-481.50612183907,-481.500182765298,-481.468537766939),.UNSPECIFIED.);
#1691=VERTEX_POINT('',#19193);
#1692=VERTEX_POINT('',#19194);
#1693=VERTEX_POINT('',#19196);
#1694=VERTEX_POINT('',#19275);
#1695=VERTEX_POINT('',#19336);
#1696=VERTEX_POINT('',#19337);
#1697=VERTEX_POINT('',#19507);
#1698=VERTEX_POINT('',#19564);
#1699=VERTEX_POINT('',#19565);
#1700=VERTEX_POINT('',#19567);
#1701=VERTEX_POINT('',#19734);
#1702=VERTEX_POINT('',#19865);
#1703=VERTEX_POINT('',#19866);
#1704=VERTEX_POINT('',#20211);
#1705=VERTEX_POINT('',#20212);
#1706=VERTEX_POINT('',#20214);
#1707=VERTEX_POINT('',#20387);
#1708=VERTEX_POINT('',#20563);
#1709=VERTEX_POINT('',#20564);
#1710=VERTEX_POINT('',#20895);
#1711=VERTEX_POINT('',#20896);
#1712=VERTEX_POINT('',#20898);
#1713=VERTEX_POINT('',#21067);
#1714=VERTEX_POINT('',#21272);
#1715=VERTEX_POINT('',#21273);
#1716=VERTEX_POINT('',#21437);
#1717=VERTEX_POINT('',#21618);
#1718=VERTEX_POINT('',#21619);
#1719=VERTEX_POINT('',#21657);
#1720=VERTEX_POINT('',#21659);
#1721=VERTEX_POINT('',#21661);
#1722=VERTEX_POINT('',#21672);
#1723=VERTEX_POINT('',#21899);
#1724=VERTEX_POINT('',#22126);
#1725=VERTEX_POINT('',#22353);
#1726=VERTEX_POINT('',#22580);
#1727=VERTEX_POINT('',#22807);
#1728=VERTEX_POINT('',#23034);
#1729=VERTEX_POINT('',#23045);
#1730=VERTEX_POINT('',#23052);
#1731=VERTEX_POINT('',#23054);
#1732=VERTEX_POINT('',#23064);
#1733=VERTEX_POINT('',#23291);
#1734=VERTEX_POINT('',#23518);
#1735=VERTEX_POINT('',#23745);
#1736=VERTEX_POINT('',#23972);
#1737=VERTEX_POINT('',#24199);
#1738=VERTEX_POINT('',#24656);
#1739=VERTEX_POINT('',#24785);
#1740=VERTEX_POINT('',#24787);
#1741=VERTEX_POINT('',#24946);
#1742=VERTEX_POINT('',#24947);
#1743=VERTEX_POINT('',#24962);
#1744=VERTEX_POINT('',#24972);
#1745=VERTEX_POINT('',#24989);
#1746=VERTEX_POINT('',#24991);
#1747=VERTEX_POINT('',#24995);
#1748=VERTEX_POINT('',#24996);
#1749=VERTEX_POINT('',#25046);
#1750=VERTEX_POINT('',#25054);
#1751=VERTEX_POINT('',#25062);
#1752=VERTEX_POINT('',#25113);
#1753=VERTEX_POINT('',#25166);
#1754=VERTEX_POINT('',#25181);
#1755=VERTEX_POINT('',#25524);
#1756=VERTEX_POINT('',#25850);
#2206=EDGE_CURVE('',#1691,#1692,#1053,.T.);
#2207=EDGE_CURVE('',#1693,#1691,#1410,.F.);
#2208=EDGE_CURVE('',#1694,#1693,#199,.F.);
#2209=EDGE_CURVE('',#1694,#1692,#1411,.T.);
#2210=EDGE_CURVE('',#1695,#1696,#1054,.T.);
#2211=EDGE_CURVE('',#1691,#1695,#1412,.F.);
#2212=EDGE_CURVE('',#1692,#1697,#1413,.T.);
#2213=EDGE_CURVE('',#1697,#1696,#1414,.T.);
#2214=EDGE_CURVE('',#1698,#1699,#1055,.T.);
#2215=EDGE_CURVE('',#1700,#1698,#1415,.F.);
#2216=EDGE_CURVE('',#1695,#1700,#1416,.F.);
#2217=EDGE_CURVE('',#1696,#1701,#1417,.T.);
#2218=EDGE_CURVE('',#1701,#1699,#1418,.T.);
#2219=EDGE_CURVE('',#1702,#1703,#1056,.T.);
#2220=EDGE_CURVE('',#1698,#1702,#1419,.F.);
#2221=EDGE_CURVE('',#1699,#1703,#1420,.T.);
#2222=EDGE_CURVE('',#1704,#1705,#1057,.T.);
#2223=EDGE_CURVE('',#1706,#1704,#1421,.F.);
#2224=EDGE_CURVE('',#1702,#1706,#1422,.F.);
#2225=EDGE_CURVE('',#1703,#1707,#1423,.T.);
#2226=EDGE_CURVE('',#1707,#1705,#1424,.T.);
#2227=EDGE_CURVE('',#1708,#1709,#1058,.T.);
#2228=EDGE_CURVE('',#1704,#1708,#1425,.F.);
#2229=EDGE_CURVE('',#1705,#1709,#1426,.T.);
#2230=EDGE_CURVE('',#1710,#1711,#1059,.T.);
#2231=EDGE_CURVE('',#1712,#1710,#1427,.F.);
#2232=EDGE_CURVE('',#1708,#1712,#1428,.F.);
#2233=EDGE_CURVE('',#1709,#1713,#1429,.T.);
#2234=EDGE_CURVE('',#1713,#1711,#1430,.T.);
#2235=EDGE_CURVE('',#1714,#1715,#1060,.T.);
#2236=EDGE_CURVE('',#1710,#1714,#1431,.F.);
#2237=EDGE_CURVE('',#1711,#1716,#1432,.T.);
#2238=EDGE_CURVE('',#1716,#1715,#1433,.F.);
#2239=EDGE_CURVE('',#1717,#1718,#1434,.T.);
#2240=EDGE_CURVE('',#1719,#1718,#200,.T.);
#2241=EDGE_CURVE('',#1719,#1720,#201,.T.);
#2242=EDGE_CURVE('',#1720,#1721,#1435,.T.);
#2243=EDGE_CURVE('',#1721,#1722,#1436,.T.);
#2244=EDGE_CURVE('',#1722,#1723,#1437,.T.);
#2245=EDGE_CURVE('',#1723,#1724,#1438,.T.);
#2246=EDGE_CURVE('',#1724,#1725,#1439,.T.);
#2247=EDGE_CURVE('',#1725,#1726,#1440,.T.);
#2248=EDGE_CURVE('',#1726,#1727,#1441,.T.);
#2249=EDGE_CURVE('',#1727,#1728,#1442,.T.);
#2250=EDGE_CURVE('',#1728,#1729,#1443,.T.);
#2251=EDGE_CURVE('',#1730,#1729,#202,.F.);
#2252=EDGE_CURVE('',#1730,#1731,#1444,.T.);
#2253=EDGE_CURVE('',#1731,#1732,#1445,.T.);
#2254=EDGE_CURVE('',#1732,#1733,#1446,.T.);
#2255=EDGE_CURVE('',#1733,#1734,#1447,.T.);
#2256=EDGE_CURVE('',#1734,#1735,#1448,.T.);
#2257=EDGE_CURVE('',#1735,#1736,#1449,.T.);
#2258=EDGE_CURVE('',#1736,#1737,#1450,.T.);
#2259=EDGE_CURVE('',#1737,#1717,#1451,.T.);
#2260=EDGE_CURVE('',#1715,#1738,#1452,.F.);
#2261=EDGE_CURVE('',#1739,#1738,#203,.T.);
#2262=EDGE_CURVE('',#1740,#1739,#1453,.T.);
#2263=EDGE_CURVE('',#1714,#1740,#1454,.F.);
#2264=EDGE_CURVE('',#1741,#1742,#1455,.T.);
#2265=EDGE_CURVE('',#1742,#1743,#1456,.T.);
#2266=EDGE_CURVE('',#1743,#1744,#1457,.T.);
#2267=EDGE_CURVE('',#1744,#1741,#1061,.T.);
#2268=EDGE_CURVE('',#1745,#1743,#1062,.T.);
#2269=EDGE_CURVE('',#1746,#1745,#204,.T.);
#2270=EDGE_CURVE('',#1742,#1746,#1063,.T.);
#2271=EDGE_CURVE('',#1747,#1748,#1458,.T.);
#2272=EDGE_CURVE('',#1747,#1749,#1064,.T.);
#2273=EDGE_CURVE('',#1749,#1745,#1459,.T.);
#2274=EDGE_CURVE('',#1746,#1750,#1460,.T.);
#2275=EDGE_CURVE('',#1750,#1751,#1065,.T.);
#2276=EDGE_CURVE('',#1748,#1751,#1461,.T.);
#2277=EDGE_CURVE('',#1748,#1752,#1066,.T.);
#2278=EDGE_CURVE('',#1752,#1752,#205,.F.);
#2279=EDGE_CURVE('',#1753,#1747,#1462,.T.);
#2280=EDGE_CURVE('',#1751,#1754,#1463,.T.);
#2281=EDGE_CURVE('',#1754,#1753,#1067,.T.);
#2282=EDGE_CURVE('',#1749,#1750,#206,.T.);
#2283=EDGE_CURVE('',#1729,#1739,#1464,.T.);
#2284=EDGE_CURVE('',#1755,#1719,#1465,.F.);
#2285=EDGE_CURVE('',#1755,#1693,#1466,.T.);
#2286=EDGE_CURVE('',#1756,#1730,#1467,.T.);
#2287=EDGE_CURVE('',#1738,#1756,#1468,.T.);
#2288=EDGE_CURVE('',#1718,#1694,#1469,.F.);
#3083=ORIENTED_EDGE('',*,*,#2206,.F.);
#3084=ORIENTED_EDGE('',*,*,#2207,.F.);
#3085=ORIENTED_EDGE('',*,*,#2208,.F.);
#3086=ORIENTED_EDGE('',*,*,#2209,.T.);
#3087=ORIENTED_EDGE('',*,*,#2210,.F.);
#3088=ORIENTED_EDGE('',*,*,#2211,.F.);
#3089=ORIENTED_EDGE('',*,*,#2206,.T.);
#3090=ORIENTED_EDGE('',*,*,#2212,.T.);
#3091=ORIENTED_EDGE('',*,*,#2213,.T.);
#3092=ORIENTED_EDGE('',*,*,#2214,.F.);
#3093=ORIENTED_EDGE('',*,*,#2215,.F.);
#3094=ORIENTED_EDGE('',*,*,#2216,.F.);
#3095=ORIENTED_EDGE('',*,*,#2210,.T.);
#3096=ORIENTED_EDGE('',*,*,#2217,.T.);
#3097=ORIENTED_EDGE('',*,*,#2218,.T.);
#3098=ORIENTED_EDGE('',*,*,#2219,.F.);
#3099=ORIENTED_EDGE('',*,*,#2220,.F.);
#3100=ORIENTED_EDGE('',*,*,#2214,.T.);
#3101=ORIENTED_EDGE('',*,*,#2221,.T.);
#3102=ORIENTED_EDGE('',*,*,#2222,.F.);
#3103=ORIENTED_EDGE('',*,*,#2223,.F.);
#3104=ORIENTED_EDGE('',*,*,#2224,.F.);
#3105=ORIENTED_EDGE('',*,*,#2219,.T.);
#3106=ORIENTED_EDGE('',*,*,#2225,.T.);
#3107=ORIENTED_EDGE('',*,*,#2226,.T.);
#3108=ORIENTED_EDGE('',*,*,#2227,.F.);
#3109=ORIENTED_EDGE('',*,*,#2228,.F.);
#3110=ORIENTED_EDGE('',*,*,#2222,.T.);
#3111=ORIENTED_EDGE('',*,*,#2229,.T.);
#3112=ORIENTED_EDGE('',*,*,#2230,.F.);
#3113=ORIENTED_EDGE('',*,*,#2231,.F.);
#3114=ORIENTED_EDGE('',*,*,#2232,.F.);
#3115=ORIENTED_EDGE('',*,*,#2227,.T.);
#3116=ORIENTED_EDGE('',*,*,#2233,.T.);
#3117=ORIENTED_EDGE('',*,*,#2234,.T.);
#3118=ORIENTED_EDGE('',*,*,#2235,.F.);
#3119=ORIENTED_EDGE('',*,*,#2236,.F.);
#3120=ORIENTED_EDGE('',*,*,#2230,.T.);
#3121=ORIENTED_EDGE('',*,*,#2237,.T.);
#3122=ORIENTED_EDGE('',*,*,#2238,.T.);
#3123=ORIENTED_EDGE('',*,*,#2239,.T.);
#3124=ORIENTED_EDGE('',*,*,#2240,.F.);
#3125=ORIENTED_EDGE('',*,*,#2241,.T.);
#3126=ORIENTED_EDGE('',*,*,#2242,.T.);
#3127=ORIENTED_EDGE('',*,*,#2243,.T.);
#3128=ORIENTED_EDGE('',*,*,#2244,.T.);
#3129=ORIENTED_EDGE('',*,*,#2245,.T.);
#3130=ORIENTED_EDGE('',*,*,#2246,.T.);
#3131=ORIENTED_EDGE('',*,*,#2247,.T.);
#3132=ORIENTED_EDGE('',*,*,#2248,.T.);
#3133=ORIENTED_EDGE('',*,*,#2249,.T.);
#3134=ORIENTED_EDGE('',*,*,#2250,.T.);
#3135=ORIENTED_EDGE('',*,*,#2251,.F.);
#3136=ORIENTED_EDGE('',*,*,#2252,.T.);
#3137=ORIENTED_EDGE('',*,*,#2253,.T.);
#3138=ORIENTED_EDGE('',*,*,#2254,.T.);
#3139=ORIENTED_EDGE('',*,*,#2255,.T.);
#3140=ORIENTED_EDGE('',*,*,#2256,.T.);
#3141=ORIENTED_EDGE('',*,*,#2257,.T.);
#3142=ORIENTED_EDGE('',*,*,#2258,.T.);
#3143=ORIENTED_EDGE('',*,*,#2259,.T.);
#3144=ORIENTED_EDGE('',*,*,#2235,.T.);
#3145=ORIENTED_EDGE('',*,*,#2260,.T.);
#3146=ORIENTED_EDGE('',*,*,#2261,.F.);
#3147=ORIENTED_EDGE('',*,*,#2262,.F.);
#3148=ORIENTED_EDGE('',*,*,#2263,.F.);
#3149=ORIENTED_EDGE('',*,*,#2264,.T.);
#3150=ORIENTED_EDGE('',*,*,#2265,.T.);
#3151=ORIENTED_EDGE('',*,*,#2266,.T.);
#3152=ORIENTED_EDGE('',*,*,#2267,.T.);
#3153=ORIENTED_EDGE('',*,*,#2266,.F.);
#3154=ORIENTED_EDGE('',*,*,#2268,.F.);
#3155=ORIENTED_EDGE('',*,*,#2269,.F.);
#3156=ORIENTED_EDGE('',*,*,#2270,.F.);
#3157=ORIENTED_EDGE('',*,*,#2264,.F.);
#3158=ORIENTED_EDGE('',*,*,#2267,.F.);
#3159=ORIENTED_EDGE('',*,*,#2271,.F.);
#3160=ORIENTED_EDGE('',*,*,#2272,.T.);
#3161=ORIENTED_EDGE('',*,*,#2273,.T.);
#3162=ORIENTED_EDGE('',*,*,#2268,.T.);
#3163=ORIENTED_EDGE('',*,*,#2265,.F.);
#3164=ORIENTED_EDGE('',*,*,#2270,.T.);
#3165=ORIENTED_EDGE('',*,*,#2274,.T.);
#3166=ORIENTED_EDGE('',*,*,#2275,.T.);
#3167=ORIENTED_EDGE('',*,*,#2276,.F.);
#3168=ORIENTED_EDGE('',*,*,#2277,.T.);
#3169=ORIENTED_EDGE('',*,*,#2278,.T.);
#3170=ORIENTED_EDGE('',*,*,#2277,.F.);
#3171=ORIENTED_EDGE('',*,*,#2279,.T.);
#3172=ORIENTED_EDGE('',*,*,#2271,.T.);
#3173=ORIENTED_EDGE('',*,*,#2276,.T.);
#3174=ORIENTED_EDGE('',*,*,#2280,.T.);
#3175=ORIENTED_EDGE('',*,*,#2281,.T.);
#3176=ORIENTED_EDGE('',*,*,#2273,.F.);
#3177=ORIENTED_EDGE('',*,*,#2282,.T.);
#3178=ORIENTED_EDGE('',*,*,#2274,.F.);
#3179=ORIENTED_EDGE('',*,*,#2269,.T.);
#3180=ORIENTED_EDGE('',*,*,#2280,.F.);
#3181=ORIENTED_EDGE('',*,*,#2275,.F.);
#3182=ORIENTED_EDGE('',*,*,#2282,.F.);
#3183=ORIENTED_EDGE('',*,*,#2272,.F.);
#3184=ORIENTED_EDGE('',*,*,#2279,.F.);
#3185=ORIENTED_EDGE('',*,*,#2281,.F.);
#3186=ORIENTED_EDGE('',*,*,#2283,.F.);
#3187=ORIENTED_EDGE('',*,*,#2250,.F.);
#3188=ORIENTED_EDGE('',*,*,#2249,.F.);
#3189=ORIENTED_EDGE('',*,*,#2248,.F.);
#3190=ORIENTED_EDGE('',*,*,#2247,.F.);
#3191=ORIENTED_EDGE('',*,*,#2246,.F.);
#3192=ORIENTED_EDGE('',*,*,#2245,.F.);
#3193=ORIENTED_EDGE('',*,*,#2244,.F.);
#3194=ORIENTED_EDGE('',*,*,#2243,.F.);
#3195=ORIENTED_EDGE('',*,*,#2242,.F.);
#3196=ORIENTED_EDGE('',*,*,#2241,.F.);
#3197=ORIENTED_EDGE('',*,*,#2284,.F.);
#3198=ORIENTED_EDGE('',*,*,#2285,.T.);
#3199=ORIENTED_EDGE('',*,*,#2207,.T.);
#3200=ORIENTED_EDGE('',*,*,#2211,.T.);
#3201=ORIENTED_EDGE('',*,*,#2216,.T.);
#3202=ORIENTED_EDGE('',*,*,#2215,.T.);
#3203=ORIENTED_EDGE('',*,*,#2220,.T.);
#3204=ORIENTED_EDGE('',*,*,#2224,.T.);
#3205=ORIENTED_EDGE('',*,*,#2223,.T.);
#3206=ORIENTED_EDGE('',*,*,#2228,.T.);
#3207=ORIENTED_EDGE('',*,*,#2232,.T.);
#3208=ORIENTED_EDGE('',*,*,#2231,.T.);
#3209=ORIENTED_EDGE('',*,*,#2236,.T.);
#3210=ORIENTED_EDGE('',*,*,#2263,.T.);
#3211=ORIENTED_EDGE('',*,*,#2262,.T.);
#3212=ORIENTED_EDGE('',*,*,#2286,.F.);
#3213=ORIENTED_EDGE('',*,*,#2287,.F.);
#3214=ORIENTED_EDGE('',*,*,#2260,.F.);
#3215=ORIENTED_EDGE('',*,*,#2238,.F.);
#3216=ORIENTED_EDGE('',*,*,#2237,.F.);
#3217=ORIENTED_EDGE('',*,*,#2234,.F.);
#3218=ORIENTED_EDGE('',*,*,#2233,.F.);
#3219=ORIENTED_EDGE('',*,*,#2229,.F.);
#3220=ORIENTED_EDGE('',*,*,#2226,.F.);
#3221=ORIENTED_EDGE('',*,*,#2225,.F.);
#3222=ORIENTED_EDGE('',*,*,#2221,.F.);
#3223=ORIENTED_EDGE('',*,*,#2218,.F.);
#3224=ORIENTED_EDGE('',*,*,#2217,.F.);
#3225=ORIENTED_EDGE('',*,*,#2213,.F.);
#3226=ORIENTED_EDGE('',*,*,#2212,.F.);
#3227=ORIENTED_EDGE('',*,*,#2209,.F.);
#3228=ORIENTED_EDGE('',*,*,#2288,.F.);
#3229=ORIENTED_EDGE('',*,*,#2239,.F.);
#3230=ORIENTED_EDGE('',*,*,#2259,.F.);
#3231=ORIENTED_EDGE('',*,*,#2258,.F.);
#3232=ORIENTED_EDGE('',*,*,#2257,.F.);
#3233=ORIENTED_EDGE('',*,*,#2256,.F.);
#3234=ORIENTED_EDGE('',*,*,#2255,.F.);
#3235=ORIENTED_EDGE('',*,*,#2254,.F.);
#3236=ORIENTED_EDGE('',*,*,#2253,.F.);
#3237=ORIENTED_EDGE('',*,*,#2252,.F.);
#3238=ORIENTED_EDGE('',*,*,#2283,.T.);
#3239=ORIENTED_EDGE('',*,*,#2261,.T.);
#3240=ORIENTED_EDGE('',*,*,#2287,.T.);
#3241=ORIENTED_EDGE('',*,*,#2286,.T.);
#3242=ORIENTED_EDGE('',*,*,#2251,.T.);
#3243=ORIENTED_EDGE('',*,*,#2278,.F.);
#3244=ORIENTED_EDGE('',*,*,#2284,.T.);
#3245=ORIENTED_EDGE('',*,*,#2240,.T.);
#3246=ORIENTED_EDGE('',*,*,#2288,.T.);
#3247=ORIENTED_EDGE('',*,*,#2208,.T.);
#3248=ORIENTED_EDGE('',*,*,#2285,.F.);
#4074=CYLINDRICAL_SURFACE('',#4580,3.22275);
#4075=CYLINDRICAL_SURFACE('',#4582,3.22275);
#4076=CYLINDRICAL_SURFACE('',#4583,3.22275);
#4077=CYLINDRICAL_SURFACE('',#4584,3.22275);
#4078=CYLINDRICAL_SURFACE('',#4585,3.22275);
#4079=CYLINDRICAL_SURFACE('',#4586,3.22275);
#4080=CYLINDRICAL_SURFACE('',#4587,3.22275);
#4081=CYLINDRICAL_SURFACE('',#4588,3.22275);
#4082=CYLINDRICAL_SURFACE('',#4589,3.933);
#4083=CYLINDRICAL_SURFACE('',#4593,3.22275);
#4084=CYLINDRICAL_SURFACE('',#4597,3.);
#4085=CYLINDRICAL_SURFACE('',#4599,24.5);
#4212=ADVANCED_FACE('',(#577),#4074,.T.);
#4213=ADVANCED_FACE('',(#578),#4075,.T.);
#4214=ADVANCED_FACE('',(#579),#4076,.T.);
#4215=ADVANCED_FACE('',(#580),#4077,.T.);
#4216=ADVANCED_FACE('',(#581),#4078,.T.);
#4217=ADVANCED_FACE('',(#582),#4079,.T.);
#4218=ADVANCED_FACE('',(#583),#4080,.T.);
#4219=ADVANCED_FACE('',(#584),#4081,.T.);
#4220=ADVANCED_FACE('',(#585),#4082,.T.);
#4221=ADVANCED_FACE('',(#586),#4083,.T.);
#4222=ADVANCED_FACE('',(#587),#51,.F.);
#4223=ADVANCED_FACE('',(#588),#139,.T.);
#4224=ADVANCED_FACE('',(#589),#4084,.T.);
#4225=ADVANCED_FACE('',(#590),#52,.F.);
#4226=ADVANCED_FACE('',(#591),#4085,.F.);
#4227=ADVANCED_FACE('',(#592),#140,.F.);
#4228=ADVANCED_FACE('',(#593),#53,.F.);
#4229=ADVANCED_FACE('',(#594),#54,.F.);
#4230=ADVANCED_FACE('',(#595,#101),#141,.F.);
#4231=ADVANCED_FACE('',(#596),#142,.T.);
#4387=CLOSED_SHELL('',(#4212,#4213,#4214,#4215,#4216,#4217,#4218,#4219,
#4220,#4221,#4222,#4223,#4224,#4225,#4226,#4227,#4228,#4229,#4230,#4231));
#4579=AXIS2_PLACEMENT_3D('',#19191,#5242,#5243);
#4580=AXIS2_PLACEMENT_3D('',#19192,#5244,#5245);
#4581=AXIS2_PLACEMENT_3D('',#19276,#5247,#5248);
#4582=AXIS2_PLACEMENT_3D('',#19335,#5249,#5250);
#4583=AXIS2_PLACEMENT_3D('',#19563,#5252,#5253);
#4584=AXIS2_PLACEMENT_3D('',#19864,#5255,#5256);
#4585=AXIS2_PLACEMENT_3D('',#20210,#5258,#5259);
#4586=AXIS2_PLACEMENT_3D('',#20562,#5261,#5262);
#4587=AXIS2_PLACEMENT_3D('',#20894,#5264,#5265);
#4588=AXIS2_PLACEMENT_3D('',#21271,#5267,#5268);
#4589=AXIS2_PLACEMENT_3D('',#21617,#5270,#5271);
#4590=AXIS2_PLACEMENT_3D('',#21658,#5272,#5273);
#4591=AXIS2_PLACEMENT_3D('',#21660,#5274,#5275);
#4592=AXIS2_PLACEMENT_3D('',#23053,#5276,#5277);
#4593=AXIS2_PLACEMENT_3D('',#24655,#5278,#5279);
#4594=AXIS2_PLACEMENT_3D('',#24786,#5280,#5281);
#4595=AXIS2_PLACEMENT_3D('',#24988,#5283,#5284);
#4596=AXIS2_PLACEMENT_3D('',#24992,#5286,#5287);
#4597=AXIS2_PLACEMENT_3D('',#24994,#5289,#5290);
#4598=AXIS2_PLACEMENT_3D('',#25115,#5294,#5295);
#4599=AXIS2_PLACEMENT_3D('',#25197,#5297,#5298);
#4600=AXIS2_PLACEMENT_3D('',#25198,#5299,#5300);
#4601=AXIS2_PLACEMENT_3D('',#25199,#5301,#5302);
#4602=AXIS2_PLACEMENT_3D('',#26040,#5303,#5304);
#4603=AXIS2_PLACEMENT_3D('',#26041,#5305,#5306);
#5242=DIRECTION('axis',(0.,0.,1.));
#5243=DIRECTION('refdir',(1.,0.,0.));
#5244=DIRECTION('center_axis',(1.22464679914735E-16,0.,-1.));
#5245=DIRECTION('ref_axis',(0.152224682118134,0.988345914219325,1.86421469707196E-17));
#5246=DIRECTION('',(-1.22464679914735E-16,0.,1.));
#5247=DIRECTION('center_axis',(1.22464679914735E-16,0.,-1.));
#5248=DIRECTION('ref_axis',(1.,-4.63459159752748E-15,1.22464679914735E-16));
#5249=DIRECTION('center_axis',(1.22464679914735E-16,0.,-1.));
#5250=DIRECTION('ref_axis',(0.152224682118134,0.988345914219325,1.86421469707196E-17));
#5251=DIRECTION('',(-1.22464679914735E-16,0.,1.));
#5252=DIRECTION('center_axis',(1.22464679914735E-16,0.,-1.));
#5253=DIRECTION('ref_axis',(0.152224682118134,0.988345914219325,1.86421469707196E-17));
#5254=DIRECTION('',(-1.22464679914735E-16,0.,1.));
#5255=DIRECTION('center_axis',(1.22464679914735E-16,0.,-1.));
#5256=DIRECTION('ref_axis',(0.152224682118134,0.988345914219325,1.86421469707196E-17));
#5257=DIRECTION('',(-1.22464679914735E-16,0.,1.));
#5258=DIRECTION('center_axis',(1.22464679914735E-16,0.,-1.));
#5259=DIRECTION('ref_axis',(0.152224682118134,0.988345914219325,1.86421469707196E-17));
#5260=DIRECTION('',(-1.22464679914735E-16,0.,1.));
#5261=DIRECTION('center_axis',(1.22464679914735E-16,0.,-1.));
#5262=DIRECTION('ref_axis',(0.152224682118134,0.988345914219325,1.86421469707196E-17));
#5263=DIRECTION('',(-1.22464679914735E-16,0.,1.));
#5264=DIRECTION('center_axis',(1.22464679914735E-16,0.,-1.));
#5265=DIRECTION('ref_axis',(0.152224682118134,0.988345914219325,1.86421469707196E-17));
#5266=DIRECTION('',(-1.22464679914735E-16,0.,1.));
#5267=DIRECTION('center_axis',(1.22464679914735E-16,0.,-1.));
#5268=DIRECTION('ref_axis',(0.152224682118134,0.988345914219325,1.86421469707196E-17));
#5269=DIRECTION('',(-1.22464679914735E-16,0.,1.));
#5270=DIRECTION('center_axis',(1.22464679914735E-16,0.,-1.));
#5271=DIRECTION('ref_axis',(1.,0.,1.22464679914735E-16));
#5272=DIRECTION('center_axis',(-1.22464679914735E-16,0.,1.));
#5273=DIRECTION('ref_axis',(1.,0.,1.22464679914735E-16));
#5274=DIRECTION('center_axis',(0.00374951423302316,-0.05043654781332,-0.998720228986923));
#5275=DIRECTION('ref_axis',(-0.999992969847666,-0.000226459877875131,-0.00374285601754598));
#5276=DIRECTION('center_axis',(-1.22464679914735E-16,0.,1.));
#5277=DIRECTION('ref_axis',(1.,0.,1.22464679914735E-16));
#5278=DIRECTION('center_axis',(1.22464679914735E-16,0.,-1.));
#5279=DIRECTION('ref_axis',(-0.533717072258489,0.845663104776262,-6.53614904191654E-17));
#5280=DIRECTION('center_axis',(1.22464679914735E-16,0.,-1.));
#5281=DIRECTION('ref_axis',(1.,-4.63459159752748E-15,1.22464679914735E-16));
#5282=DIRECTION('',(-2.22044604925031E-16,1.,-2.71926214689378E-32));
#5283=DIRECTION('center_axis',(-1.,-2.22044604925031E-16,0.));
#5284=DIRECTION('ref_axis',(-2.22044604925031E-16,1.,0.));
#5285=DIRECTION('',(1.22464679914735E-16,0.,-1.));
#5286=DIRECTION('center_axis',(1.,2.22044604925031E-16,0.));
#5287=DIRECTION('ref_axis',(-2.22044604925031E-16,1.,0.));
#5288=DIRECTION('',(-1.22464679914735E-16,0.,1.));
#5289=DIRECTION('center_axis',(1.22464679914735E-16,0.,-1.));
#5290=DIRECTION('ref_axis',(1.,0.,1.22464679914735E-16));
#5291=DIRECTION('',(-1.22464679914735E-16,0.,1.));
#5292=DIRECTION('',(1.22464679914735E-16,0.,-1.));
#5293=DIRECTION('',(-1.22464679914735E-16,0.,1.));
#5294=DIRECTION('center_axis',(-1.22464679914735E-16,0.,1.));
#5295=DIRECTION('ref_axis',(1.,0.,1.22464679914735E-16));
#5296=DIRECTION('',(2.22044604925031E-16,-1.,2.71926214689378E-32));
#5297=DIRECTION('center_axis',(1.,2.22044604925031E-16,0.));
#5298=DIRECTION('ref_axis',(-2.22044604925031E-16,1.,0.));
#5299=DIRECTION('center_axis',(-1.,-2.22044604925031E-16,0.));
#5300=DIRECTION('ref_axis',(-2.22044604925031E-16,1.,0.));
#5301=DIRECTION('center_axis',(-1.,-2.22044604925031E-16,0.));
#5302=DIRECTION('ref_axis',(-2.22044604925031E-16,1.,0.));
#5303=DIRECTION('center_axis',(-1.22464679914735E-16,0.,1.));
#5304=DIRECTION('ref_axis',(1.,0.,1.22464679914735E-16));
#5305=DIRECTION('center_axis',(-1.22464679914735E-16,0.,1.));
#5306=DIRECTION('ref_axis',(1.,0.,1.22464679914735E-16));
#19191=CARTESIAN_POINT('',(0.,0.,0.));
#19192=CARTESIAN_POINT('Origin',(-9.35406549764863E-15,0.,41.4527091182931));
#19193=CARTESIAN_POINT('',(-0.490582094004581,-3.18519179509525,59.6160848123881));
#19194=CARTESIAN_POINT('',(-0.490582094296225,-3.18519179505033,59.8598970253053));
#19195=CARTESIAN_POINT('',(-0.490582094296226,-3.18519179505033,41.4527091182931));
#19196=CARTESIAN_POINT('',(1.13209532136445,3.01736271366979,60.1999356690201));
#19197=CARTESIAN_POINT('Ctrl Pts',(-0.490582094004581,-3.18519179509525,
59.6160848123881));
#19198=CARTESIAN_POINT('Ctrl Pts',(-0.466375895170159,-3.18892002512848,
59.6176608165468));
#19199=CARTESIAN_POINT('Ctrl Pts',(-0.44212674100936,-3.19237238887795,
59.6192250328061));
#19200=CARTESIAN_POINT('Ctrl Pts',(-0.396256821284568,-3.19837018876251,
59.6221535062883));
#19201=CARTESIAN_POINT('Ctrl Pts',(-0.374645516026424,-3.20097362267201,
59.6235205400371));
#19202=CARTESIAN_POINT('Ctrl Pts',(-0.333052645145843,-3.20555714064656,
59.6261250060645));
#19203=CARTESIAN_POINT('Ctrl Pts',(-0.313076378368531,-3.20756977232229,
59.6273639259856));
#19204=CARTESIAN_POINT('Ctrl Pts',(-0.262072309293849,-3.21222746711234,
59.6304992915734));
#19205=CARTESIAN_POINT('Ctrl Pts',(-0.231021674373692,-3.21460982794318,
59.6323819053628));
#19206=CARTESIAN_POINT('Ctrl Pts',(-0.0805560152715602,-3.22396276634906,
59.6413991700732));
#19207=CARTESIAN_POINT('Ctrl Pts',(0.0391609941865398,-3.22473212080751,
59.6482541382956));
#19208=CARTESIAN_POINT('Ctrl Pts',(0.43886979987491,-3.20503081182403,59.6708602154157));
#19209=CARTESIAN_POINT('Ctrl Pts',(0.716061572440631,-3.15469193878349,
59.6861891204382));
#19210=CARTESIAN_POINT('Ctrl Pts',(1.03301637608063,-3.05315038340598,59.7058218783413));
#19211=CARTESIAN_POINT('Ctrl Pts',(1.08240011258963,-3.03599401084699,59.7089401750122));
#19212=CARTESIAN_POINT('Ctrl Pts',(1.16121272272251,-3.00644643952529,59.7140246722272));
#19213=CARTESIAN_POINT('Ctrl Pts',(1.19091385650328,-2.99480537843232,59.7159659508861));
#19214=CARTESIAN_POINT('Ctrl Pts',(1.25303898938089,-2.96938574951514,59.7200822291794));
#19215=CARTESIAN_POINT('Ctrl Pts',(1.28541949756136,-2.95551264542692,59.7222602062979));
#19216=CARTESIAN_POINT('Ctrl Pts',(1.36418413392361,-2.92022750926507,59.7276411218214));
#19217=CARTESIAN_POINT('Ctrl Pts',(1.41029773245226,-2.89823858354922,59.7308633404735));
#19218=CARTESIAN_POINT('Ctrl Pts',(1.63893656584088,-2.78246508563171,59.7472128487559));
#19219=CARTESIAN_POINT('Ctrl Pts',(1.81270655083574,-2.67250743335119,59.7608970333487));
#19220=CARTESIAN_POINT('Ctrl Pts',(2.12096735680935,-2.43347809547221,59.7872362977809));
#19221=CARTESIAN_POINT('Ctrl Pts',(2.25709670507903,-2.30777854232686,59.7998004278076));
#19222=CARTESIAN_POINT('Ctrl Pts',(2.40647463047983,-2.14390996659559,59.8141619193305));
#19223=CARTESIAN_POINT('Ctrl Pts',(2.43078442458745,-2.11630750052144,59.8165189672957));
#19224=CARTESIAN_POINT('Ctrl Pts',(2.46836942512819,-2.0721294217034,59.8201868595273));
#19225=CARTESIAN_POINT('Ctrl Pts',(2.48196177180597,-2.05582921992575,59.8215184242811));
#19226=CARTESIAN_POINT('Ctrl Pts',(2.50838504765398,-2.02349785094601,59.8241150723412));
#19227=CARTESIAN_POINT('Ctrl Pts',(2.52122566236738,-2.00747610250023,59.8253807760125));
#19228=CARTESIAN_POINT('Ctrl Pts',(2.5542877803926,-1.96540551653022,59.8286530477838));
#19229=CARTESIAN_POINT('Ctrl Pts',(2.57426472204498,-1.93916637770799,59.8306435928132));
#19230=CARTESIAN_POINT('Ctrl Pts',(2.61808593901863,-1.87973752235793,59.8350519563479));
#19231=CARTESIAN_POINT('Ctrl Pts',(2.64170902997236,-1.84639129742178,59.8374577640492));
#19232=CARTESIAN_POINT('Ctrl Pts',(2.71612113110418,-1.73699871641069,59.8451645108149));
#19233=CARTESIAN_POINT('Ctrl Pts',(2.76431174415411,-1.65923506117146,59.8503605265539));
#19234=CARTESIAN_POINT('Ctrl Pts',(2.93297905210031,-1.35926558431107,59.8697510245403));
#19235=CARTESIAN_POINT('Ctrl Pts',(3.03048391545008,-1.12522434000235,59.8836647266481));
#19236=CARTESIAN_POINT('Ctrl Pts',(3.11555328128316,-0.826329071483372,
59.901918998409));
#19237=CARTESIAN_POINT('Ctrl Pts',(3.12994056709405,-0.770041180393835,
59.9053722827996));
#19238=CARTESIAN_POINT('Ctrl Pts',(3.15094484383266,-0.677509049131582,
59.9110913581827));
#19239=CARTESIAN_POINT('Ctrl Pts',(3.15847575578115,-0.641484723233521,
59.9133281255906));
#19240=CARTESIAN_POINT('Ctrl Pts',(3.17205235309447,-0.570491287869983,
59.9177598819685));
#19241=CARTESIAN_POINT('Ctrl Pts',(3.17814063409056,-0.535535612651706,
59.9199531817326));
#19242=CARTESIAN_POINT('Ctrl Pts',(3.19154663989022,-0.450258705028328,
59.9253339451069));
#19243=CARTESIAN_POINT('Ctrl Pts',(3.19825272073982,-0.399852381390727,
59.9285398504902));
#19244=CARTESIAN_POINT('Ctrl Pts',(3.22400176597381,-0.163690560424752,
59.9436861980883));
#19245=CARTESIAN_POINT('Ctrl Pts',(3.2280675827124,0.0233108727131432,59.956072016989));
#19246=CARTESIAN_POINT('Ctrl Pts',(3.20247622072898,0.415987853826625,59.9825671308802));
#19247=CARTESIAN_POINT('Ctrl Pts',(3.16918513870429,0.620624948438658,59.996658636168));
#19248=CARTESIAN_POINT('Ctrl Pts',(3.10760221945617,0.854487606245626,60.0122770652714));
#19249=CARTESIAN_POINT('Ctrl Pts',(3.09814625203067,0.888161388407426,60.0145128509176));
#19250=CARTESIAN_POINT('Ctrl Pts',(3.08212434475082,0.941843968345828,60.0180489549775));
#19251=CARTESIAN_POINT('Ctrl Pts',(3.07590742140784,0.96195330177375,60.0193671516632));
#19252=CARTESIAN_POINT('Ctrl Pts',(3.06294421370395,1.00247309036875,60.0220083455839));
#19253=CARTESIAN_POINT('Ctrl Pts',(3.05618995538499,1.02287954771957,60.0233309268158));
#19254=CARTESIAN_POINT('Ctrl Pts',(3.03746359697704,1.07761502246025,60.0268618253843));
#19255=CARTESIAN_POINT('Ctrl Pts',(3.02511362905335,1.11181249018656,60.0290501400996));
#19256=CARTESIAN_POINT('Ctrl Pts',(2.99566979811199,1.18921753426789,60.0339783334769));
#19257=CARTESIAN_POINT('Ctrl Pts',(2.97821477328465,1.23227960679994,60.0367019836912));
#19258=CARTESIAN_POINT('Ctrl Pts',(2.91459243148628,1.37998062975321,60.0460295075257));
#19259=CARTESIAN_POINT('Ctrl Pts',(2.86378998912396,1.48253337704519,60.0524823778576));
#19260=CARTESIAN_POINT('Ctrl Pts',(2.70497413440088,1.76435964979148,60.0706896566574));
#19261=CARTESIAN_POINT('Ctrl Pts',(2.58482820751392,1.93610549366955,60.0823948713236));
#19262=CARTESIAN_POINT('Ctrl Pts',(2.41214944726657,2.13795423692312,60.0980315056522));
#19263=CARTESIAN_POINT('Ctrl Pts',(2.37427869853996,2.17993426077273,60.1013975765543));
#19264=CARTESIAN_POINT('Ctrl Pts',(2.31004064640055,2.24748213765211,60.1070220496124));
#19265=CARTESIAN_POINT('Ctrl Pts',(2.28430482472564,2.27363476560337,60.1092541670205));
#19266=CARTESIAN_POINT('Ctrl Pts',(2.2324062628475,2.32460311483087,60.1137179329303));
#19267=CARTESIAN_POINT('Ctrl Pts',(2.20626240307468,2.3494304433298,60.1159485948593));
#19268=CARTESIAN_POINT('Ctrl Pts',(2.14068633235918,2.4096444098886,60.1215033095447));
#19269=CARTESIAN_POINT('Ctrl Pts',(2.10078869149829,2.44450618879101,60.1248482219604));
#19270=CARTESIAN_POINT('Ctrl Pts',(1.90786010743347,2.60487098737753,60.1408718581635));
#19271=CARTESIAN_POINT('Ctrl Pts',(1.74436168343103,2.71706901506309,60.1540525438222));
#19272=CARTESIAN_POINT('Ctrl Pts',(1.43042747819915,2.89243075262105,60.1783204117256));
#19273=CARTESIAN_POINT('Ctrl Pts',(1.28349855475448,2.96055718234145,60.1893044281946));
#19274=CARTESIAN_POINT('Ctrl Pts',(1.13209532136445,3.01736271366979,60.1999356690201));
#19275=CARTESIAN_POINT('',(3.22243683749933,-0.0449265047301805,60.1999356690201));
#19276=CARTESIAN_POINT('Origin',(-1.16499385964724E-14,0.,60.1999356690201));
#19277=CARTESIAN_POINT('Ctrl Pts',(3.22243683749933,-0.0449265047301373,
60.1999356690201));
#19278=CARTESIAN_POINT('Ctrl Pts',(3.22101092976798,-0.147202380139736,
60.1936214602585));
#19279=CARTESIAN_POINT('Ctrl Pts',(3.21471055926815,-0.249479982211946,
60.1873072514969));
#19280=CARTESIAN_POINT('Ctrl Pts',(3.20354864224502,-0.351274336196089,
60.1809930427352));
#19281=CARTESIAN_POINT('Ctrl Pts',(3.19239330626173,-0.453008672470304,
60.1746825568161));
#19282=CARTESIAN_POINT('Ctrl Pts',(3.17638217460513,-0.554259925593877,
60.168372070897));
#19283=CARTESIAN_POINT('Ctrl Pts',(3.15558010482072,-0.654546991865061,
60.1620615849779));
#19284=CARTESIAN_POINT('Ctrl Pts',(3.13478544122438,-0.754798352801083,
60.1557533457894));
#19285=CARTESIAN_POINT('Ctrl Pts',(3.10920331875166,-0.854085813901753,
60.1494451066008));
#19286=CARTESIAN_POINT('Ctrl Pts',(3.07894980895765,-0.951937832224118,
60.1431368674123));
#19287=CARTESIAN_POINT('Ctrl Pts',(3.04869173594916,-1.04980460981743,60.1368276767358));
#19288=CARTESIAN_POINT('Ctrl Pts',(3.01376098015525,-1.14623512221458,60.1305184860594));
#19289=CARTESIAN_POINT('Ctrl Pts',(2.97432361185473,-1.24077258773048,60.1242092953829));
#19290=CARTESIAN_POINT('Ctrl Pts',(2.93488064524815,-1.33532347325103,60.1178992090894));
#19291=CARTESIAN_POINT('Ctrl Pts',(2.89092994848673,-1.42798040218852,60.1115891227959));
#19292=CARTESIAN_POINT('Ctrl Pts',(2.8426855484529,-1.51830709512831,60.1052790365023));
#19293=CARTESIAN_POINT('Ctrl Pts',(2.79442405525234,-1.60866579114455,60.0989667145222));
#19294=CARTESIAN_POINT('Ctrl Pts',(2.74186602143725,-1.6966922496596,60.0926543925422));
#19295=CARTESIAN_POINT('Ctrl Pts',(2.68527085912993,-1.78197586280161,60.0863420705621));
#19296=CARTESIAN_POINT('Ctrl Pts',(2.62864362117743,-1.86730781093911,60.0800261710359));
#19297=CARTESIAN_POINT('Ctrl Pts',(2.56797492387656,-1.94989348117759,60.0737102715097));
#19298=CARTESIAN_POINT('Ctrl Pts',(2.5035664258784,-2.02935278197616,60.0673943719836));
#19299=CARTESIAN_POINT('Ctrl Pts',(2.43906397980174,-2.10892798438494,60.0610692599056));
#19300=CARTESIAN_POINT('Ctrl Pts',(2.37081109528922,-2.18536739509907,60.0547441478276));
#19301=CARTESIAN_POINT('Ctrl Pts',(2.29914871747955,-2.25832520630048,60.0484190357497));
#19302=CARTESIAN_POINT('Ctrl Pts',(2.22742777450882,-2.3313426413393,60.0420887545548));
#19303=CARTESIAN_POINT('Ctrl Pts',(2.15229208193654,-2.40087253046784,60.03575847336));
#19304=CARTESIAN_POINT('Ctrl Pts',(2.0741169120997,-2.4666083186112,60.0294281921651));
#19305=CARTESIAN_POINT('Ctrl Pts',(1.99580700126858,-2.53245740750558,60.0230870002376));
#19306=CARTESIAN_POINT('Ctrl Pts',(1.91444747085521,-2.59449908689812,60.01674580831));
#19307=CARTESIAN_POINT('Ctrl Pts',(1.83044415092502,-2.65246899564243,60.0104046163824));
#19308=CARTESIAN_POINT('Ctrl Pts',(1.79520837690052,-2.67678487513901,60.007744759534));
#19309=CARTESIAN_POINT('Ctrl Pts',(1.7595077589201,-2.70038489766776,60.0050849026856));
#19310=CARTESIAN_POINT('Ctrl Pts',(1.72337351315524,-2.72325197083467,60.0024250458372));
#19311=CARTESIAN_POINT('Ctrl Pts',(1.64020134900485,-2.7758863602572,59.9963027082671));
#19312=CARTESIAN_POINT('Ctrl Pts',(1.55444527987673,-2.82481460533337,59.9901803706971));
#19313=CARTESIAN_POINT('Ctrl Pts',(1.46647257452095,-2.86976928526979,59.984058033127));
#19314=CARTESIAN_POINT('Ctrl Pts',(1.37861964988799,-2.91466275640246,59.977944031529));
#19315=CARTESIAN_POINT('Ctrl Pts',(1.28855647077179,-2.95559320632361,59.9718300299311));
#19316=CARTESIAN_POINT('Ctrl Pts',(1.19667952715909,-2.99233615621278,59.9657160283331));
#19317=CARTESIAN_POINT('Ctrl Pts',(1.10490206849107,-3.0290393205998,59.9596086470154));
#19318=CARTESIAN_POINT('Ctrl Pts',(1.01131515358769,-3.0615638277795,59.9535012656977));
#19319=CARTESIAN_POINT('Ctrl Pts',(0.916339171499791,-3.08973139370966,
59.9473938843799));
#19320=CARTESIAN_POINT('Ctrl Pts',(0.821439567103826,-3.11787630787434,
59.9412914144901));
#19321=CARTESIAN_POINT('Ctrl Pts',(0.725153537258198,-3.14167111718934,
59.9351889446002));
#19322=CARTESIAN_POINT('Ctrl Pts',(0.627919684477241,-3.16098630688999,
59.9290864747104));
#19323=CARTESIAN_POINT('Ctrl Pts',(0.530722109627871,-3.18029429009711,
59.9229862816509));
#19324=CARTESIAN_POINT('Ctrl Pts',(0.432577846179468,-3.19512588160265,
59.9168860885914));
#19325=CARTESIAN_POINT('Ctrl Pts',(0.33393795614733,-3.20540215947144,59.9107858955319));
#19326=CARTESIAN_POINT('Ctrl Pts',(0.235322441552297,-3.21567589791358,
59.9046872099241));
#19327=CARTESIAN_POINT('Ctrl Pts',(0.136211984133432,-3.2213965184783,59.8985885243163));
#19328=CARTESIAN_POINT('Ctrl Pts',(0.0370637567284713,-3.22253686409282,
59.8924898387085));
#19329=CARTESIAN_POINT('Ctrl Pts',(-0.0621272755162565,-3.22367770202387,
59.8863885201413));
#19330=CARTESIAN_POINT('Ctrl Pts',(-0.161355667492033,-3.2202343090346,
59.8802872015741));
#19331=CARTESIAN_POINT('Ctrl Pts',(-0.260163824525399,-3.21223167702897,
59.8741858830069));
#19332=CARTESIAN_POINT('Ctrl Pts',(-0.337297735829324,-3.20598447714331,
59.8694229304397));
#19333=CARTESIAN_POINT('Ctrl Pts',(-0.414175491816498,-3.19695991247447,
59.8646599778725));
#19334=CARTESIAN_POINT('Ctrl Pts',(-0.490582094296224,-3.18519179505033,
59.8598970253053));
#19335=CARTESIAN_POINT('Origin',(-9.35406549764863E-15,0.,41.4527091182931));
#19336=CARTESIAN_POINT('',(-0.490581924382687,-3.18519182122035,58.3609184893942));
#19337=CARTESIAN_POINT('',(-0.491343452670647,-3.19000126486617,58.6097459619479));
#19338=CARTESIAN_POINT('',(-0.490582094296226,-3.18519179505033,41.4527091182931));
#19339=CARTESIAN_POINT('Ctrl Pts',(-0.490581924382689,-3.18519182122035,
58.3609184893942));
#19340=CARTESIAN_POINT('Ctrl Pts',(-0.313703096115372,-3.2124346250527,
58.372562612839));
#19341=CARTESIAN_POINT('Ctrl Pts',(-0.134819049917065,-3.22490326967685,
58.3846048681688));
#19342=CARTESIAN_POINT('Ctrl Pts',(0.213309713732562,-3.22012646871349,
58.4081231419546));
#19343=CARTESIAN_POINT('Ctrl Pts',(0.381972481551577,-3.20450027907013,
58.4195482726045));
#19344=CARTESIAN_POINT('Ctrl Pts',(0.581198292875902,-3.17008165946916,
58.4325854790762));
#19345=CARTESIAN_POINT('Ctrl Pts',(0.613668753933233,-3.16395639032679,
58.4346949780006));
#19346=CARTESIAN_POINT('Ctrl Pts',(0.666140544478564,-3.15321982369106,
58.4380728141072));
#19347=CARTESIAN_POINT('Ctrl Pts',(0.686201526583494,-3.14891505444317,
58.4393567997329));
#19348=CARTESIAN_POINT('Ctrl Pts',(0.726994056028932,-3.13975325387554,
58.4419506707305));
#19349=CARTESIAN_POINT('Ctrl Pts',(0.747721116497325,-3.13488182288204,
58.4432597536929));
#19350=CARTESIAN_POINT('Ctrl Pts',(0.804152273584797,-3.12102739914996,
58.4468033048302));
#19351=CARTESIAN_POINT('Ctrl Pts',(0.83975417535615,-3.11163720365094,58.4490163528802));
#19352=CARTESIAN_POINT('Ctrl Pts',(1.05406394661899,-3.05116543984785,58.4622441253629));
#19353=CARTESIAN_POINT('Ctrl Pts',(1.22825785813371,-2.98530722730326,58.4726122106591));
#19354=CARTESIAN_POINT('Ctrl Pts',(1.57976380370304,-2.81640072209273,58.4944567086959));
#19355=CARTESIAN_POINT('Ctrl Pts',(1.75487935639104,-2.71074790002801,58.5059088620402));
#19356=CARTESIAN_POINT('Ctrl Pts',(1.96004769788926,-2.55870346551206,58.5209938996047));
#19357=CARTESIAN_POINT('Ctrl Pts',(2.000535331318,-2.52717398632152,58.5240583963101));
#19358=CARTESIAN_POINT('Ctrl Pts',(2.06766872466423,-2.47226982710916,58.5293018773251));
#19359=CARTESIAN_POINT('Ctrl Pts',(2.09471359160369,-2.44939724587851,58.5314607942696));
#19360=CARTESIAN_POINT('Ctrl Pts',(2.14878115026405,-2.40212041392816,58.5358758510144));
#19361=CARTESIAN_POINT('Ctrl Pts',(2.175778143979,-2.37769472619929,58.538132698705));
#19362=CARTESIAN_POINT('Ctrl Pts',(2.24376084273435,-2.31405952963211,58.5439547307397));
#19363=CARTESIAN_POINT('Ctrl Pts',(2.28413438119453,-2.27421716445005,58.5475464012496));
#19364=CARTESIAN_POINT('Ctrl Pts',(2.47380812468861,-2.07689122462769,58.5650924324503));
#19365=CARTESIAN_POINT('Ctrl Pts',(2.60797711574984,-1.90568436478878,58.5796528804779));
#19366=CARTESIAN_POINT('Ctrl Pts',(2.81397497938702,-1.57989297976098,58.605690530354));
#19367=CARTESIAN_POINT('Ctrl Pts',(2.89273425250105,-1.43059952526935,58.617074753674));
#19368=CARTESIAN_POINT('Ctrl Pts',(2.9725637041962,-1.24542294069209,58.6300790631077));
#19369=CARTESIAN_POINT('Ctrl Pts',(2.98519943069331,-1.21482419831584,58.6321926584));
#19370=CARTESIAN_POINT('Ctrl Pts',(3.00490376937524,-1.16494303527081,58.6355752686292));
#19371=CARTESIAN_POINT('Ctrl Pts',(3.01226327023129,-1.14577877567449,58.6368600128917));
#19372=CARTESIAN_POINT('Ctrl Pts',(3.02687619020863,-1.10661226115654,58.6394536912039));
#19373=CARTESIAN_POINT('Ctrl Pts',(3.03411559754703,-1.08660607708896,58.6407618501997));
#19374=CARTESIAN_POINT('Ctrl Pts',(3.05331303451801,-1.03186550227272,58.6442996352647));
#19375=CARTESIAN_POINT('Ctrl Pts',(3.06487652096581,-0.996995019063621,
58.6465079617242));
#19376=CARTESIAN_POINT('Ctrl Pts',(3.13197827491077,-0.782432865897649,
58.6598637329304));
#19377=CARTESIAN_POINT('Ctrl Pts',(3.1723005566129,-0.598342716944537,58.6703478981932));
#19378=CARTESIAN_POINT('Ctrl Pts',(3.21360917368962,-0.277687063164398,
58.6884580376908));
#19379=CARTESIAN_POINT('Ctrl Pts',(3.22242778506983,-0.142655399222014,
58.6960374992979));
#19380=CARTESIAN_POINT('Ctrl Pts',(3.22288686970446,0.0552716915044153,
58.7074246911002));
#19381=CARTESIAN_POINT('Ctrl Pts',(3.22119986485595,0.118006423353004,58.7110735185706));
#19382=CARTESIAN_POINT('Ctrl Pts',(3.21470368769381,0.233714683625658,58.7179076176479));
#19383=CARTESIAN_POINT('Ctrl Pts',(3.21041235565451,0.286695625514143,58.7210773041909));
#19384=CARTESIAN_POINT('Ctrl Pts',(3.20104688015028,0.375092387262804,58.7264463301134));
#19385=CARTESIAN_POINT('Ctrl Pts',(3.19668952831531,0.410574389751162,58.7286232146917));
#19386=CARTESIAN_POINT('Ctrl Pts',(3.18676008106815,0.481637134299323,58.7330302380956));
#19387=CARTESIAN_POINT('Ctrl Pts',(3.18118000159674,0.517211537622918,58.73526033297));
#19388=CARTESIAN_POINT('Ctrl Pts',(3.16564581402951,0.606450845601025,58.7409178973475));
#19389=CARTESIAN_POINT('Ctrl Pts',(3.15492264806733,0.659968603768021,58.7443689196773));
#19390=CARTESIAN_POINT('Ctrl Pts',(3.0904039427137,0.944287735587318,58.7630245002923));
#19391=CARTESIAN_POINT('Ctrl Pts',(3.012638488592,1.16886749148693,58.778978712579));
#19392=CARTESIAN_POINT('Ctrl Pts',(2.86589720070745,1.47776576619269,58.8020718155961));
#19393=CARTESIAN_POINT('Ctrl Pts',(2.8161933034815,1.57041895640225,58.809149752206));
#19394=CARTESIAN_POINT('Ctrl Pts',(2.73925132808562,1.69840443070662,58.819010996101));
#19395=CARTESIAN_POINT('Ctrl Pts',(2.71567342796502,1.73585530465207,58.8219070249988));
#19396=CARTESIAN_POINT('Ctrl Pts',(2.67209378292484,1.80201423519084,58.8270267075113));
#19397=CARTESIAN_POINT('Ctrl Pts',(2.65238186747647,1.83090446134634,58.8292636553493));
#19398=CARTESIAN_POINT('Ctrl Pts',(2.620137009386,1.87654920395239,58.8327928304405));
#19399=CARTESIAN_POINT('Ctrl Pts',(2.60790496625729,1.89351171276184,58.8341031935381));
#19400=CARTESIAN_POINT('Ctrl Pts',(2.58465020071729,1.92510686271911,58.8365399138185));
#19401=CARTESIAN_POINT('Ctrl Pts',(2.57366623696074,1.93976679802404,58.8376688721513));
#19402=CARTESIAN_POINT('Ctrl Pts',(2.54314933710594,1.97978112793534,58.8407481869553));
#19403=CARTESIAN_POINT('Ctrl Pts',(2.52336225329173,2.0049401436542,58.8426818712912));
#19404=CARTESIAN_POINT('Ctrl Pts',(2.42079999360231,2.13142254425649,58.8524144159525));
#19405=CARTESIAN_POINT('Ctrl Pts',(2.33227658365501,2.22794244886292,58.8598816318094));
#19406=CARTESIAN_POINT('Ctrl Pts',(2.10863837172773,2.44379763223764,58.8774036577988));
#19407=CARTESIAN_POINT('Ctrl Pts',(1.96891793083494,2.55770682443238,58.8873598692556));
#19408=CARTESIAN_POINT('Ctrl Pts',(1.7608040979732,2.7001677802958,58.9017692453151));
#19409=CARTESIAN_POINT('Ctrl Pts',(1.69983507276302,2.73895909531567,58.90594231409));
#19410=CARTESIAN_POINT('Ctrl Pts',(1.58686718293911,2.8056090446986,58.9136387510404));
#19411=CARTESIAN_POINT('Ctrl Pts',(1.53530869790419,2.83415174864578,58.9171384361721));
#19412=CARTESIAN_POINT('Ctrl Pts',(1.4502967543022,2.878213615928,58.922905928523));
#19413=CARTESIAN_POINT('Ctrl Pts',(1.41730736223012,2.89460082980786,58.925143267815));
#19414=CARTESIAN_POINT('Ctrl Pts',(1.35264234208755,2.9253521874344,58.9295311237942));
#19415=CARTESIAN_POINT('Ctrl Pts',(1.32100070407811,2.93977613376806,58.9316792036037));
#19416=CARTESIAN_POINT('Ctrl Pts',(1.25092893156231,2.97035888933485,58.9364410058048));
#19417=CARTESIAN_POINT('Ctrl Pts',(1.21240664442007,2.98628950270077,58.9390619602566));
#19418=CARTESIAN_POINT('Ctrl Pts',(1.07042996233498,3.04180303056521,58.9487370813451));
#19419=CARTESIAN_POINT('Ctrl Pts',(0.965271876809903,3.07678920455712,58.955936110015));
#19420=CARTESIAN_POINT('Ctrl Pts',(0.838364585865782,3.1118644117633,58.964647882717));
#19421=CARTESIAN_POINT('Ctrl Pts',(0.81814502216379,3.11724140811213,58.9660364571504));
#19422=CARTESIAN_POINT('Ctrl Pts',(0.606425175934186,3.17134235218727,58.98057932777));
#19423=CARTESIAN_POINT('Ctrl Pts',(0.410893209371642,3.20254979908285,58.9940719396457));
#19424=CARTESIAN_POINT('Ctrl Pts',(0.153388597667511,3.2196658143404,59.0112982136109));
#19425=CARTESIAN_POINT('Ctrl Pts',(0.0929324324061976,3.22197770424125,
59.0153009342391));
#19426=CARTESIAN_POINT('Ctrl Pts',(-0.0114722981714657,3.2230288239894,
59.0221058586023));
#19427=CARTESIAN_POINT('Ctrl Pts',(-0.0553956913796581,3.22257321959653,
59.0249358098143));
#19428=CARTESIAN_POINT('Ctrl Pts',(-0.121995253913166,3.22052020007587,
59.0291636161899));
#19429=CARTESIAN_POINT('Ctrl Pts',(-0.144684904973048,3.21958064813989,
59.0305928363602));
#19430=CARTESIAN_POINT('Ctrl Pts',(-0.18712917660364,3.21737345867217,59.0332431856965));
#19431=CARTESIAN_POINT('Ctrl Pts',(-0.206883956676711,3.21616360679244,
59.034467032317));
#19432=CARTESIAN_POINT('Ctrl Pts',(-0.25090510005703,3.21306030319763,59.0371743808418));
#19433=CARTESIAN_POINT('Ctrl Pts',(-0.275163111547384,3.21107384279669,
59.0386529471544));
#19434=CARTESIAN_POINT('Ctrl Pts',(-0.365898148618014,3.20260784299262,
59.0441411750631));
#19435=CARTESIAN_POINT('Ctrl Pts',(-0.432195005777373,3.19433673544487,
59.0480663330513));
#19436=CARTESIAN_POINT('Ctrl Pts',(-0.693620149646696,3.15343243308761,
59.0633727922369));
#19437=CARTESIAN_POINT('Ctrl Pts',(-0.88582981802671,3.10492519762998,59.0742680308405));
#19438=CARTESIAN_POINT('Ctrl Pts',(-1.16822794358344,3.00527703844516,59.0911344287984));
#19439=CARTESIAN_POINT('Ctrl Pts',(-1.26241005717512,2.96694549572378,59.0969092347154));
#19440=CARTESIAN_POINT('Ctrl Pts',(-1.42252883533251,2.89277212603626,59.1071465043538));
#19441=CARTESIAN_POINT('Ctrl Pts',(-1.48931755300562,2.85895975226926,59.1115499560623));
#19442=CARTESIAN_POINT('Ctrl Pts',(-1.58971711902455,2.80365835931714,59.1184151583117));
#19443=CARTESIAN_POINT('Ctrl Pts',(-1.62420901905247,2.78381852207022,59.1208197310163));
#19444=CARTESIAN_POINT('Ctrl Pts',(-1.68774326791549,2.74569070394599,59.1253405507286));
#19445=CARTESIAN_POINT('Ctrl Pts',(-1.71687812658293,2.72756743929242,59.1274506245945));
#19446=CARTESIAN_POINT('Ctrl Pts',(-1.78206279698645,2.68556126875977,59.1322587111041));
#19447=CARTESIAN_POINT('Ctrl Pts',(-1.81793183235876,2.6614114121675,59.1349663351169));
#19448=CARTESIAN_POINT('Ctrl Pts',(-1.93193576583333,2.58127488488144,59.1437788676825));
#19449=CARTESIAN_POINT('Ctrl Pts',(-2.00804961445334,2.52251652644894,59.1499858383815));
#19450=CARTESIAN_POINT('Ctrl Pts',(-2.19784622960557,2.36195797922543,59.1663176417798));
#19451=CARTESIAN_POINT('Ctrl Pts',(-2.30712753929267,2.25533352930772,59.1765917799252));
#19452=CARTESIAN_POINT('Ctrl Pts',(-2.51270917982429,2.02411316306989,59.1974927171383));
#19453=CARTESIAN_POINT('Ctrl Pts',(-2.60827955554223,1.89937527874125,59.208092588991));
#19454=CARTESIAN_POINT('Ctrl Pts',(-2.71595262172634,1.73529940296152,59.2208316499056));
#19455=CARTESIAN_POINT('Ctrl Pts',(-2.73691689645245,1.70204256057179,59.2233556851422));
#19456=CARTESIAN_POINT('Ctrl Pts',(-2.76854989788951,1.64976480029569,59.2272242952187));
#19457=CARTESIAN_POINT('Ctrl Pts',(-2.7796423029921,1.63100618146715,59.2285930901741));
#19458=CARTESIAN_POINT('Ctrl Pts',(-2.80063906359022,1.59466161282985,59.2312058931905));
#19459=CARTESIAN_POINT('Ctrl Pts',(-2.81056989382123,1.57709280511396,59.2324513482967));
#19460=CARTESIAN_POINT('Ctrl Pts',(-2.83547732451168,1.5320460674253,59.2356029189787));
#19461=CARTESIAN_POINT('Ctrl Pts',(-2.85022039138348,1.50444032662634,59.2374951572292));
#19462=CARTESIAN_POINT('Ctrl Pts',(-2.9197415106292,1.36957355175137,59.2465726321053));
#19463=CARTESIAN_POINT('Ctrl Pts',(-2.96888494376337,1.25950390291113,59.2534767143923));
#19464=CARTESIAN_POINT('Ctrl Pts',(-3.11044237894284,0.887784916053613,
59.275959742021));
#19465=CARTESIAN_POINT('Ctrl Pts',(-3.17526602581569,0.617005136844247,
59.2911396651945));
#19466=CARTESIAN_POINT('Ctrl Pts',(-3.21022110947204,0.288766173036444,
59.3106123424897));
#19467=CARTESIAN_POINT('Ctrl Pts',(-3.21452098042975,0.236135282172697,
59.3137622071998));
#19468=CARTESIAN_POINT('Ctrl Pts',(-3.21935478132504,0.151343617337449,
59.3188930054627));
#19469=CARTESIAN_POINT('Ctrl Pts',(-3.22070369453345,0.11923798067955,59.3208486068182));
#19470=CARTESIAN_POINT('Ctrl Pts',(-3.22253010664521,0.0516986523011541,
59.3249921676658));
#19471=CARTESIAN_POINT('Ctrl Pts',(-3.22290370253146,0.0162666845945092,
59.3271830733254));
#19472=CARTESIAN_POINT('Ctrl Pts',(-3.22238791594585,-0.0704737995444062,
59.3325914541781));
#19473=CARTESIAN_POINT('Ctrl Pts',(-3.2208574442024,-0.121767328821068,
59.335828199242));
#19474=CARTESIAN_POINT('Ctrl Pts',(-3.20712032331414,-0.377301517376942,
59.3521539036567));
#19475=CARTESIAN_POINT('Ctrl Pts',(-3.1767091700218,-0.580062455399293,
59.365791885938));
#19476=CARTESIAN_POINT('Ctrl Pts',(-3.08256721426357,-0.958217421897955,
59.3920923054007));
#19477=CARTESIAN_POINT('Ctrl Pts',(-3.02243315722774,-1.13371434719622,
59.4046654065589));
#19478=CARTESIAN_POINT('Ctrl Pts',(-2.93265848917949,-1.33678318485918,
59.4190411984297));
#19479=CARTESIAN_POINT('Ctrl Pts',(-2.91718316834908,-1.37022542796239,
59.4214019132187));
#19480=CARTESIAN_POINT('Ctrl Pts',(-2.89185638029371,-1.42258161000561,
59.425078818019));
#19481=CARTESIAN_POINT('Ctrl Pts',(-2.88238538007774,-1.44167483905053,
59.426415653761));
#19482=CARTESIAN_POINT('Ctrl Pts',(-2.86339215993269,-1.47902905396084,
59.4290209915457));
#19483=CARTESIAN_POINT('Ctrl Pts',(-2.8538830477831,-1.49729529171775,59.4302901016983));
#19484=CARTESIAN_POINT('Ctrl Pts',(-2.82857976978781,-1.54478391707973,
59.4335798930614));
#19485=CARTESIAN_POINT('Ctrl Pts',(-2.81250728646633,-1.57385635361129,
59.4355842605114));
#19486=CARTESIAN_POINT('Ctrl Pts',(-2.77546245002854,-1.6384838121772,59.440029870302));
#19487=CARTESIAN_POINT('Ctrl Pts',(-2.75425054015925,-1.67389523808841,
59.4424587868245));
#19488=CARTESIAN_POINT('Ctrl Pts',(-2.6829884315633,-1.78783696300309,59.4502834191538));
#19489=CARTESIAN_POINT('Ctrl Pts',(-2.63021234622076,-1.86461064868825,
59.4555710001201));
#19490=CARTESIAN_POINT('Ctrl Pts',(-2.41650882681915,-2.14832051555247,
59.4755791294502));
#19491=CARTESIAN_POINT('Ctrl Pts',(-2.23390724096757,-2.33761537859557,
59.4900236324999));
#19492=CARTESIAN_POINT('Ctrl Pts',(-1.99087765978373,-2.53478097948101,
59.5085210285756));
#19493=CARTESIAN_POINT('Ctrl Pts',(-1.95059670433833,-2.56590735306645,
59.5115624673259));
#19494=CARTESIAN_POINT('Ctrl Pts',(-1.88136348061117,-2.61683347962296,
59.5167606006669));
#19495=CARTESIAN_POINT('Ctrl Pts',(-1.85279384056996,-2.63713876040281,
59.5188975074895));
#19496=CARTESIAN_POINT('Ctrl Pts',(-1.79378185994841,-2.67764798155062,
59.5232981600596));
#19497=CARTESIAN_POINT('Ctrl Pts',(-1.76331584096983,-2.69780821145064,
59.5255631217287));
#19498=CARTESIAN_POINT('Ctrl Pts',(-1.68435682414545,-2.74814874305156,
59.5314187549751));
#19499=CARTESIAN_POINT('Ctrl Pts',(-1.63539393730862,-2.77756465969716,
59.5350363680787));
#19500=CARTESIAN_POINT('Ctrl Pts',(-1.4402809663901,-2.8878367470472,59.549407630889));
#19501=CARTESIAN_POINT('Ctrl Pts',(-1.28873492577402,-2.95857393868106,
59.5604920753131));
#19502=CARTESIAN_POINT('Ctrl Pts',(-0.938560002642515,-3.08999894691175,
59.5856742768592));
#19503=CARTESIAN_POINT('Ctrl Pts',(-0.73814310172579,-3.1439054014834,59.599808555615));
#19504=CARTESIAN_POINT('Ctrl Pts',(-0.519498516188417,-3.18063721291414,
59.6141969279335));
#19505=CARTESIAN_POINT('Ctrl Pts',(-0.505047975621658,-3.18296376521452,
59.6151429755576));
#19506=CARTESIAN_POINT('Ctrl Pts',(-0.490582094004581,-3.18519179509525,
59.6160848123881));
#19507=CARTESIAN_POINT('',(-3.22274929773161,-0.00212755034421634,59.5777091182932));
#19508=CARTESIAN_POINT('Ctrl Pts',(-0.490582094296224,-3.18519179505033,
59.8598970253053));
#19509=CARTESIAN_POINT('Ctrl Pts',(-0.588567220510107,-3.17010016116424,
59.8537889339454));
#19510=CARTESIAN_POINT('Ctrl Pts',(-0.685776785759724,-3.15049492155716,
59.8476808425855));
#19511=CARTESIAN_POINT('Ctrl Pts',(-0.781768325518016,-3.12649257918786,
59.8415727512256));
#19512=CARTESIAN_POINT('Ctrl Pts',(-0.877926813432343,-3.10244849202721,
59.8354540366942));
#19513=CARTESIAN_POINT('Ctrl Pts',(-0.972862618905612,-3.07399214979295,
59.8293353221628));
#19514=CARTESIAN_POINT('Ctrl Pts',(-1.06614928443358,-3.0412897372335,59.8232166076314));
#19515=CARTESIAN_POINT('Ctrl Pts',(-1.15916173008287,-3.00868345472172,
59.8171158793057));
#19516=CARTESIAN_POINT('Ctrl Pts',(-1.25053434997069,-2.97185627268983,
59.81101515098));
#19517=CARTESIAN_POINT('Ctrl Pts',(-1.33986848452895,-2.93101859541459,
59.8049144226543));
#19518=CARTESIAN_POINT('Ctrl Pts',(-1.43040172758154,-2.88963276478283,
59.7987318058636));
#19519=CARTESIAN_POINT('Ctrl Pts',(-1.5191708502785,-2.84397750535809,59.7925491890728));
#19520=CARTESIAN_POINT('Ctrl Pts',(-1.60574627620447,-2.79422555620614,
59.786366572282));
#19521=CARTESIAN_POINT('Ctrl Pts',(-1.69220561574934,-2.74454031794436,
59.7801922455759));
#19522=CARTESIAN_POINT('Ctrl Pts',(-1.77647673364627,-2.69076952301357,
59.7740179188698));
#19523=CARTESIAN_POINT('Ctrl Pts',(-1.85815124673768,-2.63313340086431,
59.7678435921637));
#19524=CARTESIAN_POINT('Ctrl Pts',(-1.93974013763877,-2.57555770063658,
59.7616757382158));
#19525=CARTESIAN_POINT('Ctrl Pts',(-2.01873748447073,-2.51412497820492,
59.7555078842679));
#19526=CARTESIAN_POINT('Ctrl Pts',(-2.09476151080866,-2.44910019707947,
59.74934003032));
#19527=CARTESIAN_POINT('Ctrl Pts',(-2.17073027706268,-2.38412268094423,
59.7431766596407));
#19528=CARTESIAN_POINT('Ctrl Pts',(-2.24372969248937,-2.31555857830692,
59.7370132889614));
#19529=CARTESIAN_POINT('Ctrl Pts',(-2.31340960483721,-2.24371423375326,
59.730849918282));
#19530=CARTESIAN_POINT('Ctrl Pts',(-2.38306332949095,-2.17189689034893,
59.7246888639728));
#19531=CARTESIAN_POINT('Ctrl Pts',(-2.44939972943618,-2.09680206519114,
59.7185278096636));
#19532=CARTESIAN_POINT('Ctrl Pts',(-2.51210483965493,-2.01877359728185,
59.7123667553544));
#19533=CARTESIAN_POINT('Ctrl Pts',(-2.57480299288723,-1.94075378645,59.7062063845998));
#19534=CARTESIAN_POINT('Ctrl Pts',(-2.63387038655929,-1.85980131735224,
59.7000460138453));
#19535=CARTESIAN_POINT('Ctrl Pts',(-2.68903339717869,-1.77629303645477,
59.6938856430907));
#19536=CARTESIAN_POINT('Ctrl Pts',(-2.74420489893484,-1.69277190128729,
59.6877243240821));
#19537=CARTESIAN_POINT('Ctrl Pts',(-2.79547058542601,-1.60669453391276,
59.6815630050734));
#19538=CARTESIAN_POINT('Ctrl Pts',(-2.84260075887082,-1.5184658337174,59.6754016860648));
#19539=CARTESIAN_POINT('Ctrl Pts',(-2.88977971480695,-1.4301458116472,59.6692339897299));
#19540=CARTESIAN_POINT('Ctrl Pts',(-2.93281440624732,-1.33967039270124,
59.6630662933951));
#19541=CARTESIAN_POINT('Ctrl Pts',(-2.97152169936721,-1.24746797661899,
59.6568985970602));
#19542=CARTESIAN_POINT('Ctrl Pts',(-3.01025038863967,-1.15521459399263,
59.6507274914202));
#19543=CARTESIAN_POINT('Ctrl Pts',(-3.04464676656595,-1.06123271913011,
59.6445563857803));
#19544=CARTESIAN_POINT('Ctrl Pts',(-3.07457705306434,-0.965967653325046,
59.6383852801403));
#19545=CARTESIAN_POINT('Ctrl Pts',(-3.10455510623962,-0.870550551032845,
59.6322043258406));
#19546=CARTESIAN_POINT('Ctrl Pts',(-3.13005272184961,-0.773846585983105,
59.6260233715408));
#19547=CARTESIAN_POINT('Ctrl Pts',(-3.15098685273959,-0.676313105271749,
59.6198424172411));
#19548=CARTESIAN_POINT('Ctrl Pts',(-3.16502954150311,-0.610887302746178,
59.6156962113179));
#19549=CARTESIAN_POINT('Ctrl Pts',(-3.17701983363642,-0.545088434709207,
59.6115500053947));
#19550=CARTESIAN_POINT('Ctrl Pts',(-3.18694576623428,-0.479055576714712,
59.6074037994715));
#19551=CARTESIAN_POINT('Ctrl Pts',(-3.21064192036897,-0.321415499516386,
59.597505572412));
#19552=CARTESIAN_POINT('Ctrl Pts',(-3.22264376531188,-0.161984886987291,
59.5876073453526));
#19553=CARTESIAN_POINT('Ctrl Pts',(-3.22274929773161,-0.00212755034421634,
59.5777091182932));
#19554=CARTESIAN_POINT('Ctrl Pts',(-3.22515705657206,-0.00210809394305351,
59.5777078161216));
#19555=CARTESIAN_POINT('Ctrl Pts',(-3.21756318232272,0.901980015450162,
59.5217696028439));
#19556=CARTESIAN_POINT('Ctrl Pts',(-2.35196096173306,2.88200781430396,59.3999945151719));
#19557=CARTESIAN_POINT('Ctrl Pts',(0.998193681065493,3.67000140801024,59.2123825531058));
#19558=CARTESIAN_POINT('Ctrl Pts',(3.61883085014894,1.16896682075721,59.0148719299228));
#19559=CARTESIAN_POINT('Ctrl Pts',(2.95640798566869,-2.39226680571159,58.81736130674));
#19560=CARTESIAN_POINT('Ctrl Pts',(0.669413081115714,-3.34327461681512,
58.6823193174151));
#19561=CARTESIAN_POINT('Ctrl Pts',(-0.437675410847414,-3.19850339953065,
58.6131142024843));
#19562=CARTESIAN_POINT('Ctrl Pts',(-0.491343452670647,-3.19000126486617,
58.6097459619479));
#19563=CARTESIAN_POINT('Origin',(-9.35406549764863E-15,0.,41.4527091182931));
#19564=CARTESIAN_POINT('',(-0.49058180811571,-3.18519183912774,57.1123311812828));
#19565=CARTESIAN_POINT('',(-0.490582240097165,-3.18519177259412,57.3619600447814));
#19566=CARTESIAN_POINT('',(-0.490582094296226,-3.18519179505033,41.4527091182931));
#19567=CARTESIAN_POINT('',(-3.22274878421801,0.00279934303327976,58.081859847365));
#19568=CARTESIAN_POINT('Ctrl Pts',(-0.490581808115708,-3.18519183912774,
57.1123311812828));
#19569=CARTESIAN_POINT('Ctrl Pts',(-0.363519266685327,-3.20476195435689,
57.1195896121718));
#19570=CARTESIAN_POINT('Ctrl Pts',(-0.235300550620664,-3.21672691832773,
57.126950618447));
#19571=CARTESIAN_POINT('Ctrl Pts',(-0.0531215777745777,-3.22275646010443,
57.1376960522343));
#19572=CARTESIAN_POINT('Ctrl Pts',(0.000394523536829932,-3.22319413942321,
57.140886515961));
#19573=CARTESIAN_POINT('Ctrl Pts',(0.086128815411882,-3.22176019097727,
57.1460645706055));
#19574=CARTESIAN_POINT('Ctrl Pts',(0.118352235991067,-3.22073742078687,
57.148025852026));
#19575=CARTESIAN_POINT('Ctrl Pts',(0.185817376770669,-3.2175822738534,57.1521664065113));
#19576=CARTESIAN_POINT('Ctrl Pts',(0.221050091166339,-3.21535386658781,
57.1543483955745));
#19577=CARTESIAN_POINT('Ctrl Pts',(0.306693210253217,-3.2085228313182,57.1597030759785));
#19578=CARTESIAN_POINT('Ctrl Pts',(0.35704415803387,-3.20331055208824,57.1628941814196));
#19579=CARTESIAN_POINT('Ctrl Pts',(0.588399476729501,-3.17383860920283,
57.1777633587442));
#19580=CARTESIAN_POINT('Ctrl Pts',(0.767234648021058,-3.13541050638952,
57.1898690476116));
#19581=CARTESIAN_POINT('Ctrl Pts',(1.14335297295845,-3.02047431222032,57.2163549205064));
#19582=CARTESIAN_POINT('Ctrl Pts',(1.33835832866908,-2.939273283835,57.2307398731188));
#19583=CARTESIAN_POINT('Ctrl Pts',(1.55560851429715,-2.82267297650291,57.2466884357191));
#19584=CARTESIAN_POINT('Ctrl Pts',(1.58688632482501,-2.80520812392022,57.2489814973636));
#19585=CARTESIAN_POINT('Ctrl Pts',(1.63610451452224,-2.77663901318277,57.2525772636646));
#19586=CARTESIAN_POINT('Ctrl Pts',(1.65423740809246,-2.76587433689308,57.2538992418942));
#19587=CARTESIAN_POINT('Ctrl Pts',(1.68994586731178,-2.74419904129099,57.2564950470604));
#19588=CARTESIAN_POINT('Ctrl Pts',(1.70752451203387,-2.73329572064327,57.2577691746616));
#19589=CARTESIAN_POINT('Ctrl Pts',(1.75361087552491,-2.7040920738317,57.2611029858357));
#19590=CARTESIAN_POINT('Ctrl Pts',(1.78193797792735,-2.68550968985088,57.2631453791153));
#19591=CARTESIAN_POINT('Ctrl Pts',(1.94734533430325,-2.57323370755409,57.2750638598141));
#19592=CARTESIAN_POINT('Ctrl Pts',(2.07732683492534,-2.4694961026689,57.2844072039961));
#19593=CARTESIAN_POINT('Ctrl Pts',(2.35823966240032,-2.20735460217788,57.3059475879948));
#19594=CARTESIAN_POINT('Ctrl Pts',(2.50219601326392,-2.04272224416803,57.3180941750521));
#19595=CARTESIAN_POINT('Ctrl Pts',(2.66117883123958,-1.81863976646521,57.3342465664888));
#19596=CARTESIAN_POINT('Ctrl Pts',(2.69271724329053,-1.77160849232256,57.3376146691767));
#19597=CARTESIAN_POINT('Ctrl Pts',(2.74246304998617,-1.69302633623517,57.3432223880811));
#19598=CARTESIAN_POINT('Ctrl Pts',(2.76140411902098,-1.6619533330701,57.3454348191831));
#19599=CARTESIAN_POINT('Ctrl Pts',(2.79774321602195,-1.60000191844197,57.3498397290469));
#19600=CARTESIAN_POINT('Ctrl Pts',(2.81516609456666,-1.56914401621594,57.3520309055797));
#19601=CARTESIAN_POINT('Ctrl Pts',(2.85660363979631,-1.49284114252743,57.3574449397183));
#19602=CARTESIAN_POINT('Ctrl Pts',(2.88004607694429,-1.44709818075665,57.3606871970129));
#19603=CARTESIAN_POINT('Ctrl Pts',(2.99206482870654,-1.21500392724573,57.3771299233356));
#19604=CARTESIAN_POINT('Ctrl Pts',(3.06368188208961,-1.02103655511887,57.3908900278049));
#19605=CARTESIAN_POINT('Ctrl Pts',(3.16298229078933,-0.644392258938267,
57.417183776433));
#19606=CARTESIAN_POINT('Ctrl Pts',(3.19450366314214,-0.463523224311926,
57.4296237777371));
#19607=CARTESIAN_POINT('Ctrl Pts',(3.21369957739114,-0.244163597585218,
57.4438832688859));
#19608=CARTESIAN_POINT('Ctrl Pts',(3.21628613982045,-0.207327201106171,
57.446249287105));
#19609=CARTESIAN_POINT('Ctrl Pts',(3.21936648206036,-0.149168692678552,
57.4499316091332));
#19610=CARTESIAN_POINT('Ctrl Pts',(3.22028264788585,-0.127873265124269,
57.4512686983814));
#19611=CARTESIAN_POINT('Ctrl Pts',(3.22166541011702,-0.0860803088763244,
57.4538686960056));
#19612=CARTESIAN_POINT('Ctrl Pts',(3.22214781228551,-0.0655846227731079,
57.4551322850543));
#19613=CARTESIAN_POINT('Ctrl Pts',(3.22289569486623,-0.0121303332849647,
57.4584010521021));
#19614=CARTESIAN_POINT('Ctrl Pts',(3.22285123074699,0.0208312194294717,
57.4603901734727));
#19615=CARTESIAN_POINT('Ctrl Pts',(3.21946010656653,0.223985875842655,57.4725180470774));
#19616=CARTESIAN_POINT('Ctrl Pts',(3.20313865414242,0.393711827527747,57.4820887489451));
#19617=CARTESIAN_POINT('Ctrl Pts',(3.13598090366949,0.77336166160849,57.5036993069403));
#19618=CARTESIAN_POINT('Ctrl Pts',(3.07733795816236,0.981043346933699,57.5156948280978));
#19619=CARTESIAN_POINT('Ctrl Pts',(2.97759373200925,1.23421434138993,57.5316888541461));
#19620=CARTESIAN_POINT('Ctrl Pts',(2.9553601140516,1.2865440115326,57.5350700945385));
#19621=CARTESIAN_POINT('Ctrl Pts',(2.91662626969095,1.37139932984,57.5406936963356));
#19622=CARTESIAN_POINT('Ctrl Pts',(2.90093697063014,1.40428253743463,57.5429085490009));
#19623=CARTESIAN_POINT('Ctrl Pts',(2.86890856587276,1.4685825459715,57.5473138388743));
#19624=CARTESIAN_POINT('Ctrl Pts',(2.85260244524963,1.50001006172084,57.5495028966313));
#19625=CARTESIAN_POINT('Ctrl Pts',(2.81144881726522,1.57622849126425,57.5549033243697));
#19626=CARTESIAN_POINT('Ctrl Pts',(2.78604558587402,1.62070670556981,57.5581338672329));
#19627=CARTESIAN_POINT('Ctrl Pts',(2.65368110125754,1.84014761399111,57.5744817918008));
#19628=CARTESIAN_POINT('Ctrl Pts',(2.53126682652806,2.00520100772327,57.5881517712879));
#19629=CARTESIAN_POINT('Ctrl Pts',(2.27013744495275,2.2949600152189,57.6144797810067));
#19630=CARTESIAN_POINT('Ctrl Pts',(2.13462777313359,2.42151583033966,57.6270474072483));
#19631=CARTESIAN_POINT('Ctrl Pts',(1.96001051197897,2.55848265217056,57.6414175725839));
#19632=CARTESIAN_POINT('Ctrl Pts',(1.93063529101231,2.5807212800703,57.6437780771931));
#19633=CARTESIAN_POINT('Ctrl Pts',(1.88368612655658,2.61501389902058,57.6474538659723));
#19634=CARTESIAN_POINT('Ctrl Pts',(1.86636377332607,2.62740507734548,57.6487898198236));
#19635=CARTESIAN_POINT('Ctrl Pts',(1.83211736628624,2.65139290376272,57.6513894626546));
#19636=CARTESIAN_POINT('Ctrl Pts',(1.81520314212203,2.66300130681889,57.6526538040951));
#19637=CARTESIAN_POINT('Ctrl Pts',(1.77077340573991,2.69287387244312,57.6559272391761));
#19638=CARTESIAN_POINT('Ctrl Pts',(1.74308512396861,2.71087856409127,57.6579201886513));
#19639=CARTESIAN_POINT('Ctrl Pts',(1.68043072432765,2.75026350591833,57.6623371249689));
#19640=CARTESIAN_POINT('Ctrl Pts',(1.64532336772238,2.77140904136289,57.6647489552529));
#19641=CARTESIAN_POINT('Ctrl Pts',(1.53007546459174,2.83786192085284,57.6724952171617));
#19642=CARTESIAN_POINT('Ctrl Pts',(1.44839199149357,2.88040860677375,57.6777232160301));
#19643=CARTESIAN_POINT('Ctrl Pts',(1.13351642074583,3.02763176556984,57.6973004500824));
#19644=CARTESIAN_POINT('Ctrl Pts',(0.89000703225663,3.10794045130935,57.7113713746647));
#19645=CARTESIAN_POINT('Ctrl Pts',(0.585365619488878,3.1696251382868,57.729665176306));
#19646=CARTESIAN_POINT('Ctrl Pts',(0.53088770096092,3.17920338149255,57.7329582698494));
#19647=CARTESIAN_POINT('Ctrl Pts',(0.440445945405425,3.19271534501132,57.7384754743614));
#19648=CARTESIAN_POINT('Ctrl Pts',(0.404613181634699,3.19745397395242,57.7406742230626));
#19649=CARTESIAN_POINT('Ctrl Pts',(0.333315922573735,3.20566488727956,57.745078103364));
#19650=CARTESIAN_POINT('Ctrl Pts',(0.297858486792379,3.20915363215339,57.7472823869861));
#19651=CARTESIAN_POINT('Ctrl Pts',(0.210041500496304,3.21632627861556,57.7527795916799));
#19652=CARTESIAN_POINT('Ctrl Pts',(0.157637461614142,3.2193201271046,57.7560933098251));
#19653=CARTESIAN_POINT('Ctrl Pts',(-0.0917388816373725,3.22746375842088,
57.7720288896367));
#19654=CARTESIAN_POINT('Ctrl Pts',(-0.288810206972034,3.21582118715856,
57.7851517432284));
#19655=CARTESIAN_POINT('Ctrl Pts',(-0.672175759190451,3.1576405591133,57.8113142293623));
#19656=CARTESIAN_POINT('Ctrl Pts',(-0.857891958734288,3.11232146478025,
57.8242851999409));
#19657=CARTESIAN_POINT('Ctrl Pts',(-1.07313730631409,3.03905105567359,57.8390041155607));
#19658=CARTESIAN_POINT('Ctrl Pts',(-1.10755602583907,3.0266772053551,57.8413468780503));
#19659=CARTESIAN_POINT('Ctrl Pts',(-1.16162207360763,3.0061940929379,57.8450016315258));
#19660=CARTESIAN_POINT('Ctrl Pts',(-1.18141165373373,2.99847216590604,57.8463339214628));
#19661=CARTESIAN_POINT('Ctrl Pts',(-1.22019903013725,2.98289363506496,57.8489324080083));
#19662=CARTESIAN_POINT('Ctrl Pts',(-1.23920062974529,2.97504990648184,57.8501991662501));
#19663=CARTESIAN_POINT('Ctrl Pts',(-1.28872644456465,2.95404916140932,57.8534877198561));
#19664=CARTESIAN_POINT('Ctrl Pts',(-1.31912538154011,2.94060040117383,57.8554930848966));
#19665=CARTESIAN_POINT('Ctrl Pts',(-1.38684799971036,2.90937770132362,57.8599426936834));
#19666=CARTESIAN_POINT('Ctrl Pts',(-1.4240491136981,2.89135096434638,57.8623744997194));
#19667=CARTESIAN_POINT('Ctrl Pts',(-1.54415575708393,2.83026958342802,57.8702172436427));
#19668=CARTESIAN_POINT('Ctrl Pts',(-1.62554138035429,2.784323991421,57.8755188768522));
#19669=CARTESIAN_POINT('Ctrl Pts',(-1.9278482624066,2.59587914200526,57.8955744331124));
#19670=CARTESIAN_POINT('Ctrl Pts',(-2.13301448771868,2.43010860565412,57.9100503415682));
#19671=CARTESIAN_POINT('Ctrl Pts',(-2.35119945571632,2.20467075676006,57.928590028529));
#19672=CARTESIAN_POINT('Ctrl Pts',(-2.3857487111276,2.16723664813066,57.9316330520963));
#19673=CARTESIAN_POINT('Ctrl Pts',(-2.44251976480121,2.10272206840221,57.9368299593646));
#19674=CARTESIAN_POINT('Ctrl Pts',(-2.46521407632804,2.07606895539098,57.9389639148773));
#19675=CARTESIAN_POINT('Ctrl Pts',(-2.51062549333277,2.02094127610624,57.9433545662086));
#19676=CARTESIAN_POINT('Ctrl Pts',(-2.5333029291489,1.99244074097,57.94561241152));
#19677=CARTESIAN_POINT('Ctrl Pts',(-2.59008993137165,1.91853492560334,57.9514399116409));
#19678=CARTESIAN_POINT('Ctrl Pts',(-2.62349007300798,1.87260281541914,57.9550361453516));
#19679=CARTESIAN_POINT('Ctrl Pts',(-2.74910266747708,1.68989857125249,57.9692504537943));
#19680=CARTESIAN_POINT('Ctrl Pts',(-2.83196379421096,1.54702658207734,57.9801910008034));
#19681=CARTESIAN_POINT('Ctrl Pts',(-2.99616117652605,1.20611534976638,58.0056587850009));
#19682=CARTESIAN_POINT('Ctrl Pts',(-3.06946401062656,1.00503504499575,58.0202444199064));
#19683=CARTESIAN_POINT('Ctrl Pts',(-3.13145700286321,0.762527647538431,
58.0364515086102));
#19684=CARTESIAN_POINT('Ctrl Pts',(-3.13995907753847,0.726724589054719,
58.0388090374126));
#19685=CARTESIAN_POINT('Ctrl Pts',(-3.15240936265674,0.669989495848835,
58.0424812889327));
#19686=CARTESIAN_POINT('Ctrl Pts',(-3.15676623937361,0.649151510502292,
58.0438166193007));
#19687=CARTESIAN_POINT('Ctrl Pts',(-3.16491685405933,0.60814467847215,58.0464160269189));
#19688=CARTESIAN_POINT('Ctrl Pts',(-3.16872500682859,0.587980023328616,
58.0476807417008));
#19689=CARTESIAN_POINT('Ctrl Pts',(-3.17613289852994,0.54659012512587,58.0502515363195));
#19690=CARTESIAN_POINT('Ctrl Pts',(-3.17971312438338,0.525362213561324,
58.051556560361));
#19691=CARTESIAN_POINT('Ctrl Pts',(-3.19095758302043,0.454360310408386,
58.0558813662784));
#19692=CARTESIAN_POINT('Ctrl Pts',(-3.19766820145649,0.404440628147002,
58.0588563528042));
#19693=CARTESIAN_POINT('Ctrl Pts',(-3.21612230502583,0.23763649453959,58.0686390841135));
#19694=CARTESIAN_POINT('Ctrl Pts',(-3.22264674940602,0.120267106854988,
58.0752674424239));
#19695=CARTESIAN_POINT('Ctrl Pts',(-3.22274878421801,0.00279934303327976,
58.081859847365));
#19696=CARTESIAN_POINT('Ctrl Pts',(-3.22274878256121,0.00280124978110204,
58.0818597403565));
#19697=CARTESIAN_POINT('Ctrl Pts',(-3.22295790297624,-0.237785136880605,
58.0953616829093));
#19698=CARTESIAN_POINT('Ctrl Pts',(-3.19622788100395,-0.477625984509487,
58.1087087916921));
#19699=CARTESIAN_POINT('Ctrl Pts',(-3.13170233469332,-0.762362747975631,
58.1259544749398));
#19700=CARTESIAN_POINT('Ctrl Pts',(-3.11915318526195,-0.812181903703197,
58.1290223747661));
#19701=CARTESIAN_POINT('Ctrl Pts',(-3.09594587134366,-0.895819233599449,
58.134270033571));
#19702=CARTESIAN_POINT('Ctrl Pts',(-3.08591040996868,-0.929800906142302,
58.1364296532173));
#19703=CARTESIAN_POINT('Ctrl Pts',(-3.0644347111692,-0.998339668287042,
58.1408447584817));
#19704=CARTESIAN_POINT('Ctrl Pts',(-3.05296521092551,-1.03288210431023,
58.1431009286621));
#19705=CARTESIAN_POINT('Ctrl Pts',(-3.02215318343816,-1.12067707895704,
58.1489181680934));
#19706=CARTESIAN_POINT('Ctrl Pts',(-3.00198759552633,-1.17362550002979,
58.1525056297787));
#19707=CARTESIAN_POINT('Ctrl Pts',(-2.89758663148219,-1.42742439535898,
58.1700974239904));
#19708=CARTESIAN_POINT('Ctrl Pts',(-2.79454360409339,-1.61989141685892,
58.1847130849878));
#19709=CARTESIAN_POINT('Ctrl Pts',(-2.57906900765981,-1.93977628476205,
58.2107663277831));
#19710=CARTESIAN_POINT('Ctrl Pts',(-2.47447761883421,-2.0715450545229,58.2221108682565));
#19711=CARTESIAN_POINT('Ctrl Pts',(-2.33757865467796,-2.21876896399696,
58.235074729393));
#19712=CARTESIAN_POINT('Ctrl Pts',(-2.31470281759417,-2.24262362977957,
58.2371847270472));
#19713=CARTESIAN_POINT('Ctrl Pts',(-2.27703559774215,-2.2807120456572,58.2405631615659));
#19714=CARTESIAN_POINT('Ctrl Pts',(-2.2624685004369,-2.29516337260248,58.2418472562922));
#19715=CARTESIAN_POINT('Ctrl Pts',(-2.23250540864576,-2.32432582029433,
58.2444413378016));
#19716=CARTESIAN_POINT('Ctrl Pts',(-2.21709980732378,-2.33902531445437,
58.2457505230534));
#19717=CARTESIAN_POINT('Ctrl Pts',(-2.17466456586406,-2.37871957031481,
58.2492940767393));
#19718=CARTESIAN_POINT('Ctrl Pts',(-2.14734977241055,-2.4034063285044,58.2515070328352));
#19719=CARTESIAN_POINT('Ctrl Pts',(-1.97956498306949,-2.5499034445019,58.2647386416641));
#19720=CARTESIAN_POINT('Ctrl Pts',(-1.8291779708738,-2.65985118417592,58.2751102861338));
#19721=CARTESIAN_POINT('Ctrl Pts',(-1.49562741863346,-2.86196610976069,
58.2969567991984));
#19722=CARTESIAN_POINT('Ctrl Pts',(-1.31149223152743,-2.95088606072196,
58.3084073852797));
#19723=CARTESIAN_POINT('Ctrl Pts',(-1.07210638021965,-3.03962760092729,
58.3234893452765));
#19724=CARTESIAN_POINT('Ctrl Pts',(-1.02359959563135,-3.05630356440855,
58.326552552832));
#19725=CARTESIAN_POINT('Ctrl Pts',(-0.940958123590885,-3.08252653125341,
58.3317947104971));
#19726=CARTESIAN_POINT('Ctrl Pts',(-0.907025579250325,-3.09268111043141,
58.3339536286457));
#19727=CARTESIAN_POINT('Ctrl Pts',(-0.837877438667938,-3.11213836407604,
58.3383694703585));
#19728=CARTESIAN_POINT('Ctrl Pts',(-0.802657813982536,-3.12140738465124,
58.3406271149749));
#19729=CARTESIAN_POINT('Ctrl Pts',(-0.712158911981906,-3.14359178348112,
58.3464529982583));
#19730=CARTESIAN_POINT('Ctrl Pts',(-0.656683589866342,-3.15564662703973,
58.350047782547));
#19731=CARTESIAN_POINT('Ctrl Pts',(-0.564240146069718,-3.17319154966375,
58.3560799619886));
#19732=CARTESIAN_POINT('Ctrl Pts',(-0.527454640627873,-3.17951270074406,
58.3584911188382));
#19733=CARTESIAN_POINT('Ctrl Pts',(-0.490581924382687,-3.18519182122035,
58.3609184893942));
#19734=CARTESIAN_POINT('',(-3.21795389890993,-0.00035016928829556,58.3278759108383));
#19735=CARTESIAN_POINT('Ctrl Pts',(-0.491343452670647,-3.19000126486617,
58.6097459619479));
#19736=CARTESIAN_POINT('Ctrl Pts',(-1.48669079152002,-3.03231753307098,
58.54727732809));
#19737=CARTESIAN_POINT('Ctrl Pts',(-2.87365562611969,-2.04127453831248,
58.4532651482571));
#19738=CARTESIAN_POINT('Ctrl Pts',(-3.218177270761,-0.513265825290757,58.3592529684242));
#19739=CARTESIAN_POINT('Ctrl Pts',(-3.21766489697672,-0.000360507783602748,
58.3277094224493));
#19740=CARTESIAN_POINT('Ctrl Pts',(-3.22274999505125,-0.000178598057266107,
58.3306388484816));
#19741=CARTESIAN_POINT('Ctrl Pts',(-3.22275152166445,0.0273686931957166,
58.3289650202219));
#19742=CARTESIAN_POINT('Ctrl Pts',(-3.22239984723638,0.0549143201914142,
58.3272804884336));
#19743=CARTESIAN_POINT('Ctrl Pts',(-3.22079629405421,0.117571233435313,
58.3234225393163));
#19744=CARTESIAN_POINT('Ctrl Pts',(-3.21932332163406,0.152672718248279,
58.3212424896283));
#19745=CARTESIAN_POINT('Ctrl Pts',(-3.21401069872221,0.243713480325951,
58.3155367566181));
#19746=CARTESIAN_POINT('Ctrl Pts',(-3.20928464604641,0.299587168385481,
58.3119843242949));
#19747=CARTESIAN_POINT('Ctrl Pts',(-3.17931917787674,0.569727177749854,
58.294554344316));
#19748=CARTESIAN_POINT('Ctrl Pts',(-3.13406741837616,0.78118830237778,58.2800786983285));
#19749=CARTESIAN_POINT('Ctrl Pts',(-3.01625659151334,1.14757963909402,58.254080626764));
#19750=CARTESIAN_POINT('Ctrl Pts',(-2.95185826318816,1.30433323055823,58.242649922579));
#19751=CARTESIAN_POINT('Ctrl Pts',(-2.86054366726118,1.48475457999423,58.2296109801442));
#19752=CARTESIAN_POINT('Ctrl Pts',(-2.84519200336798,1.51396462788519,58.2275044157394));
#19753=CARTESIAN_POINT('Ctrl Pts',(-2.81957559134375,1.56093933224634,58.2241300538921));
#19754=CARTESIAN_POINT('Ctrl Pts',(-2.80958537046108,1.57885028879635,58.2228466634055));
#19755=CARTESIAN_POINT('Ctrl Pts',(-2.78887008968411,1.6151702717317,58.2202526387115));
#19756=CARTESIAN_POINT('Ctrl Pts',(-2.77813221753765,1.63357057532253,58.2189428275464));
#19757=CARTESIAN_POINT('Ctrl Pts',(-2.74831278439676,1.68352427672631,58.215395117694));
#19758=CARTESIAN_POINT('Ctrl Pts',(-2.72887036732328,1.71485973987912,58.2131787225866));
#19759=CARTESIAN_POINT('Ctrl Pts',(-2.60908685154661,1.90071743809104,58.2000447344578));
#19760=CARTESIAN_POINT('Ctrl Pts',(-2.4961729413212,2.04675268544039,58.1897617202013));
#19761=CARTESIAN_POINT('Ctrl Pts',(-2.23210266184536,2.33369686681867,58.1679184331134));
#19762=CARTESIAN_POINT('Ctrl Pts',(-2.07866626243933,2.47134758087012,58.1563815547593));
#19763=CARTESIAN_POINT('Ctrl Pts',(-1.87191063449352,2.62387055738965,58.1412036805653));
#19764=CARTESIAN_POINT('Ctrl Pts',(-1.82993408336617,2.65331621627637,58.1381415669522));
#19765=CARTESIAN_POINT('Ctrl Pts',(-1.75780676175894,2.70138612694307,58.1329008464759));
#19766=CARTESIAN_POINT('Ctrl Pts',(-1.72801808305598,2.72053762503069,58.1307422522321));
#19767=CARTESIAN_POINT('Ctrl Pts',(-1.66696737707833,2.75838060668851,58.1263267214002));
#19768=CARTESIAN_POINT('Ctrl Pts',(-1.6356920612514,2.77704071202683,58.1240690578455));
#19769=CARTESIAN_POINT('Ctrl Pts',(-1.55486590233354,2.82342575527607,58.1182423863547));
#19770=CARTESIAN_POINT('Ctrl Pts',(-1.50488806505103,2.85037756022782,58.1146468106689));
#19771=CARTESIAN_POINT('Ctrl Pts',(-1.26122400666847,2.97358463703967,58.0971423012683));
#19772=CARTESIAN_POINT('Ctrl Pts',(-1.05891428376394,3.05148588624235,58.0826320773377));
#19773=CARTESIAN_POINT('Ctrl Pts',(-0.687068309131056,3.15320719913749,
58.0565907867791));
#19774=CARTESIAN_POINT('Ctrl Pts',(-0.520492782642464,3.18494510044275,
58.0451525613443));
#19775=CARTESIAN_POINT('Ctrl Pts',(-0.319361332270748,3.20705724999789,
58.0321048781007));
#19776=CARTESIAN_POINT('Ctrl Pts',(-0.286484335774406,3.21016117764605,
58.0299966875096));
#19777=CARTESIAN_POINT('Ctrl Pts',(-0.233115856756237,3.21437323459194,
58.0266204376985));
#19778=CARTESIAN_POINT('Ctrl Pts',(-0.212651889309117,3.21579189966969,
58.0253367533369));
#19779=CARTESIAN_POINT('Ctrl Pts',(-0.17091425004314,3.21828518122513,58.0227427044638));
#19780=CARTESIAN_POINT('Ctrl Pts',(-0.149640894194258,3.21934447522593,
58.0214331534443));
#19781=CARTESIAN_POINT('Ctrl Pts',(-0.0915432161865209,3.22166026724364,
58.0178874059432));
#19782=CARTESIAN_POINT('Ctrl Pts',(-0.0547043013658262,3.22249635138902,
58.0156726675859));
#19783=CARTESIAN_POINT('Ctrl Pts',(0.16717426609087,3.22372581202411,58.0024925420027));
#19784=CARTESIAN_POINT('Ctrl Pts',(0.351971713844922,3.2088138540784,57.9921675813208));
#19785=CARTESIAN_POINT('Ctrl Pts',(0.736428993599204,3.14415729803788,57.9703299018682));
#19786=CARTESIAN_POINT('Ctrl Pts',(0.934656032977894,3.09102893572924,57.9588410105805));
#19787=CARTESIAN_POINT('Ctrl Pts',(1.17459898318525,3.00151144521947,57.9437130510065));
#19788=CARTESIAN_POINT('Ctrl Pts',(1.22226592145437,2.98241836605535,57.9406466737853));
#19789=CARTESIAN_POINT('Ctrl Pts',(1.30201901417135,2.94824002571026,57.9354006893267));
#19790=CARTESIAN_POINT('Ctrl Pts',(1.33435005684172,2.93374888736945,57.9332411843586));
#19791=CARTESIAN_POINT('Ctrl Pts',(1.39940641215535,2.9032920391361,57.9288255043921));
#19792=CARTESIAN_POINT('Ctrl Pts',(1.43211309689951,2.88729888938893,57.9265686312074));
#19793=CARTESIAN_POINT('Ctrl Pts',(1.51504573119677,2.84499008861874,57.9207477453517));
#19794=CARTESIAN_POINT('Ctrl Pts',(1.56485920046809,2.81789765813526,57.9171572797799));
#19795=CARTESIAN_POINT('Ctrl Pts',(1.80195888149963,2.68071848168018,57.8995974803984));
#19796=CARTESIAN_POINT('Ctrl Pts',(1.97848079589825,2.55321264091338,57.8850205591927));
#19797=CARTESIAN_POINT('Ctrl Pts',(2.26502172379285,2.29856618809587,57.8591260603297));
#19798=CARTESIAN_POINT('Ctrl Pts',(2.38051765674133,2.17873233430675,57.8479016010264));
#19799=CARTESIAN_POINT('Ctrl Pts',(2.50802674302002,2.02412684917581,57.8349615700869));
#19800=CARTESIAN_POINT('Ctrl Pts',(2.52937054621828,1.99739142401738,57.8327750653107));
#19801=CARTESIAN_POINT('Ctrl Pts',(2.56297379075501,1.95389703319851,57.8293058696407));
#19802=CARTESIAN_POINT('Ctrl Pts',(2.57550354005013,1.93735124506997,57.828006037752));
#19803=CARTESIAN_POINT('Ctrl Pts',(2.60039596799797,1.903811937988,57.8254128785718));
#19804=CARTESIAN_POINT('Ctrl Pts',(2.61275399041164,1.88681629418159,57.8241198574134));
#19805=CARTESIAN_POINT('Ctrl Pts',(2.64551751752937,1.84081830226653,57.8206729010836));
#19806=CARTESIAN_POINT('Ctrl Pts',(2.6656126140456,1.81159724589741,57.8185384448015));
#19807=CARTESIAN_POINT('Ctrl Pts',(2.79692150756155,1.61373875257659,57.8044092364315));
#19808=CARTESIAN_POINT('Ctrl Pts',(2.89256221463683,1.43527892424226,57.7931948972296));
#19809=CARTESIAN_POINT('Ctrl Pts',(3.02044469736014,1.13110286277834,57.7747045425397));
#19810=CARTESIAN_POINT('Ctrl Pts',(3.06295355279475,1.0103429281048,57.7675143048786));
#19811=CARTESIAN_POINT('Ctrl Pts',(3.11494092598975,0.828836170490921,57.7566352669263));
#19812=CARTESIAN_POINT('Ctrl Pts',(3.13004608136707,0.769829393781804,57.7530887388334));
#19813=CARTESIAN_POINT('Ctrl Pts',(3.15493079553585,0.659721306799046,57.7464246407004));
#19814=CARTESIAN_POINT('Ctrl Pts',(3.16516232242812,0.608742597816576,57.7433212621948));
#19815=CARTESIAN_POINT('Ctrl Pts',(3.18030452796812,0.52253594410534,57.7380313647149));
#19816=CARTESIAN_POINT('Ctrl Pts',(3.18587345172688,0.487432967305735,57.7358657832285));
#19817=CARTESIAN_POINT('Ctrl Pts',(3.19594792353134,0.416351683497813,57.7314540202528));
#19818=CARTESIAN_POINT('Ctrl Pts',(3.20042909687102,0.380375183808316,57.7292074151364));
#19819=CARTESIAN_POINT('Ctrl Pts',(3.21027376138446,0.288762168159615,57.7234487816755));
#19820=CARTESIAN_POINT('Ctrl Pts',(3.2147983655815,0.233049490379661,57.7199114154083));
#19821=CARTESIAN_POINT('Ctrl Pts',(3.23029217082074,-0.0482316991034988,
57.7018649371716));
#19822=CARTESIAN_POINT('Ctrl Pts',(3.21897644745742,-0.274362845236531,
57.6866888837325));
#19823=CARTESIAN_POINT('Ctrl Pts',(3.15982160339512,-0.653033594529865,
57.6608009758255));
#19824=CARTESIAN_POINT('Ctrl Pts',(3.12413385428399,-0.806672911467985,
57.6501793253463));
#19825=CARTESIAN_POINT('Ctrl Pts',(3.06691634995948,-0.990644225063457,
57.6377262915629));
#19826=CARTESIAN_POINT('Ctrl Pts',(3.05593417190987,-1.02402072591774,57.635478592567));
#19827=CARTESIAN_POINT('Ctrl Pts',(3.03753715548488,-1.07699779823064,57.6319367022852));
#19828=CARTESIAN_POINT('Ctrl Pts',(3.0304734944639,-1.0967163190735,57.6306241568628));
#19829=CARTESIAN_POINT('Ctrl Pts',(3.01600744814588,-1.13589168003481,57.6280300187548));
#19830=CARTESIAN_POINT('Ctrl Pts',(3.00860780279707,-1.15534842209092,57.6267483720005));
#19831=CARTESIAN_POINT('Ctrl Pts',(2.98844055814241,-1.20686848666052,57.6233692421735));
#19832=CARTESIAN_POINT('Ctrl Pts',(2.97534523209174,-1.23880163022747,57.6212899197271));
#19833=CARTESIAN_POINT('Ctrl Pts',(2.87884433953011,-1.46375717624347,57.6067083562));
#19834=CARTESIAN_POINT('Ctrl Pts',(2.77722700054671,-1.64844209560315,57.5950631146779));
#19835=CARTESIAN_POINT('Ctrl Pts',(2.5882554094643,-1.92416597647126,57.5763245108605));
#19836=CARTESIAN_POINT('Ctrl Pts',(2.51234635132951,-2.02227448472634,57.5693469378452));
#19837=CARTESIAN_POINT('Ctrl Pts',(2.39168404625158,-2.16091361971217,57.558747191949));
#19838=CARTESIAN_POINT('Ctrl Pts',(2.35113988230167,-2.2049582593451,57.5552585816594));
#19839=CARTESIAN_POINT('Ctrl Pts',(2.27359208394664,-2.28462937133571,57.5486909517378));
#19840=CARTESIAN_POINT('Ctrl Pts',(2.23691769887164,-2.32054974158849,57.5456253619101));
#19841=CARTESIAN_POINT('Ctrl Pts',(2.17350962106284,-2.37975385878226,57.5403803933288));
#19842=CARTESIAN_POINT('Ctrl Pts',(2.14722061240321,-2.40350077778701,57.5382211014456));
#19843=CARTESIAN_POINT('Ctrl Pts',(2.09313103548318,-2.4507642665179,57.533805583614));
#19844=CARTESIAN_POINT('Ctrl Pts',(2.06531276550229,-2.47425262058322,57.5315486548871));
#19845=CARTESIAN_POINT('Ctrl Pts',(1.99316131752587,-2.53310901936143,57.5257270458555));
#19846=CARTESIAN_POINT('Ctrl Pts',(1.94828313717074,-2.5677861117591,57.5221358955008));
#19847=CARTESIAN_POINT('Ctrl Pts',(1.72726646840164,-2.72943382840837,57.5045824560281));
#19848=CARTESIAN_POINT('Ctrl Pts',(1.5395372650818,-2.83955228568609,57.4900132958563));
#19849=CARTESIAN_POINT('Ctrl Pts',(1.18908557348437,-3.000092735002,57.4639745444006));
#19850=CARTESIAN_POINT('Ctrl Pts',(1.03069679576482,-3.0581292438205,57.4525979376705));
#19851=CARTESIAN_POINT('Ctrl Pts',(0.836608868096332,-3.11244259429169,
57.4396005828479));
#19852=CARTESIAN_POINT('Ctrl Pts',(0.804594551051987,-3.12087185037611,
57.4374869748035));
#19853=CARTESIAN_POINT('Ctrl Pts',(0.75252401882504,-3.13372727041929,57.4341042560607));
#19854=CARTESIAN_POINT('Ctrl Pts',(0.73254598776435,-3.13845749587943,57.4328194178716));
#19855=CARTESIAN_POINT('Ctrl Pts',(0.691772070086702,-3.14770101929637,
57.4302254545844));
#19856=CARTESIAN_POINT('Ctrl Pts',(0.67097415693125,-3.15219987361767,57.4289171063298));
#19857=CARTESIAN_POINT('Ctrl Pts',(0.614144107171793,-3.16390497480123,
57.425378508203));
#19858=CARTESIAN_POINT('Ctrl Pts',(0.578029820853918,-3.17070172920799,
57.4231695713823));
#19859=CARTESIAN_POINT('Ctrl Pts',(0.35667228352335,-3.2084534693292,57.4098291812621));
#19860=CARTESIAN_POINT('Ctrl Pts',(0.169112102368853,-3.22378745357848,
57.3993589396824));
#19861=CARTESIAN_POINT('Ctrl Pts',(-0.176784835446328,-3.22177683668667,
57.3799828441799));
#19862=CARTESIAN_POINT('Ctrl Pts',(-0.334490470502797,-3.20923297810243,
57.3711216961903));
#19863=CARTESIAN_POINT('Ctrl Pts',(-0.490582240097166,-3.18519177259412,
57.3619600447814));
#19864=CARTESIAN_POINT('Origin',(-9.35406549764863E-15,0.,41.4527091182931));
#19865=CARTESIAN_POINT('',(-0.490582094113513,-3.18519179507847,55.8661429281184));
#19866=CARTESIAN_POINT('',(-0.49058220660185,-3.18519177775306,56.1109990110886));
#19867=CARTESIAN_POINT('',(-0.490582094296226,-3.18519179505033,41.4527091182931));
#19868=CARTESIAN_POINT('Ctrl Pts',(-0.490582094113513,-3.18519179507847,
55.8661429281184));
#19869=CARTESIAN_POINT('Ctrl Pts',(-0.47670444968123,-3.18732922488018,
55.8670384748254));
#19870=CARTESIAN_POINT('Ctrl Pts',(-0.462812504433887,-3.18937600998039,
55.8679297983106));
#19871=CARTESIAN_POINT('Ctrl Pts',(-0.428211029566095,-3.1942432094582,
55.8701363448911));
#19872=CARTESIAN_POINT('Ctrl Pts',(-0.407486404536188,-3.19695312033762,
55.8714459329507));
#19873=CARTESIAN_POINT('Ctrl Pts',(-0.366029888983269,-3.20196419399069,
55.874039599157));
#19874=CARTESIAN_POINT('Ctrl Pts',(-0.345299098145667,-3.2042660885778,
55.8753236541104));
#19875=CARTESIAN_POINT('Ctrl Pts',(-0.2900088855317,-3.20986253539667,55.8787173338094));
#19876=CARTESIAN_POINT('Ctrl Pts',(-0.255415183741497,-3.21280032880294,
55.8808085154941));
#19877=CARTESIAN_POINT('Ctrl Pts',(-0.0127784440216769,-3.22946165812842,
55.8952927104781));
#19878=CARTESIAN_POINT('Ctrl Pts',(0.19614304644915,-3.22352829094271,55.9068455410471));
#19879=CARTESIAN_POINT('Ctrl Pts',(0.588178394484766,-3.17411124605778,
55.928994475777));
#19880=CARTESIAN_POINT('Ctrl Pts',(0.770914411840194,-3.13474354180852,
55.9395246334886));
#19881=CARTESIAN_POINT('Ctrl Pts',(0.997698312050101,-3.06484750303191,
55.9535510446941));
#19882=CARTESIAN_POINT('Ctrl Pts',(1.04582596875649,-3.04876036475308,55.9565828701577));
#19883=CARTESIAN_POINT('Ctrl Pts',(1.12677929858761,-3.01955852641632,55.9617877941285));
#19884=CARTESIAN_POINT('Ctrl Pts',(1.15980628279295,-3.00702752160471,55.9639415577062));
#19885=CARTESIAN_POINT('Ctrl Pts',(1.2265778419221,-2.98042958286822,55.9683611056681));
#19886=CARTESIAN_POINT('Ctrl Pts',(1.26030227251802,-2.96632629839689,55.9706278507027));
#19887=CARTESIAN_POINT('Ctrl Pts',(1.34642832032429,-2.92857523828918,55.9765093250905));
#19888=CARTESIAN_POINT('Ctrl Pts',(1.39844840145215,-2.90409427310019,55.980151615767));
#19889=CARTESIAN_POINT('Ctrl Pts',(1.63118595926614,-2.78686309019022,55.9968679769992));
#19890=CARTESIAN_POINT('Ctrl Pts',(1.80351938886978,-2.67855735466658,56.0104606601649));
#19891=CARTESIAN_POINT('Ctrl Pts',(2.06293104411941,-2.47908302951427,56.0325605787091));
#19892=CARTESIAN_POINT('Ctrl Pts',(2.15691535032348,-2.39776051821599,56.0409633809983));
#19893=CARTESIAN_POINT('Ctrl Pts',(2.29619436507772,-2.26241300559162,56.0538313522796));
#19894=CARTESIAN_POINT('Ctrl Pts',(2.34481369435936,-2.21198357967963,56.0584112750476));
#19895=CARTESIAN_POINT('Ctrl Pts',(2.40976248496615,-2.1400664063542,56.0646082076616));
#19896=CARTESIAN_POINT('Ctrl Pts',(2.42752112403396,-2.11990112066129,56.0663112408296));
#19897=CARTESIAN_POINT('Ctrl Pts',(2.45775939543882,-2.08468662931633,56.0692226271702));
#19898=CARTESIAN_POINT('Ctrl Pts',(2.470357560228,-2.06974229793869,56.0704390228371));
#19899=CARTESIAN_POINT('Ctrl Pts',(2.49809864744352,-2.03622076502335,56.0731247757435));
#19900=CARTESIAN_POINT('Ctrl Pts',(2.51317143908598,-2.01758797934894,56.0745894140769));
#19901=CARTESIAN_POINT('Ctrl Pts',(2.55954443531488,-1.95893615018212,56.079118649174));
#19902=CARTESIAN_POINT('Ctrl Pts',(2.59010851189404,-1.91834226992867,56.0821376347155));
#19903=CARTESIAN_POINT('Ctrl Pts',(2.73331671616837,-1.71847295094721,56.0965417879778));
#19904=CARTESIAN_POINT('Ctrl Pts',(2.83231019682779,-1.54990383381216,56.1073319787516));
#19905=CARTESIAN_POINT('Ctrl Pts',(2.98423636713134,-1.22739564660362,56.1273378692314));
#19906=CARTESIAN_POINT('Ctrl Pts',(3.04194603784082,-1.07644050393369,56.1364734983749));
#19907=CARTESIAN_POINT('Ctrl Pts',(3.10421208437822,-0.86784567607846,56.1492746312506));
#19908=CARTESIAN_POINT('Ctrl Pts',(3.11890163276317,-0.813474539407798,
56.1526252391296));
#19909=CARTESIAN_POINT('Ctrl Pts',(3.14071244108851,-0.723438265365074,
56.1582118220488));
#19910=CARTESIAN_POINT('Ctrl Pts',(3.14866821898781,-0.687986804370231,
56.1604210409529));
#19911=CARTESIAN_POINT('Ctrl Pts',(3.16312164009831,-0.618068561490217,
56.1648003310201));
#19912=CARTESIAN_POINT('Ctrl Pts',(3.16965935520165,-0.583615177516491,
56.166968791248));
#19913=CARTESIAN_POINT('Ctrl Pts',(3.18437365578035,-0.498511604972874,
56.1723537130019));
#19914=CARTESIAN_POINT('Ctrl Pts',(3.19190520724935,-0.447761173836143,
56.1755898173135));
#19915=CARTESIAN_POINT('Ctrl Pts',(3.2302866202595,-0.138448366816227,56.1954743207642));
#19916=CARTESIAN_POINT('Ctrl Pts',(3.23091024889173,0.122854387471132,56.2130669271184));
#19917=CARTESIAN_POINT('Ctrl Pts',(3.18893482938931,0.475113758040776,56.2369964425577));
#19918=CARTESIAN_POINT('Ctrl Pts',(3.17364099128598,0.568368749314567,56.2433387032443));
#19919=CARTESIAN_POINT('Ctrl Pts',(3.14574154603605,0.70154007975339,56.2523029659562));
#19920=CARTESIAN_POINT('Ctrl Pts',(3.13642287670455,0.74209177557174,56.2550198158851));
#19921=CARTESIAN_POINT('Ctrl Pts',(3.11821209969496,0.814853604234161,56.2598585442939));
#19922=CARTESIAN_POINT('Ctrl Pts',(3.10959943034297,0.847127310274433,56.2619917936124));
#19923=CARTESIAN_POINT('Ctrl Pts',(3.09486913226624,0.899069790828841,56.2653977364233));
#19924=CARTESIAN_POINT('Ctrl Pts',(3.0890621621364,0.918823412828881,56.266686536685));
#19925=CARTESIAN_POINT('Ctrl Pts',(3.07689197904674,0.958802788549101,56.269279881261));
#19926=CARTESIAN_POINT('Ctrl Pts',(3.0705177399317,0.979023955243096,56.2705837807056));
#19927=CARTESIAN_POINT('Ctrl Pts',(3.05266689599205,1.03376275462796,56.2740959343032));
#19928=CARTESIAN_POINT('Ctrl Pts',(3.04080440289872,1.06815234990088,56.2762834098996));
#19929=CARTESIAN_POINT('Ctrl Pts',(2.96226897875499,1.28390672583224,56.2899297652349));
#19930=CARTESIAN_POINT('Ctrl Pts',(2.87997276202006,1.45918736029554,56.3006842756705));
#19931=CARTESIAN_POINT('Ctrl Pts',(2.71569104769115,1.74030178001293,56.3189247676308));
#19932=CARTESIAN_POINT('Ctrl Pts',(2.64195380804453,1.8503258137384,56.3263511990141));
#19933=CARTESIAN_POINT('Ctrl Pts',(2.52402775760024,2.00480649901951,56.3375389904976));
#19934=CARTESIAN_POINT('Ctrl Pts',(2.48497554605672,2.05301269454797,56.3411480963542));
#19935=CARTESIAN_POINT('Ctrl Pts',(2.41021738422415,2.14003433369257,56.3479162099498));
#19936=CARTESIAN_POINT('Ctrl Pts',(2.3749027870915,2.1791583406538,56.3510601803951));
#19937=CARTESIAN_POINT('Ctrl Pts',(2.31410666266537,2.24327884102337,56.3563984183446));
#19938=CARTESIAN_POINT('Ctrl Pts',(2.28913990124072,2.26875030806929,56.3585708221852));
#19939=CARTESIAN_POINT('Ctrl Pts',(2.23806354121418,2.31915764973697,56.3629792488577));
#19940=CARTESIAN_POINT('Ctrl Pts',(2.21194744237422,2.34407955571488,56.3652154050871));
#19941=CARTESIAN_POINT('Ctrl Pts',(2.1449502155314,2.40589653163552,56.3709104276494));
#19942=CARTESIAN_POINT('Ctrl Pts',(2.10353317742379,2.44219105097937,56.3743935063971));
#19943=CARTESIAN_POINT('Ctrl Pts',(1.88203893702601,2.62647493840984,56.3928384337499));
#19944=CARTESIAN_POINT('Ctrl Pts',(1.68725166408408,2.75564704606478,56.4085202932165));
#19945=CARTESIAN_POINT('Ctrl Pts',(1.38522339005281,2.9118251449608,56.4314837317641));
#19946=CARTESIAN_POINT('Ctrl Pts',(1.28777264186515,2.95621602239485,56.4386960798101));
#19947=CARTESIAN_POINT('Ctrl Pts',(1.14673207983078,3.01216233257248,56.4487196328347));
#19948=CARTESIAN_POINT('Ctrl Pts',(1.10483354061134,3.02778129904125,56.4516468943765));
#19949=CARTESIAN_POINT('Ctrl Pts',(1.02935303677655,3.05414336653264,56.4568152507961));
#19950=CARTESIAN_POINT('Ctrl Pts',(0.995894395060094,3.06521678928511,56.4590699900929));
#19951=CARTESIAN_POINT('Ctrl Pts',(0.942249672518553,3.08199978786892,56.4626202237089));
#19952=CARTESIAN_POINT('Ctrl Pts',(0.922178750631355,3.08806469275649,56.4639342139344));
#19953=CARTESIAN_POINT('Ctrl Pts',(0.882087236783464,3.0997535436629,56.4665284938078));
#19954=CARTESIAN_POINT('Ctrl Pts',(0.862068609168573,3.10538044172264,56.4678088767183));
#19955=CARTESIAN_POINT('Ctrl Pts',(0.808785512829795,3.11980244888435,56.4711805404664));
#19956=CARTESIAN_POINT('Ctrl Pts',(0.775431349086768,3.12825954205491,56.4732538042292));
#19957=CARTESIAN_POINT('Ctrl Pts',(0.536450082281223,3.18479688517124,56.4878848007231));
#19958=CARTESIAN_POINT('Ctrl Pts',(0.326647292156141,3.21310333627802,56.4995769360888));
#19959=CARTESIAN_POINT('Ctrl Pts',(-0.00787833689097536,3.22510664609324,
56.518343107162));
#19960=CARTESIAN_POINT('Ctrl Pts',(-0.131466998268363,3.22243524287872,
56.5252977480078));
#19961=CARTESIAN_POINT('Ctrl Pts',(-0.314145882711706,3.20795868050048,
56.5358672764335));
#19962=CARTESIAN_POINT('Ctrl Pts',(-0.373554652365925,3.20158443251951,
56.5393495261672));
#19963=CARTESIAN_POINT('Ctrl Pts',(-0.483542419707747,3.18668033611588,
56.5459065319408));
#19964=CARTESIAN_POINT('Ctrl Pts',(-0.534161461463274,3.17858709762858,
56.5489679404079));
#19965=CARTESIAN_POINT('Ctrl Pts',(-0.619388244642953,3.16286733055723,
56.5542078987026));
#19966=CARTESIAN_POINT('Ctrl Pts',(-0.654103134020785,3.15587079653844,
56.5563664546534));
#19967=CARTESIAN_POINT('Ctrl Pts',(-0.724276330986334,3.14052033868824,
56.5607822979248));
#19968=CARTESIAN_POINT('Ctrl Pts',(-0.759722279522704,3.13213442993292,
56.5630403187705));
#19969=CARTESIAN_POINT('Ctrl Pts',(-0.850059794046157,3.1091384491417,56.5688688078742));
#19970=CARTESIAN_POINT('Ctrl Pts',(-0.904719212054918,3.09367516885826,
56.5724658721226));
#19971=CARTESIAN_POINT('Ctrl Pts',(-1.16513282242976,3.01251206080619,56.5899531173097));
#19972=CARTESIAN_POINT('Ctrl Pts',(-1.36431596881225,2.92769182767227,56.6044425727736));
#19973=CARTESIAN_POINT('Ctrl Pts',(-1.70186246377706,2.74198091464352,56.6304669194268));
#19974=CARTESIAN_POINT('Ctrl Pts',(-1.84358136506399,2.64877564821555,56.6419090284364));
#19975=CARTESIAN_POINT('Ctrl Pts',(-2.00347763309022,2.52453790421698,56.654967539123));
#19976=CARTESIAN_POINT('Ctrl Pts',(-2.02931455270895,2.50381646684228,56.6570820993504));
#19977=CARTESIAN_POINT('Ctrl Pts',(-2.07064536373954,2.46960864950359,56.660465917439));
#19978=CARTESIAN_POINT('Ctrl Pts',(-2.08633734176591,2.45636635574517,56.6617509213592));
#19979=CARTESIAN_POINT('Ctrl Pts',(-2.11802790831272,2.42910021773898,56.6643447469881));
#19980=CARTESIAN_POINT('Ctrl Pts',(-2.13401619253562,2.41506625930702,56.6656527991246));
#19981=CARTESIAN_POINT('Ctrl Pts',(-2.17722194371027,2.37637763832796,56.6691898050035));
#19982=CARTESIAN_POINT('Ctrl Pts',(-2.20415963682996,2.35141374975379,56.671397476776));
#19983=CARTESIAN_POINT('Ctrl Pts',(-2.39560230770309,2.16781709975211,56.687156021637));
#19984=CARTESIAN_POINT('Ctrl Pts',(-2.54326602324136,1.9925271211549,56.6997218025243));
#19985=CARTESIAN_POINT('Ctrl Pts',(-2.73309519742439,1.71130532520461,56.7187858117523));
#19986=CARTESIAN_POINT('Ctrl Pts',(-2.79026517818625,1.61641373081543,56.725051730982));
#19987=CARTESIAN_POINT('Ctrl Pts',(-2.87976139486696,1.44891845261527,56.7360404852419));
#19988=CARTESIAN_POINT('Ctrl Pts',(-2.91449605258379,1.37771612195877,56.7406903348094));
#19989=CARTESIAN_POINT('Ctrl Pts',(-2.96300379955642,1.2682160977233,56.7478551755739));
#19990=CARTESIAN_POINT('Ctrl Pts',(-2.9787338318114,1.23081603875404,56.7503045430426));
#19991=CARTESIAN_POINT('Ctrl Pts',(-3.00644600427892,1.16128179931595,56.7548676906535));
#19992=CARTESIAN_POINT('Ctrl Pts',(-3.01862944661091,1.12923386242605,56.7569743705802));
#19993=CARTESIAN_POINT('Ctrl Pts',(-3.04469977284466,1.05721838103859,56.7617190010019));
#19994=CARTESIAN_POINT('Ctrl Pts',(-3.05831531635106,1.01716005002643,56.7643654460466));
#19995=CARTESIAN_POINT('Ctrl Pts',(-3.09835471442656,0.891278983986175,
56.7727087230335));
#19996=CARTESIAN_POINT('Ctrl Pts',(-3.12198127854482,0.804618311694492,
56.7784925252685));
#19997=CARTESIAN_POINT('Ctrl Pts',(-3.19580997906034,0.481135234170011,
56.8002219860887));
#19998=CARTESIAN_POINT('Ctrl Pts',(-3.22290709110659,0.239875915335549,
56.8167722868544));
#19999=CARTESIAN_POINT('Ctrl Pts',(-3.22268781229327,-0.0964266138825664,
56.8392710364056));
#20000=CARTESIAN_POINT('Ctrl Pts',(-3.21848516002261,-0.19071206053494,
56.8455055763825));
#20001=CARTESIAN_POINT('Ctrl Pts',(-3.20750067365725,-0.314575060533712,
56.8534938739027));
#20002=CARTESIAN_POINT('Ctrl Pts',(-3.20443242981268,-0.344428503107231,
56.85540353909));
#20003=CARTESIAN_POINT('Ctrl Pts',(-3.19865291071894,-0.393862389159491,
56.8585349646516));
#20004=CARTESIAN_POINT('Ctrl Pts',(-3.19617775182092,-0.413468119291994,
56.8597687931013));
#20005=CARTESIAN_POINT('Ctrl Pts',(-3.19053934935145,-0.455048348932169,
56.862366875966));
#20006=CARTESIAN_POINT('Ctrl Pts',(-3.18732915729476,-0.477014935039213,
56.8637286352716));
#20007=CARTESIAN_POINT('Ctrl Pts',(-3.1774972106612,-0.539754739861388,
56.8675915824539));
#20008=CARTESIAN_POINT('Ctrl Pts',(-3.17031801139851,-0.580437559142972,
56.8700644258148));
#20009=CARTESIAN_POINT('Ctrl Pts',(-3.15165928328733,-0.675458710877265,
56.875788317086));
#20010=CARTESIAN_POINT('Ctrl Pts',(-3.13955339492991,-0.729661426069452,
56.8790133507642));
#20011=CARTESIAN_POINT('Ctrl Pts',(-3.08657282978102,-0.941039040599342,
56.891525386038));
#20012=CARTESIAN_POINT('Ctrl Pts',(-3.03524329246229,-1.09534897354148,
56.9005274824662));
#20013=CARTESIAN_POINT('Ctrl Pts',(-2.90797420169957,-1.39917649074966,
56.919029781238));
#20014=CARTESIAN_POINT('Ctrl Pts',(-2.83158073567251,-1.547950601993,56.9285127391271));
#20015=CARTESIAN_POINT('Ctrl Pts',(-2.71776850439516,-1.73273066165305,
56.9413487171698));
#20016=CARTESIAN_POINT('Ctrl Pts',(-2.69054019086809,-1.7747152635268,56.9443402225764));
#20017=CARTESIAN_POINT('Ctrl Pts',(-2.64270507366503,-1.84484210203831,
56.9494764573911));
#20018=CARTESIAN_POINT('Ctrl Pts',(-2.62259831550368,-1.87331535421201,
56.9516024003649));
#20019=CARTESIAN_POINT('Ctrl Pts',(-2.58040604001634,-1.93105307955987,
56.9560005114345));
#20020=CARTESIAN_POINT('Ctrl Pts',(-2.55827513279346,-1.96027791315073,
56.9582742283772));
#20021=CARTESIAN_POINT('Ctrl Pts',(-2.4998319705294,-2.03477901321709,56.9641979775069));
#20022=CARTESIAN_POINT('Ctrl Pts',(-2.46278784603072,-2.07946167326016,
56.9678763492484));
#20023=CARTESIAN_POINT('Ctrl Pts',(-2.30947364543152,-2.25454352882659,
56.9828113549079));
#20024=CARTESIAN_POINT('Ctrl Pts',(-2.18390711485839,-2.37637756037815,
56.9944328268553));
#20025=CARTESIAN_POINT('Ctrl Pts',(-1.89154285511145,-2.61722308799599,
57.019965039001));
#20026=CARTESIAN_POINT('Ctrl Pts',(-1.72199565712268,-2.7317635137031,57.0338791711534));
#20027=CARTESIAN_POINT('Ctrl Pts',(-1.51182289155625,-2.84635721979762,
57.0493533901504));
#20028=CARTESIAN_POINT('Ctrl Pts',(-1.48062646122085,-2.86270910045825,
57.0516067231796));
#20029=CARTESIAN_POINT('Ctrl Pts',(-1.43044397967395,-2.88797281387489,
57.0551552852409));
#20030=CARTESIAN_POINT('Ctrl Pts',(-1.41162900444431,-2.89721600220376,
57.0564689818545));
#20031=CARTESIAN_POINT('Ctrl Pts',(-1.37396939336562,-2.91526297354355,
57.0590632169092));
#20032=CARTESIAN_POINT('Ctrl Pts',(-1.3551270998134,-2.92406920103678,57.0603438408823));
#20033=CARTESIAN_POINT('Ctrl Pts',(-1.30487266002862,-2.94696624716074,
57.0637169508428));
#20034=CARTESIAN_POINT('Ctrl Pts',(-1.27331686516579,-2.96073759320142,
57.0657913918869));
#20035=CARTESIAN_POINT('Ctrl Pts',(-1.20156321774696,-2.99069231707555,
57.0704237587892));
#20036=CARTESIAN_POINT('Ctrl Pts',(-1.16124706578631,-3.00657617311166,
57.0729676164234));
#20037=CARTESIAN_POINT('Ctrl Pts',(-1.02565995311446,-3.05686066842746,
57.0813658825689));
#20038=CARTESIAN_POINT('Ctrl Pts',(-0.92908579829348,-3.08758438891062,
57.0870938219642));
#20039=CARTESIAN_POINT('Ctrl Pts',(-0.71895002008604,-3.14368117062449,
57.0993140318433));
#20040=CARTESIAN_POINT('Ctrl Pts',(-0.605236661070453,-3.16753275047228,
57.1057815379584));
#20041=CARTESIAN_POINT('Ctrl Pts',(-0.490581808115708,-3.18519183912774,
57.1123311812828));
#20042=CARTESIAN_POINT('Ctrl Pts',(-0.490582240097165,-3.18519177259412,
57.3619600447814));
#20043=CARTESIAN_POINT('Ctrl Pts',(-0.528616395488554,-3.17933376388247,
57.3597276678007));
#20044=CARTESIAN_POINT('Ctrl Pts',(-0.566554773874653,-3.17279310424186,
57.3574782319896));
#20045=CARTESIAN_POINT('Ctrl Pts',(-0.657353474889526,-3.1554575811956,
57.3520309897278));
#20046=CARTESIAN_POINT('Ctrl Pts',(-0.710063144317063,-3.14401589865181,
57.3488165503753));
#20047=CARTESIAN_POINT('Ctrl Pts',(-0.797329981891067,-3.12276649170889,
57.3433938679773));
#20048=CARTESIAN_POINT('Ctrl Pts',(-0.832055764269073,-3.11369374011445,
57.341209120607));
#20049=CARTESIAN_POINT('Ctrl Pts',(-0.90116188029666,-3.09439991633808,
57.3368038840464));
#20050=CARTESIAN_POINT('Ctrl Pts',(-0.935537490481778,-3.08418109333674,
57.3345837387818));
#20051=CARTESIAN_POINT('Ctrl Pts',(-1.02101466384346,-3.05721083487565,
57.3289877996397));
#20052=CARTESIAN_POINT('Ctrl Pts',(-1.07187935136914,-3.03975050596263,
57.3255895231349));
#20053=CARTESIAN_POINT('Ctrl Pts',(-1.35017156914257,-2.93636773752018,
57.3066066019719));
#20054=CARTESIAN_POINT('Ctrl Pts',(-1.56771828938307,-2.82620618732505,
57.2902240416626));
#20055=CARTESIAN_POINT('Ctrl Pts',(-1.85613349627362,-2.63653614801889,
57.2669189161702));
#20056=CARTESIAN_POINT('Ctrl Pts',(-1.93877758632558,-2.57637299759377,
57.2600428463621));
#20057=CARTESIAN_POINT('Ctrl Pts',(-2.05237161865966,-2.48511251269254,
57.2504263656573));
#20058=CARTESIAN_POINT('Ctrl Pts',(-2.08576134547418,-2.45715555370437,
57.2475781827734));
#20059=CARTESIAN_POINT('Ctrl Pts',(-2.14461419195035,-2.40581410636247,
57.2425333042742));
#20060=CARTESIAN_POINT('Ctrl Pts',(-2.17028691670122,-2.38268052148736,
57.2403238390731));
#20061=CARTESIAN_POINT('Ctrl Pts',(-2.21082779571737,-2.34495025061651,
57.2368274009425));
#20062=CARTESIAN_POINT('Ctrl Pts',(-2.22593449617254,-2.33061513303711,
57.2355228347075));
#20063=CARTESIAN_POINT('Ctrl Pts',(-2.25594755574726,-2.30157695437281,
57.2329295306156));
#20064=CARTESIAN_POINT('Ctrl Pts',(-2.27085170100453,-2.28687307463408,
57.2316409584689));
#20065=CARTESIAN_POINT('Ctrl Pts',(-2.31034942376289,-2.24713914267313,
57.2282205017733));
#20066=CARTESIAN_POINT('Ctrl Pts',(-2.33467994111702,-2.22185026147899,
57.2261075784178));
#20067=CARTESIAN_POINT('Ctrl Pts',(-2.49845997688234,-2.04595726480858,
57.2118009763286));
#20068=CARTESIAN_POINT('Ctrl Pts',(-2.62367386487158,-1.88271048827538,
57.200417263054));
#20069=CARTESIAN_POINT('Ctrl Pts',(-2.8297366118413,-1.55316860075325,57.1786346129206));
#20070=CARTESIAN_POINT('Ctrl Pts',(-2.91349988128619,-1.38969468509997,
57.1682972974079));
#20071=CARTESIAN_POINT('Ctrl Pts',(-3.00310887193664,-1.17059930024392,
57.1543411321359));
#20072=CARTESIAN_POINT('Ctrl Pts',(-3.02208040672273,-1.12071189441505,
57.1511589541182));
#20073=CARTESIAN_POINT('Ctrl Pts',(-3.05168990622288,-1.03662288124369,
57.1457749557538));
#20074=CARTESIAN_POINT('Ctrl Pts',(-3.06301248925283,-1.00267273520027,
57.1435958792124));
#20075=CARTESIAN_POINT('Ctrl Pts',(-3.08457605985087,-0.93423854665951,
57.1391894118032));
#20076=CARTESIAN_POINT('Ctrl Pts',(-3.09480971998556,-0.899757613207197,
57.1369621494825));
#20077=CARTESIAN_POINT('Ctrl Pts',(-3.11905262462062,-0.81276185640739,
57.1313221504434));
#20078=CARTESIAN_POINT('Ctrl Pts',(-3.13231406278992,-0.760052073671085,
57.1278861668829));
#20079=CARTESIAN_POINT('Ctrl Pts',(-3.1966232932322,-0.474064111955712,
57.109133148888));
#20080=CARTESIAN_POINT('Ctrl Pts',(-3.22294807162268,-0.236025879415922,
57.0930523698287));
#20081=CARTESIAN_POINT('Ctrl Pts',(-3.22263065423201,0.144369481261549,
57.0673664502987));
#20082=CARTESIAN_POINT('Ctrl Pts',(-3.21316958118118,0.285899179383458,
57.0578333077411));
#20083=CARTESIAN_POINT('Ctrl Pts',(-3.18933104872129,0.464506651136535,
57.0461463786206));
#20084=CARTESIAN_POINT('Ctrl Pts',(-3.1835558176421,0.502565040915061,57.0436766772242));
#20085=CARTESIAN_POINT('Ctrl Pts',(-3.17347134504083,0.561840943787612,
57.0398716355887));
#20086=CARTESIAN_POINT('Ctrl Pts',(-3.16962801691703,0.583132849548935,
57.0385132907892));
#20087=CARTESIAN_POINT('Ctrl Pts',(-3.1617663835976,0.624309498041845,57.0359048417039));
#20088=CARTESIAN_POINT('Ctrl Pts',(-3.15777427376064,0.644197696971805,
57.0346535468147));
#20089=CARTESIAN_POINT('Ctrl Pts',(-3.14703435003528,0.695202148264648,
57.0314637198799));
#20090=CARTESIAN_POINT('Ctrl Pts',(-3.14001251429949,0.726259465015385,
57.0295397682748));
#20091=CARTESIAN_POINT('Ctrl Pts',(-3.10148683257822,0.885638071081805,
57.0197377274504));
#20092=CARTESIAN_POINT('Ctrl Pts',(-3.06257026290644,1.01205034349357,57.0121993307134));
#20093=CARTESIAN_POINT('Ctrl Pts',(-2.92588144408565,1.37503644571576,56.9903393362015));
#20094=CARTESIAN_POINT('Ctrl Pts',(-2.80761224600205,1.60275220779664,56.9762712783642));
#20095=CARTESIAN_POINT('Ctrl Pts',(-2.63168424484929,1.86107113983018,56.9579008786663));
#20096=CARTESIAN_POINT('Ctrl Pts',(-2.59845629744995,1.90718956757727,56.9545205015128));
#20097=CARTESIAN_POINT('Ctrl Pts',(-2.54195715546749,1.98138804991861,56.9488978815025));
#20098=CARTESIAN_POINT('Ctrl Pts',(-2.51939736447835,2.00999540746983,56.9466831250393));
#20099=CARTESIAN_POINT('Ctrl Pts',(-2.47396421076819,2.06564091951147,56.9422776840643));
#20100=CARTESIAN_POINT('Ctrl Pts',(-2.45112050867779,2.09269668577328,56.9400883731959));
#20101=CARTESIAN_POINT('Ctrl Pts',(-2.39414436143811,2.15796550523621,56.9346866658749));
#20102=CARTESIAN_POINT('Ctrl Pts',(-2.35953845406876,2.19575047575958,56.9314550773603));
#20103=CARTESIAN_POINT('Ctrl Pts',(-2.28268710674562,2.27574635443214,56.9243785670789));
#20104=CARTESIAN_POINT('Ctrl Pts',(-2.24013988672676,2.31763985149693,56.92052190858));
#20105=CARTESIAN_POINT('Ctrl Pts',(-2.10617269548767,2.44241185593695,56.9085637623392));
#20106=CARTESIAN_POINT('Ctrl Pts',(-2.01114259494639,2.5212378215737,56.9003279005751));
#20107=CARTESIAN_POINT('Ctrl Pts',(-1.74157465162653,2.71988341876357,56.8777719394522));
#20108=CARTESIAN_POINT('Ctrl Pts',(-1.55936847360893,2.82829066686042,56.8633370472115));
#20109=CARTESIAN_POINT('Ctrl Pts',(-1.33672482780621,2.93265505104793,56.8474569318508));
#20110=CARTESIAN_POINT('Ctrl Pts',(-1.30537064805736,2.9467450862445,56.8452595700417));
#20111=CARTESIAN_POINT('Ctrl Pts',(-1.25470173153,2.96854732247601,56.8417775242171));
#20112=CARTESIAN_POINT('Ctrl Pts',(-1.23552809244358,2.97657857868915,56.8404754846363));
#20113=CARTESIAN_POINT('Ctrl Pts',(-1.1968534942814,2.99234009235655,56.8378823438486));
#20114=CARTESIAN_POINT('Ctrl Pts',(-1.1773521324151,3.00006658724949,56.8365914816703));
#20115=CARTESIAN_POINT('Ctrl Pts',(-1.12485122755343,3.02027680299959,56.8331573613142));
#20116=CARTESIAN_POINT('Ctrl Pts',(-1.09171892556598,3.03241030654612,56.8310333309168));
#20117=CARTESIAN_POINT('Ctrl Pts',(-1.01609885996644,3.0587032671405,56.8262686762409));
#20118=CARTESIAN_POINT('Ctrl Pts',(-0.973501345665638,3.07252633167772,
56.8236433648069));
#20119=CARTESIAN_POINT('Ctrl Pts',(-0.827895540025725,3.11644357669647,
56.8148247065277));
#20120=CARTESIAN_POINT('Ctrl Pts',(-0.723673924140468,3.142281051443,56.8087715379145));
#20121=CARTESIAN_POINT('Ctrl Pts',(-0.390197211506187,3.20747690972804,
56.7897022532714));
#20122=CARTESIAN_POINT('Ctrl Pts',(-0.157906703169872,3.22726164570263,
56.7768038713047));
#20123=CARTESIAN_POINT('Ctrl Pts',(0.129603295213574,3.22061488165758,56.7598751109661));
#20124=CARTESIAN_POINT('Ctrl Pts',(0.184677365624063,3.21792650188442,56.7565919510726));
#20125=CARTESIAN_POINT('Ctrl Pts',(0.275665038386236,3.21114160687779,56.7510866568729));
#20126=CARTESIAN_POINT('Ctrl Pts',(0.311628104763981,3.20785121143749,56.7488896459302));
#20127=CARTESIAN_POINT('Ctrl Pts',(0.382975766200873,3.20011226519172,56.7444855927078));
#20128=CARTESIAN_POINT('Ctrl Pts',(0.418356890651453,3.1956793171569,56.7422793357473));
#20129=CARTESIAN_POINT('Ctrl Pts',(0.505773843253056,3.18325015559359,56.7367700172121));
#20130=CARTESIAN_POINT('Ctrl Pts',(0.557699591627092,3.17456443976123,56.733445955008));
#20131=CARTESIAN_POINT('Ctrl Pts',(0.806608589090579,3.1266337793043,56.7172543094878));
#20132=CARTESIAN_POINT('Ctrl Pts',(0.999819630099894,3.07030857137375,56.7038641530815));
#20133=CARTESIAN_POINT('Ctrl Pts',(1.35963244771787,2.92783020926508,56.6777450358051));
#20134=CARTESIAN_POINT('Ctrl Pts',(1.5265029539427,2.84439590346127,56.6650967169967));
#20135=CARTESIAN_POINT('Ctrl Pts',(1.71661144367588,2.72776778437452,56.6506554727207));
#20136=CARTESIAN_POINT('Ctrl Pts',(1.74765021781395,2.70798650536941,56.6482974431587));
#20137=CARTESIAN_POINT('Ctrl Pts',(1.79609969212866,2.67592912955357,56.6446245549487));
#20138=CARTESIAN_POINT('Ctrl Pts',(1.81373833918672,2.66400527528795,56.6432890789227));
#20139=CARTESIAN_POINT('Ctrl Pts',(1.8481438813376,2.64024674046124,56.6406895042798));
#20140=CARTESIAN_POINT('Ctrl Pts',(1.86491822502484,2.62842513765273,56.6394247663321));
#20141=CARTESIAN_POINT('Ctrl Pts',(1.90841623696524,2.59714415319372,56.6361490092902));
#20142=CARTESIAN_POINT('Ctrl Pts',(1.93495626078633,2.57743181221607,56.6341541772658));
#20143=CARTESIAN_POINT('Ctrl Pts',(2.09500673429521,2.45469001099885,56.6221165519411));
#20144=CARTESIAN_POINT('Ctrl Pts',(2.22057847839881,2.34170885431434,56.6126301846416));
#20145=CARTESIAN_POINT('Ctrl Pts',(2.48613639395769,2.06211156412784,56.5910138039755));
#20146=CARTESIAN_POINT('Ctrl Pts',(2.61925587011288,1.8901500982262,56.5789313584732));
#20147=CARTESIAN_POINT('Ctrl Pts',(2.76411827132919,1.65800636262168,56.5628460336113));
#20148=CARTESIAN_POINT('Ctrl Pts',(2.7928697056949,1.60910321326351,56.5594721116918));
#20149=CARTESIAN_POINT('Ctrl Pts',(2.83793300675741,1.52760580019844,56.5538572944632));
#20150=CARTESIAN_POINT('Ctrl Pts',(2.85500963846013,1.49544743465277,56.5516437263571));
#20151=CARTESIAN_POINT('Ctrl Pts',(2.88761827610561,1.43144440699284,56.5472384712733));
#20152=CARTESIAN_POINT('Ctrl Pts',(2.90317726564428,1.39961923573217,56.545048120027));
#20153=CARTESIAN_POINT('Ctrl Pts',(2.93998530508501,1.32107446127606,56.5396397382782));
#20154=CARTESIAN_POINT('Ctrl Pts',(2.96064838831183,1.27409260556704,56.536402404589));
#20155=CARTESIAN_POINT('Ctrl Pts',(3.00295635081758,1.17130336132989,56.5293109042868));
#20156=CARTESIAN_POINT('Ctrl Pts',(3.02418580093954,1.11534655708579,56.5254449083658));
#20157=CARTESIAN_POINT('Ctrl Pts',(3.08454914157848,0.941819233628293,56.513442553246));
#20158=CARTESIAN_POINT('Ctrl Pts',(3.11846936556817,0.822563823904482,56.5051706797111));
#20159=CARTESIAN_POINT('Ctrl Pts',(3.19124924603733,0.496302722796112,56.4826510771134));
#20160=CARTESIAN_POINT('Ctrl Pts',(3.21684046069395,0.286941853983922,56.4682934616393));
#20161=CARTESIAN_POINT('Ctrl Pts',(3.22265983724127,0.0420849375795456,
56.4524734239454));
#20162=CARTESIAN_POINT('Ctrl Pts',(3.22292572783027,0.00758564547516927,
56.4502677627509));
#20163=CARTESIAN_POINT('Ctrl Pts',(3.2224638228948,-0.047724523493845,56.4467758529688));
#20164=CARTESIAN_POINT('Ctrl Pts',(3.22208841634583,-0.0685347891252205,
56.4454720857196));
#20165=CARTESIAN_POINT('Ctrl Pts',(3.22093070862584,-0.110280263771302,
56.4428788483934));
#20166=CARTESIAN_POINT('Ctrl Pts',(3.22014583698556,-0.131214371300375,
56.4415895669234));
#20167=CARTESIAN_POINT('Ctrl Pts',(3.21749759655341,-0.187248952041684,
56.4381648739455));
#20168=CARTESIAN_POINT('Ctrl Pts',(3.21526399231875,-0.222330025129312,
56.4360485061869));
#20169=CARTESIAN_POINT('Ctrl Pts',(3.19972431648013,-0.416294782983535,
56.4244662067931));
#20170=CARTESIAN_POINT('Ctrl Pts',(3.17521441052865,-0.574074312448822,
56.4154812662513));
#20171=CARTESIAN_POINT('Ctrl Pts',(3.08857924390017,-0.946923869543753,
56.3940145063559));
#20172=CARTESIAN_POINT('Ctrl Pts',(3.01557093985495,-1.15858050863655,56.3815966511459));
#20173=CARTESIAN_POINT('Ctrl Pts',(2.89756360208515,-1.41187637228609,56.3651621607647));
#20174=CARTESIAN_POINT('Ctrl Pts',(2.87252896379868,-1.46213765235327,56.3618212353156));
#20175=CARTESIAN_POINT('Ctrl Pts',(2.82916747646319,-1.54377676857688,56.3562462819122));
#20176=CARTESIAN_POINT('Ctrl Pts',(2.811599648374,-1.57554516710002,56.3540387727067));
#20177=CARTESIAN_POINT('Ctrl Pts',(2.77579566901384,-1.63778401756406,56.349634282699));
#20178=CARTESIAN_POINT('Ctrl Pts',(2.75758509697339,-1.66826327601977,56.34743844144));
#20179=CARTESIAN_POINT('Ctrl Pts',(2.71158632281412,-1.74244035037105,56.3419949712612));
#20180=CARTESIAN_POINT('Ctrl Pts',(2.68324212780437,-1.7857799281773,56.3387274525053));
#20181=CARTESIAN_POINT('Ctrl Pts',(2.54161483072516,-1.99134587978948,56.322794573898));
#20182=CARTESIAN_POINT('Ctrl Pts',(2.41461308575272,-2.14356864449937,56.3096211050842));
#20183=CARTESIAN_POINT('Ctrl Pts',(2.13873446261977,-2.41839745623974,56.2833484804977));
#20184=CARTESIAN_POINT('Ctrl Pts',(1.99119116298506,-2.54125923587026,56.2703189992719));
#20185=CARTESIAN_POINT('Ctrl Pts',(1.80357338840829,-2.67106225735202,56.2555512535026));
#20186=CARTESIAN_POINT('Ctrl Pts',(1.77319630560614,-2.69132414793122,56.2532125159911));
#20187=CARTESIAN_POINT('Ctrl Pts',(1.7246211812975,-2.7225447720268,56.2495625052813));
#20188=CARTESIAN_POINT('Ctrl Pts',(1.70664875693812,-2.73384680148835,56.2482310172543));
#20189=CARTESIAN_POINT('Ctrl Pts',(1.67104724562507,-2.7557470272628,56.2456326608416));
#20190=CARTESIAN_POINT('Ctrl Pts',(1.65342599662417,-2.76635556015612,56.2443652523415));
#20191=CARTESIAN_POINT('Ctrl Pts',(1.60702002156084,-2.79369155064803,56.2410728881965));
#20192=CARTESIAN_POINT('Ctrl Pts',(1.57807467715588,-2.81014347297185,56.2390644333779));
#20193=CARTESIAN_POINT('Ctrl Pts',(1.51255487041812,-2.84605182978926,56.2346067184971));
#20194=CARTESIAN_POINT('Ctrl Pts',(1.47584939481442,-2.86525777431323,56.2321699655945));
#20195=CARTESIAN_POINT('Ctrl Pts',(1.35489777665518,-2.92560383677135,56.2243033348266));
#20196=CARTESIAN_POINT('Ctrl Pts',(1.26922212481919,-2.9637784934947,56.2189834736516));
#20197=CARTESIAN_POINT('Ctrl Pts',(0.938244169545973,-3.09426357872117,
56.1989557983675));
#20198=CARTESIAN_POINT('Ctrl Pts',(0.683702014462386,-3.16027086118547,
56.1845209890317));
#20199=CARTESIAN_POINT('Ctrl Pts',(0.373369530560781,-3.20145583187507,
56.1660234575779));
#20200=CARTESIAN_POINT('Ctrl Pts',(0.322607334643781,-3.2069687136015,56.1629735674045));
#20201=CARTESIAN_POINT('Ctrl Pts',(0.236835962114637,-3.21422667775019,
56.1577684634486));
#20202=CARTESIAN_POINT('Ctrl Pts',(0.20188961603973,-3.21661076956348,56.1556333296901));
#20203=CARTESIAN_POINT('Ctrl Pts',(0.130567843740047,-3.22030962469205,
56.1512432720793));
#20204=CARTESIAN_POINT('Ctrl Pts',(0.094195227287036,-3.22157867017424,
56.1489872489192));
#20205=CARTESIAN_POINT('Ctrl Pts',(0.00118407400272861,-3.22324738345739,
56.1431712266743));
#20206=CARTESIAN_POINT('Ctrl Pts',(-0.0554557993264142,-3.22277040920566,
56.1395848593229));
#20207=CARTESIAN_POINT('Ctrl Pts',(-0.238862715804239,-3.21638972139729,
56.1278211027386));
#20208=CARTESIAN_POINT('Ctrl Pts',(-0.365258903978403,-3.2044940322575,
56.1194749953687));
#20209=CARTESIAN_POINT('Ctrl Pts',(-0.490582206601849,-3.18519177775306,
56.1109990110886));
#20210=CARTESIAN_POINT('Origin',(-9.35406549764863E-15,0.,41.4527091182931));
#20211=CARTESIAN_POINT('',(-0.490582094190866,-3.18519179506656,54.6110712720502));
#20212=CARTESIAN_POINT('',(-0.490582094360392,-3.18519179504045,54.8568649631546));
#20213=CARTESIAN_POINT('',(-0.490582094296226,-3.18519179505033,41.4527091182931));
#20214=CARTESIAN_POINT('',(-3.22274988921121,-0.000845038000876335,55.5782875026161));
#20215=CARTESIAN_POINT('Ctrl Pts',(-0.490582094190866,-3.18519179506656,
54.6110712720502));
#20216=CARTESIAN_POINT('Ctrl Pts',(-0.488218115883238,-3.1855558941549,
54.611227721965));
#20217=CARTESIAN_POINT('Ctrl Pts',(-0.485853718871332,-3.18591736356377,
54.6113842388328));
#20218=CARTESIAN_POINT('Ctrl Pts',(-0.351460153215834,-3.20631038479086,
54.6202829572151));
#20219=CARTESIAN_POINT('Ctrl Pts',(-0.218324002549986,-3.21811745328552,
54.6292281850042));
#20220=CARTESIAN_POINT('Ctrl Pts',(0.106064238668979,-3.2266610217964,54.651122488147));
#20221=CARTESIAN_POINT('Ctrl Pts',(0.297058771535315,-3.21470938461955,
54.6641076547093));
#20222=CARTESIAN_POINT('Ctrl Pts',(0.522018803503048,-3.18040096678932,
54.6788384446438));
#20223=CARTESIAN_POINT('Ctrl Pts',(0.558062842856231,-3.17427473015587,
54.6811802521084));
#20224=CARTESIAN_POINT('Ctrl Pts',(0.614871191674995,-3.1636216676205,54.6848338705702));
#20225=CARTESIAN_POINT('Ctrl Pts',(0.635707347140247,-3.15950073048629,
54.6861659607087));
#20226=CARTESIAN_POINT('Ctrl Pts',(0.676629338688906,-3.15098602866014,
54.6887643975192));
#20227=CARTESIAN_POINT('Ctrl Pts',(0.696716634985155,-3.14660550133401,
54.6900313007804));
#20228=CARTESIAN_POINT('Ctrl Pts',(0.7491778894538,-3.1346380312295,54.693320715881));
#20229=CARTESIAN_POINT('Ctrl Pts',(0.781479750868551,-3.12674154523719,
54.6953267815058));
#20230=CARTESIAN_POINT('Ctrl Pts',(0.853668320567097,-3.10790573043213,
54.6997782296994));
#20231=CARTESIAN_POINT('Ctrl Pts',(0.893478717135233,-3.0966956109964,54.7022111589021));
#20232=CARTESIAN_POINT('Ctrl Pts',(1.02254588647406,-3.05765548667885,54.7100593276068));
#20233=CARTESIAN_POINT('Ctrl Pts',(1.11081292321616,-3.02670675312847,54.7153651018596));
#20234=CARTESIAN_POINT('Ctrl Pts',(1.44143606593318,-2.89436590925381,54.7354142972265));
#20235=CARTESIAN_POINT('Ctrl Pts',(1.67239317729549,-2.7673424425744,54.7498808505692));
#20236=CARTESIAN_POINT('Ctrl Pts',(1.92670902215607,-2.58389379516368,54.7684109264884));
#20237=CARTESIAN_POINT('Ctrl Pts',(1.96732617105176,-2.55310440683157,54.7714555112382));
#20238=CARTESIAN_POINT('Ctrl Pts',(2.03458496251802,-2.49956141516522,54.7766542789936));
#20239=CARTESIAN_POINT('Ctrl Pts',(2.06161727853339,-2.47731251277647,54.7787884994527));
#20240=CARTESIAN_POINT('Ctrl Pts',(2.11601605908315,-2.43103261822754,54.783179005822));
#20241=CARTESIAN_POINT('Ctrl Pts',(2.14334828081445,-2.40696936587802,54.7854364297395));
#20242=CARTESIAN_POINT('Ctrl Pts',(2.21221951650372,-2.34423185932014,54.7912612898189));
#20243=CARTESIAN_POINT('Ctrl Pts',(2.25315393433647,-2.30491537869107,54.7948552562641));
#20244=CARTESIAN_POINT('Ctrl Pts',(2.40874120755135,-2.14737091506546,54.8090500962703));
#20245=CARTESIAN_POINT('Ctrl Pts',(2.5152899636175,-2.02151923606187,54.8199723345397));
#20246=CARTESIAN_POINT('Ctrl Pts',(2.73021884882513,-1.72421430528529,54.8446626096796));
#20247=CARTESIAN_POINT('Ctrl Pts',(2.83300785689257,-1.54954281128614,54.8584657211345));
#20248=CARTESIAN_POINT('Ctrl Pts',(2.93722615732429,-1.32692078660549,54.8744817813078));
#20249=CARTESIAN_POINT('Ctrl Pts',(2.95489954742953,-1.28708405060101,54.8772888476052));
#20250=CARTESIAN_POINT('Ctrl Pts',(2.98052022963348,-1.22602174445777,54.8814899085258));
#20251=CARTESIAN_POINT('Ctrl Pts',(2.98906003671107,-1.20505200055721,54.8829147095781));
#20252=CARTESIAN_POINT('Ctrl Pts',(3.00466203717626,-1.16555422660129,54.8855626242622));
#20253=CARTESIAN_POINT('Ctrl Pts',(3.01177528816914,-1.14704849148357,54.886788403533));
#20254=CARTESIAN_POINT('Ctrl Pts',(3.02893398960021,-1.10114836536465,54.889794254239));
#20255=CARTESIAN_POINT('Ctrl Pts',(3.03877926878053,-1.07368036595767,54.8915631270241));
#20256=CARTESIAN_POINT('Ctrl Pts',(3.07778227376683,-0.960026748210863,
54.8987741659585));
#20257=CARTESIAN_POINT('Ctrl Pts',(3.10365925895005,-0.872752596838835,
54.9040582613079));
#20258=CARTESIAN_POINT('Ctrl Pts',(3.177701441098,-0.577731922154442,54.9214352989276));
#20259=CARTESIAN_POINT('Ctrl Pts',(3.20895147900944,-0.366329106762467,
54.9331324619785));
#20260=CARTESIAN_POINT('Ctrl Pts',(3.22444208500906,-0.0412225616575212,
54.9516571341262));
#20261=CARTESIAN_POINT('Ctrl Pts',(3.22392043589067,0.0711311809176215,
54.958148622425));
#20262=CARTESIAN_POINT('Ctrl Pts',(3.21515817504531,0.225004222129187,54.967299187262));
#20263=CARTESIAN_POINT('Ctrl Pts',(3.21196533500696,0.266734771071235,54.9698067678853));
#20264=CARTESIAN_POINT('Ctrl Pts',(3.2046306230547,0.343032554627598,54.9744454551272));
#20265=CARTESIAN_POINT('Ctrl Pts',(3.20073950528671,0.377617844704507,54.9765685412857));
#20266=CARTESIAN_POINT('Ctrl Pts',(3.19158941898791,0.448581270669863,54.980969879876));
#20267=CARTESIAN_POINT('Ctrl Pts',(3.18626669841827,0.484945899457673,54.9832498333774));
#20268=CARTESIAN_POINT('Ctrl Pts',(3.17085844146737,0.578964055487841,54.9892113601973));
#20269=CARTESIAN_POINT('Ctrl Pts',(3.15982253884326,0.636445952793806,54.9929219746265));
#20270=CARTESIAN_POINT('Ctrl Pts',(3.13182434411174,0.763489837621306,55.0012740666996));
#20271=CARTESIAN_POINT('Ctrl Pts',(3.11409697861974,0.83285011229521,55.0059364133257));
#20272=CARTESIAN_POINT('Ctrl Pts',(3.04477199207156,1.07076776055898,55.0222720414879));
#20273=CARTESIAN_POINT('Ctrl Pts',(2.9816728753774,1.23563686823562,55.0342182951517));
#20274=CARTESIAN_POINT('Ctrl Pts',(2.84655902074834,1.51714327284305,55.0552756732612));
#20275=CARTESIAN_POINT('Ctrl Pts',(2.77998623611765,1.63594168325348,55.0643847445945));
#20276=CARTESIAN_POINT('Ctrl Pts',(2.68868265146704,1.77711326759151,55.0752135535526));
#20277=CARTESIAN_POINT('Ctrl Pts',(2.67086528292944,1.80378069270038,55.0772590136826));
#20278=CARTESIAN_POINT('Ctrl Pts',(2.64224617140743,1.84526108952761,55.0804350436958));
#20279=CARTESIAN_POINT('Ctrl Pts',(2.63171154252255,1.86025474453597,55.0815818802716));
#20280=CARTESIAN_POINT('Ctrl Pts',(2.60889596721909,1.89214578661093,55.0840171978852));
#20281=CARTESIAN_POINT('Ctrl Pts',(2.59657737887008,1.90901540513135,55.0853030019798));
#20282=CARTESIAN_POINT('Ctrl Pts',(2.56326421694991,1.95371681027129,55.0887071220249));
#20283=CARTESIAN_POINT('Ctrl Pts',(2.54198005792617,1.98133046896721,55.0908067924381));
#20284=CARTESIAN_POINT('Ctrl Pts',(2.49278897680459,2.04305217090431,55.0955063593431));
#20285=CARTESIAN_POINT('Ctrl Pts',(2.46462185836465,2.07694450967805,55.0980915619189));
#20286=CARTESIAN_POINT('Ctrl Pts',(2.36746817842859,2.18908466427151,55.1067014214772));
#20287=CARTESIAN_POINT('Ctrl Pts',(2.29537802043148,2.26456163854045,55.1125927844746));
#20288=CARTESIAN_POINT('Ctrl Pts',(2.04679223468783,2.5007349834269,55.1318464105637));
#20289=CARTESIAN_POINT('Ctrl Pts',(1.85613950081233,2.6453299153189,55.1450636770429));
#20290=CARTESIAN_POINT('Ctrl Pts',(1.60459149852999,2.79541763769887,55.1623181247083));
#20291=CARTESIAN_POINT('Ctrl Pts',(1.55720566281375,2.82208852818438,55.165557646386));
#20292=CARTESIAN_POINT('Ctrl Pts',(1.47738802898349,2.86439103105369,55.1710103759082));
#20293=CARTESIAN_POINT('Ctrl Pts',(1.44532749154622,2.88070124249163,55.1731994967862));
#20294=CARTESIAN_POINT('Ctrl Pts',(1.38084303808594,2.91215905463831,55.1776038667476));
#20295=CARTESIAN_POINT('Ctrl Pts',(1.34842647043407,2.92730998463742,55.1798186071413));
#20296=CARTESIAN_POINT('Ctrl Pts',(1.26707330265888,2.96369498773936,55.1853813329415));
#20297=CARTESIAN_POINT('Ctrl Pts',(1.21785056105438,2.98425907190415,55.1887512322334));
#20298=CARTESIAN_POINT('Ctrl Pts',(1.00023236152541,3.0688941050392,55.2036758173797));
#20299=CARTESIAN_POINT('Ctrl Pts',(0.82716517735864,3.11999313967493,55.2156371047934));
#20300=CARTESIAN_POINT('Ctrl Pts',(0.44563305019645,3.19865504127307,55.2418828576738));
#20301=CARTESIAN_POINT('Ctrl Pts',(0.236862671107257,3.22085221301945,55.2561720757712));
#20302=CARTESIAN_POINT('Ctrl Pts',(-0.00720010715993356,3.22292776502206,
55.2719388574884));
#20303=CARTESIAN_POINT('Ctrl Pts',(-0.0418101800208314,3.22266463527656,
55.2741518324622));
#20304=CARTESIAN_POINT('Ctrl Pts',(-0.0972398023030859,3.2213500387901,
55.2776524036174));
#20305=CARTESIAN_POINT('Ctrl Pts',(-0.11806418050657,3.22065405773964,55.2789576628939));
#20306=CARTESIAN_POINT('Ctrl Pts',(-0.159784173360221,3.21885450656175,
55.2815508983957));
#20307=CARTESIAN_POINT('Ctrl Pts',(-0.180678702375732,3.21774930334034,
55.2828387307623));
#20308=CARTESIAN_POINT('Ctrl Pts',(-0.236523009938695,3.21424976080671,
55.2862549481559));
#20309=CARTESIAN_POINT('Ctrl Pts',(-0.271447932757623,3.21148889198248,
55.2883644532032));
#20310=CARTESIAN_POINT('Ctrl Pts',(-0.467659118559107,3.19275419284158,
55.300098298393));
#20311=CARTESIAN_POINT('Ctrl Pts',(-0.627622114528567,3.16519922858504,
55.3092240629311));
#20312=CARTESIAN_POINT('Ctrl Pts',(-0.998528769734702,3.07206715490697,
55.3306661321348));
#20313=CARTESIAN_POINT('Ctrl Pts',(-1.20612623910482,2.99664915791563,55.3429263936251));
#20314=CARTESIAN_POINT('Ctrl Pts',(-1.45519184959555,2.8760595511611,55.3591973130293));
#20315=CARTESIAN_POINT('Ctrl Pts',(-1.5053244718323,2.85014026515908,55.3625545474207));
#20316=CARTESIAN_POINT('Ctrl Pts',(-1.5865921549261,2.8053813435495,55.3681491350678));
#20317=CARTESIAN_POINT('Ctrl Pts',(-1.61813548670954,2.78730632152881,55.3703595700089));
#20318=CARTESIAN_POINT('Ctrl Pts',(-1.67983096543237,2.75055322182661,55.3747642135771));
#20319=CARTESIAN_POINT('Ctrl Pts',(-1.70999393280832,2.73190330900102,55.3769571843854));
#20320=CARTESIAN_POINT('Ctrl Pts',(-1.7832308407509,2.68493245518761,55.3823826924286));
#20321=CARTESIAN_POINT('Ctrl Pts',(-1.8259435900971,2.65606928378936,55.3856348208993));
#20322=CARTESIAN_POINT('Ctrl Pts',(-1.91699804750518,2.59130463791565,55.3927650003643));
#20323=CARTESIAN_POINT('Ctrl Pts',(-1.96506230900659,2.5550480704773,55.3966551219498));
#20324=CARTESIAN_POINT('Ctrl Pts',(-2.10991110106341,2.4392780155006,55.4087724047032));
#20325=CARTESIAN_POINT('Ctrl Pts',(-2.20309280971632,2.35545741010476,55.4171380706289));
#20326=CARTESIAN_POINT('Ctrl Pts',(-2.43713927062181,2.11885818303161,55.439563752036));
#20327=CARTESIAN_POINT('Ctrl Pts',(-2.56853123956947,1.95751502339181,55.4537213442129));
#20328=CARTESIAN_POINT('Ctrl Pts',(-2.70277920996137,1.75565220021036,55.4693856091766));
#20329=CARTESIAN_POINT('Ctrl Pts',(-2.72159191814923,1.72634520396884,55.471612745882));
#20330=CARTESIAN_POINT('Ctrl Pts',(-2.75091945432572,1.67898649887106,55.4751301590685));
#20331=CARTESIAN_POINT('Ctrl Pts',(-2.7617397357215,1.6611282900715,55.4764383782975));
#20332=CARTESIAN_POINT('Ctrl Pts',(-2.78303070629782,1.62520568494068,55.4790318885782));
#20333=CARTESIAN_POINT('Ctrl Pts',(-2.7935009461426,1.60714216865211,55.4803171198939));
#20334=CARTESIAN_POINT('Ctrl Pts',(-2.82095965793227,1.55869050692258,55.4837178237241));
#20335=CARTESIAN_POINT('Ctrl Pts',(-2.83763298748904,1.52812589044978,55.48581471675));
#20336=CARTESIAN_POINT('Ctrl Pts',(-2.92810354252212,1.35569125747713,55.4974102114491));
#20337=CARTESIAN_POINT('Ctrl Pts',(-2.99176434782105,1.20873743676747,55.506422547652));
#20338=CARTESIAN_POINT('Ctrl Pts',(-3.11764965582723,0.84639941413445,55.5279344931588));
#20339=CARTESIAN_POINT('Ctrl Pts',(-3.16884980097137,0.628102370317696,
55.5403697591376));
#20340=CARTESIAN_POINT('Ctrl Pts',(-3.20397397894642,0.35170175904735,55.5567576483647));
#20341=CARTESIAN_POINT('Ctrl Pts',(-3.20950983955604,0.296967088794769,
55.5600304232696));
#20342=CARTESIAN_POINT('Ctrl Pts',(-3.21638275917703,0.205743228111225,
55.5655451551488));
#20343=CARTESIAN_POINT('Ctrl Pts',(-3.21850548643902,0.169323938624154,
55.567762617296));
#20344=CARTESIAN_POINT('Ctrl Pts',(-3.22098376837375,0.109267967967994,
55.5714483292774));
#20345=CARTESIAN_POINT('Ctrl Pts',(-3.22169833283886,0.0856488782510573,
55.5729052527132));
#20346=CARTESIAN_POINT('Ctrl Pts',(-3.22255645023745,0.0410699880881085,
55.5756697160235));
#20347=CARTESIAN_POINT('Ctrl Pts',(-3.22275538448412,0.0201124694179753,
55.5769754575503));
#20348=CARTESIAN_POINT('Ctrl Pts',(-3.22274988921121,-0.000845038000876335,
55.5782875026161));
#20349=CARTESIAN_POINT('Ctrl Pts',(-3.2227498896419,-0.000843393838916127,
55.5782873996834));
#20350=CARTESIAN_POINT('Ctrl Pts',(-3.22274288764006,-0.0275992220640488,
55.5799624482896));
#20351=CARTESIAN_POINT('Ctrl Pts',(-3.2224026891714,-0.0543534235100241,
55.5816476755399));
#20352=CARTESIAN_POINT('Ctrl Pts',(-3.22071865370461,-0.121252538950575,
55.5858879877087));
#20353=CARTESIAN_POINT('Ctrl Pts',(-3.2189573858021,-0.161381378275452,
55.5884553222044));
#20354=CARTESIAN_POINT('Ctrl Pts',(-3.20369698711565,-0.40501746016145,
55.6041886682182));
#20355=CARTESIAN_POINT('Ctrl Pts',(-3.17165512760259,-0.606874403716984,
55.6178876259209));
#20356=CARTESIAN_POINT('Ctrl Pts',(-3.07882886738486,-0.9670399381762,55.6430118722649));
#20357=CARTESIAN_POINT('Ctrl Pts',(-3.02422566227135,-1.1262423935776,55.6543629498995));
#20358=CARTESIAN_POINT('Ctrl Pts',(-2.94421363512423,-1.3110429138473,55.6673528114193));
#20359=CARTESIAN_POINT('Ctrl Pts',(-2.9305029700883,-1.34140970404138,55.6694804781047));
#20360=CARTESIAN_POINT('Ctrl Pts',(-2.90756845006362,-1.39017496879325,
55.6728798093302));
#20361=CARTESIAN_POINT('Ctrl Pts',(-2.898635233766,-1.40870670787885,55.6741674727357));
#20362=CARTESIAN_POINT('Ctrl Pts',(-2.88012690263248,-1.44618012740074,
55.6767609413572));
#20363=CARTESIAN_POINT('Ctrl Pts',(-2.87054099256361,-1.4651151505743,55.6780660647625));
#20364=CARTESIAN_POINT('Ctrl Pts',(-2.8439724507588,-1.51633399517883,55.6815855398929));
#20365=CARTESIAN_POINT('Ctrl Pts',(-2.8266271669469,-1.54842732962711,55.6837789652586));
#20366=CARTESIAN_POINT('Ctrl Pts',(-2.7145897948392,-1.74756649714963,55.697357630424));
#20367=CARTESIAN_POINT('Ctrl Pts',(-2.60566127469289,-1.9061826603677,55.7080484664413));
#20368=CARTESIAN_POINT('Ctrl Pts',(-2.35937874486132,-2.20390894904481,
55.7296939621426));
#20369=CARTESIAN_POINT('Ctrl Pts',(-2.22223501455478,-2.34212389944741,
55.7406156173946));
#20370=CARTESIAN_POINT('Ctrl Pts',(-2.03273493147719,-2.50138757836204,
55.7552119021853));
#20371=CARTESIAN_POINT('Ctrl Pts',(-1.99114402250642,-2.53461952182791,
55.7583862970687));
#20372=CARTESIAN_POINT('Ctrl Pts',(-1.92026818942323,-2.58842935473143,
55.7637609130451));
#20373=CARTESIAN_POINT('Ctrl Pts',(-1.8914284429096,-2.60957750047474,55.7659385696278));
#20374=CARTESIAN_POINT('Ctrl Pts',(-1.83286989453582,-2.65103769142701,
55.7703452258239));
#20375=CARTESIAN_POINT('Ctrl Pts',(-1.80315084620381,-2.67134044096244,
55.7725741488184));
#20376=CARTESIAN_POINT('Ctrl Pts',(-1.72760165192969,-2.72111717745418,
55.77822470734));
#20377=CARTESIAN_POINT('Ctrl Pts',(-1.68135385394976,-2.74993360047054,
55.7816697758867));
#20378=CARTESIAN_POINT('Ctrl Pts',(-1.42952675426891,-2.89811611484992,
55.8003649843496));
#20379=CARTESIAN_POINT('Ctrl Pts',(-1.21197332966864,-2.99561514582695,
55.8163704929202));
#20380=CARTESIAN_POINT('Ctrl Pts',(-0.886011331371105,-3.100333893371,55.8394895939961));
#20381=CARTESIAN_POINT('Ctrl Pts',(-0.784791778974033,-3.12748943776473,
55.8465437945079));
#20382=CARTESIAN_POINT('Ctrl Pts',(-0.639262530915241,-3.15902065320963,
55.8563762400436));
#20383=CARTESIAN_POINT('Ctrl Pts',(-0.595909771719696,-3.16748480194819,
55.8592666350033));
#20384=CARTESIAN_POINT('Ctrl Pts',(-0.531824175297743,-3.17863438760384,
55.863470131914));
#20385=CARTESIAN_POINT('Ctrl Pts',(-0.511218946646582,-3.18201331447733,
55.8648111988455));
#20386=CARTESIAN_POINT('Ctrl Pts',(-0.490582094113513,-3.18519179507847,
55.8661429281184));
#20387=CARTESIAN_POINT('',(-3.22274963550475,-0.0023652837118349,55.8259788468706));
#20388=CARTESIAN_POINT('Ctrl Pts',(-0.49058220660185,-3.18519177775306,
56.1109990110886));
#20389=CARTESIAN_POINT('Ctrl Pts',(-0.527035938123794,-3.17957718582367,
56.1085335377979));
#20390=CARTESIAN_POINT('Ctrl Pts',(-0.563398927501597,-3.17333592017435,
56.1060575984741));
#20391=CARTESIAN_POINT('Ctrl Pts',(-0.796465884766915,-3.12919850823935,
56.0900953600583));
#20392=CARTESIAN_POINT('Ctrl Pts',(-0.989378531457401,-3.0736586133384,
56.0764232066526));
#20393=CARTESIAN_POINT('Ctrl Pts',(-1.2182107367988,-2.98398159018331,56.0603845464486));
#20394=CARTESIAN_POINT('Ctrl Pts',(-1.26017687552495,-2.96650269469745,
56.0574525416929));
#20395=CARTESIAN_POINT('Ctrl Pts',(-1.32279957160357,-2.93885143421542,
56.053106105014));
#20396=CARTESIAN_POINT('Ctrl Pts',(-1.3437383898767,-2.92933672895247,56.0516577533548));
#20397=CARTESIAN_POINT('Ctrl Pts',(-1.38244238719976,-2.91124709052142,
56.0489922228911));
#20398=CARTESIAN_POINT('Ctrl Pts',(-1.40023254369973,-2.90273240534161,
56.0477719377583));
#20399=CARTESIAN_POINT('Ctrl Pts',(-1.44349863930908,-2.88153413959549,
56.0448144440116));
#20400=CARTESIAN_POINT('Ctrl Pts',(-1.4688866149837,-2.86867557584027,56.0430875900951));
#20401=CARTESIAN_POINT('Ctrl Pts',(-1.56820833451165,-2.81670649430969,
56.0363528461759));
#20402=CARTESIAN_POINT('Ctrl Pts',(-1.64078337656342,-2.77505766260991,
56.0314777162139));
#20403=CARTESIAN_POINT('Ctrl Pts',(-1.85995454523111,-2.63767291986913,
56.0166480833059));
#20404=CARTESIAN_POINT('Ctrl Pts',(-2.0004349232622,-2.53278794508391,56.006974110287));
#20405=CARTESIAN_POINT('Ctrl Pts',(-2.24541729786842,-2.31672312410082,
55.9885819914824));
#20406=CARTESIAN_POINT('Ctrl Pts',(-2.35189683224743,-2.20854688599951,
55.9799334391777));
#20407=CARTESIAN_POINT('Ctrl Pts',(-2.48261416030586,-2.05553158101331,
55.9680256366292));
#20408=CARTESIAN_POINT('Ctrl Pts',(-2.51398831649961,-2.01703879449303,
55.9650559859045));
#20409=CARTESIAN_POINT('Ctrl Pts',(-2.56581365002936,-1.95036626671955,
55.9599453173604));
#20410=CARTESIAN_POINT('Ctrl Pts',(-2.58672080573658,-1.92255132255864,
55.9578226057174));
#20411=CARTESIAN_POINT('Ctrl Pts',(-2.62878586494356,-1.86465930245229,
55.953420526404));
#20412=CARTESIAN_POINT('Ctrl Pts',(-2.64988747072764,-1.83454780620086,
55.9511394322938));
#20413=CARTESIAN_POINT('Ctrl Pts',(-2.7032776208159,-1.75551777622357,55.9451713118334));
#20414=CARTESIAN_POINT('Ctrl Pts',(-2.7347538836124,-1.7060694726035,55.9414551235481));
#20415=CARTESIAN_POINT('Ctrl Pts',(-2.80170958235842,-1.59426604139773,
55.9330879108246));
#20416=CARTESIAN_POINT('Ctrl Pts',(-2.83648992433679,-1.53153013190146,
55.9284158944086));
#20417=CARTESIAN_POINT('Ctrl Pts',(-2.88940044191937,-1.42809679512133,
55.9207565769007));
#20418=CARTESIAN_POINT('Ctrl Pts',(-2.90883162626377,-1.38808995565332,
55.9178043519347));
#20419=CARTESIAN_POINT('Ctrl Pts',(-3.02222465732457,-1.14178053141678,
55.8997066447939));
#20420=CARTESIAN_POINT('Ctrl Pts',(-3.09502800721153,-0.926446943796116,
55.8841573814485));
#20421=CARTESIAN_POINT('Ctrl Pts',(-3.15710934938906,-0.649636544659183,
55.8654938365189));
#20422=CARTESIAN_POINT('Ctrl Pts',(-3.16810694615104,-0.593688732898751,
55.8617902145876));
#20423=CARTESIAN_POINT('Ctrl Pts',(-3.18178388576271,-0.512829088650184,
55.8565624849481));
#20424=CARTESIAN_POINT('Ctrl Pts',(-3.18566590138256,-0.488134434512769,
55.8549825768815));
#20425=CARTESIAN_POINT('Ctrl Pts',(-3.19206108095442,-0.444120497028435,
55.8521991974741));
#20426=CARTESIAN_POINT('Ctrl Pts',(-3.19468695256116,-0.424820289713105,
55.8509900062762));
#20427=CARTESIAN_POINT('Ctrl Pts',(-3.19954298916008,-0.38653279932615,
55.84861325251));
#20428=CARTESIAN_POINT('Ctrl Pts',(-3.20177939753818,-0.36754819363111,
55.8474452333136));
#20429=CARTESIAN_POINT('Ctrl Pts',(-3.20662700924488,-0.322988561302356,
55.84472592308));
#20430=CARTESIAN_POINT('Ctrl Pts',(-3.20910142055447,-0.297399641046346,
55.8431814292897));
#20431=CARTESIAN_POINT('Ctrl Pts',(-3.21885286366528,-0.182180850534396,
55.8362930114648));
#20432=CARTESIAN_POINT('Ctrl Pts',(-3.22268324456027,-0.0922947409880173,
55.8310977937728));
#20433=CARTESIAN_POINT('Ctrl Pts',(-3.22274913503596,-0.00236117027106857,
55.8259777403464));
#20434=CARTESIAN_POINT('Ctrl Pts',(-3.22274913198354,-0.0023653328352537,
55.8259779773275));
#20435=CARTESIAN_POINT('Ctrl Pts',(-3.2228229772883,0.0982483686585223,
55.8202498852851));
#20436=CARTESIAN_POINT('Ctrl Pts',(-3.21818507087071,0.198815352652257,
55.8146211056984));
#20437=CARTESIAN_POINT('Ctrl Pts',(-3.1899723467413,0.501587428547368,55.7975878224515));
#20438=CARTESIAN_POINT('Ctrl Pts',(-3.15195669874257,0.7019056765601,55.7861689506042));
#20439=CARTESIAN_POINT('Ctrl Pts',(-3.08100654171627,0.946655981404647,
55.771116825202));
#20440=CARTESIAN_POINT('Ctrl Pts',(-3.06551922547341,0.995665757241424,
55.7680475947046));
#20441=CARTESIAN_POINT('Ctrl Pts',(-3.03738470469542,1.07780678037972,55.7627982896777));
#20442=CARTESIAN_POINT('Ctrl Pts',(-3.02535030728503,1.11113845408135,55.7606383831365));
#20443=CARTESIAN_POINT('Ctrl Pts',(-2.99984781661115,1.17828477790705,55.7562232213153));
#20444=CARTESIAN_POINT('Ctrl Pts',(-2.9863516480399,1.21208316678579,55.7539672903639));
#20445=CARTESIAN_POINT('Ctrl Pts',(-2.95039889775408,1.29787157203897,55.7481518282855));
#20446=CARTESIAN_POINT('Ctrl Pts',(-2.92713978260316,1.34950966125318,55.7445659390009));
#20447=CARTESIAN_POINT('Ctrl Pts',(-2.80775960541484,1.59692382822402,55.72695676684));
#20448=CARTESIAN_POINT('Ctrl Pts',(-2.69330580822685,1.78318728664743,55.7123201359199));
#20449=CARTESIAN_POINT('Ctrl Pts',(-2.45953151085422,2.08919383284132,55.6863076360253));
#20450=CARTESIAN_POINT('Ctrl Pts',(-2.34793756856334,2.21387094349798,55.6750248556402));
#20451=CARTESIAN_POINT('Ctrl Pts',(-2.20304183693845,2.35241125151116,55.6620925586476));
#20452=CARTESIAN_POINT('Ctrl Pts',(-2.17855464697723,2.37510670989627,55.6599603613078));
#20453=CARTESIAN_POINT('Ctrl Pts',(-2.13840448373938,2.41117556174831,55.6565556302991));
#20454=CARTESIAN_POINT('Ctrl Pts',(-2.12295873902952,2.42478609140215,55.6552670106535));
#20455=CARTESIAN_POINT('Ctrl Pts',(-2.09133894538991,2.45211514403191,55.6526735279007));
#20456=CARTESIAN_POINT('Ctrl Pts',(-2.07515791596265,2.46582378650117,55.6513693174119));
#20457=CARTESIAN_POINT('Ctrl Pts',(-2.03084080818286,2.50262420511306,55.6478554726257));
#20458=CARTESIAN_POINT('Ctrl Pts',(-2.00244616786446,2.52540133324973,55.6456666498142));
#20459=CARTESIAN_POINT('Ctrl Pts',(-1.82112306513656,2.66587036417349,55.632034669634));
#20460=CARTESIAN_POINT('Ctrl Pts',(-1.65825209483043,2.77012108498177,55.6212937401246));
#20461=CARTESIAN_POINT('Ctrl Pts',(-1.31375262187064,2.94929002360706,55.599540367835));
#20462=CARTESIAN_POINT('Ctrl Pts',(-1.13267591374804,3.02345707916979,55.5885612852658));
#20463=CARTESIAN_POINT('Ctrl Pts',(-0.895906682083919,3.0961614568649,55.5739454656203));
#20464=CARTESIAN_POINT('Ctrl Pts',(-0.845438308573807,3.11032123045247,
55.5708179555036));
#20465=CARTESIAN_POINT('Ctrl Pts',(-0.760133394249979,3.13202542171231,
55.5654992995984));
#20466=CARTESIAN_POINT('Ctrl Pts',(-0.72547558018151,3.14023423417916,55.5633296399231));
#20467=CARTESIAN_POINT('Ctrl Pts',(-0.655369501236063,3.15561657494592,
55.558919855515));
#20468=CARTESIAN_POINT('Ctrl Pts',(-0.619922391875828,3.16277112843798,
55.5566794803967));
#20469=CARTESIAN_POINT('Ctrl Pts',(-0.529887102066823,3.17937191761829,
55.5509589283532));
#20470=CARTESIAN_POINT('Ctrl Pts',(-0.475163652542741,3.18800957248449,
55.5474540904453));
#20471=CARTESIAN_POINT('Ctrl Pts',(-0.16699929074674,3.22854035184702,55.5275512141267));
#20472=CARTESIAN_POINT('Ctrl Pts',(0.0892767622137504,3.23161726034424,
55.510268933566));
#20473=CARTESIAN_POINT('Ctrl Pts',(0.43467214958567,3.19462763151725,55.4868460016672));
#20474=CARTESIAN_POINT('Ctrl Pts',(0.525713846636263,3.18091373893239,55.4806717228103));
#20475=CARTESIAN_POINT('Ctrl Pts',(0.656262508258042,3.15548976322421,55.4719142417823));
#20476=CARTESIAN_POINT('Ctrl Pts',(0.696326090455761,3.14689154512072,55.4692401943707));
#20477=CARTESIAN_POINT('Ctrl Pts',(0.768362834847134,3.12998824302095,55.4644689102693));
#20478=CARTESIAN_POINT('Ctrl Pts',(0.800392813565002,3.12195121473609,55.4623607446143));
#20479=CARTESIAN_POINT('Ctrl Pts',(0.852111900807501,3.10812542289005,55.4589844560805));
#20480=CARTESIAN_POINT('Ctrl Pts',(0.87187861437407,3.10263856929728,55.4577007106795));
#20481=CARTESIAN_POINT('Ctrl Pts',(0.912060380634412,3.09107053977376,55.4551065589134));
#20482=CARTESIAN_POINT('Ctrl Pts',(0.932470028740062,3.08497502811768,55.453796966314));
#20483=CARTESIAN_POINT('Ctrl Pts',(0.988019647061457,3.0677830033401,55.450250902765));
#20484=CARTESIAN_POINT('Ctrl Pts',(1.02303313710983,3.05628513662685,55.4480358972749));
#20485=CARTESIAN_POINT('Ctrl Pts',(1.23249066356965,2.98349948840664,55.4348640724989));
#20486=CARTESIAN_POINT('Ctrl Pts',(1.40161133343692,2.90788637419721,55.4245466315709));
#20487=CARTESIAN_POINT('Ctrl Pts',(1.74279660810602,2.71862062998475,55.4026916864046));
#20488=CARTESIAN_POINT('Ctrl Pts',(1.91232651738564,2.6021595600219,55.3911777956687));
#20489=CARTESIAN_POINT('Ctrl Pts',(2.10887186918008,2.43749837051577,55.3760295996038));
#20490=CARTESIAN_POINT('Ctrl Pts',(2.14732705043697,2.40368986655771,55.3729715248353));
#20491=CARTESIAN_POINT('Ctrl Pts',(2.21098293632375,2.34497875631701,55.3677354533713));
#20492=CARTESIAN_POINT('Ctrl Pts',(2.23660864693423,2.32055004663294,55.3655773749361));
#20493=CARTESIAN_POINT('Ctrl Pts',(2.28778336730374,2.27013053808316,55.3611609429905));
#20494=CARTESIAN_POINT('Ctrl Pts',(2.31330426221159,2.24411867192428,55.3589018296224));
#20495=CARTESIAN_POINT('Ctrl Pts',(2.37751820064189,2.17640988789781,55.3530670147389));
#20496=CARTESIAN_POINT('Ctrl Pts',(2.41555701762706,2.13411256500581,55.3494646047582));
#20497=CARTESIAN_POINT('Ctrl Pts',(2.61821643490829,1.89640199489849,55.3294369328708));
#20498=CARTESIAN_POINT('Ctrl Pts',(2.76024606778113,1.68297327409865,55.3121342896196));
#20499=CARTESIAN_POINT('Ctrl Pts',(2.91623504233318,1.37470120936979,55.2888458395013));
#20500=CARTESIAN_POINT('Ctrl Pts',(2.95351678504418,1.2926602276134,55.2828064878133));
#20501=CARTESIAN_POINT('Ctrl Pts',(3.00892371422408,1.15577371167581,55.2730875351161));
#20502=CARTESIAN_POINT('Ctrl Pts',(3.0290996503226,1.10181258479639,55.2693442976301));
#20503=CARTESIAN_POINT('Ctrl Pts',(3.05597322053875,1.02360867522688,55.2640720573803));
#20504=CARTESIAN_POINT('Ctrl Pts',(3.06384979676633,0.999785757031245,55.2624860096359));
#20505=CARTESIAN_POINT('Ctrl Pts',(3.07676210538083,0.959145732012153,55.2598170805789));
#20506=CARTESIAN_POINT('Ctrl Pts',(3.08193979420671,0.942376109745944,55.258726474967));
#20507=CARTESIAN_POINT('Ctrl Pts',(3.0939773524714,0.902227920664037,55.2561408859006));
#20508=CARTESIAN_POINT('Ctrl Pts',(3.10070950966011,0.878812664418354,55.2546530341183));
#20509=CARTESIAN_POINT('Ctrl Pts',(3.12127516616435,0.80410270538572,55.2499630077144));
#20510=CARTESIAN_POINT('Ctrl Pts',(3.13410683553579,0.752538939672678,55.2468112067589));
#20511=CARTESIAN_POINT('Ctrl Pts',(3.18759408098974,0.512410811455773,55.2324271559637));
#20512=CARTESIAN_POINT('Ctrl Pts',(3.2125468570552,0.320742991126696,55.2217580674986));
#20513=CARTESIAN_POINT('Ctrl Pts',(3.22657771771426,-0.0322955815934162,
55.2019281767073));
#20514=CARTESIAN_POINT('Ctrl Pts',(3.22097258947683,-0.19280949751601,55.1928455629736));
#20515=CARTESIAN_POINT('Ctrl Pts',(3.19730343434968,-0.408074149992268,
55.1801092845613));
#20516=CARTESIAN_POINT('Ctrl Pts',(3.18970435823871,-0.463744878929698,
55.1767663020544));
#20517=CARTESIAN_POINT('Ctrl Pts',(3.1748053402836,-0.555019696872055,55.1711888647571));
#20518=CARTESIAN_POINT('Ctrl Pts',(3.16835121267288,-0.590750574196046,
55.1689809788493));
#20519=CARTESIAN_POINT('Ctrl Pts',(3.15447562094606,-0.66078151366893,55.1646017117433));
#20520=CARTESIAN_POINT('Ctrl Pts',(3.14709484965502,-0.695084531290105,
55.1624318961566));
#20521=CARTESIAN_POINT('Ctrl Pts',(3.12752203686441,-0.779337303921066,
55.1570385276832));
#20522=CARTESIAN_POINT('Ctrl Pts',(3.11469227106025,-0.829127432213722,
55.1537951924818));
#20523=CARTESIAN_POINT('Ctrl Pts',(3.02989180791858,-1.12840210429823,55.1339486834457));
#20524=CARTESIAN_POINT('Ctrl Pts',(2.929184546471,-1.36871056398113,55.1164078666076));
#20525=CARTESIAN_POINT('Ctrl Pts',(2.73194841900223,-1.71520681340992,55.0895126245274));
#20526=CARTESIAN_POINT('Ctrl Pts',(2.65535275315824,-1.83155271109945,55.0801878383818));
#20527=CARTESIAN_POINT('Ctrl Pts',(2.55212101470315,-1.96820381127954,55.0691565932237));
#20528=CARTESIAN_POINT('Ctrl Pts',(2.53239003932206,-1.99352672076478,55.0671091302164));
#20529=CARTESIAN_POINT('Ctrl Pts',(2.49954757192841,-2.03440235382374,55.0638044637458));
#20530=CARTESIAN_POINT('Ctrl Pts',(2.48666168770702,-2.05013285725691,55.0625327980774));
#20531=CARTESIAN_POINT('Ctrl Pts',(2.45981008772527,-2.08228637545829,55.0599354361305));
#20532=CARTESIAN_POINT('Ctrl Pts',(2.44582696565218,-2.09869310092674,55.0586109842135));
#20533=CARTESIAN_POINT('Ctrl Pts',(2.40667549163683,-2.14370761774219,55.0549756299731));
#20534=CARTESIAN_POINT('Ctrl Pts',(2.38116207566722,-2.17201213709358,55.0526880484139));
#20535=CARTESIAN_POINT('Ctrl Pts',(2.23561226365501,-2.32783661269814,55.0400403495102));
#20536=CARTESIAN_POINT('Ctrl Pts',(2.10582737704225,-2.44587192721079,55.0302421907769));
#20537=CARTESIAN_POINT('Ctrl Pts',(1.80158902890794,-2.68030670418677,55.0087267326335));
#20538=CARTESIAN_POINT('Ctrl Pts',(1.62410625321696,-2.7914217267226,54.9970336041673));
#20539=CARTESIAN_POINT('Ctrl Pts',(1.38973372734427,-2.90818868842021,54.9815894440076));
#20540=CARTESIAN_POINT('Ctrl Pts',(1.34176725120063,-2.93062816661406,54.978431124287));
#20541=CARTESIAN_POINT('Ctrl Pts',(1.26056152441024,-2.96620591623068,54.9730756737991));
#20542=CARTESIAN_POINT('Ctrl Pts',(1.22761646392611,-2.97999170372793,54.9709007353649));
#20543=CARTESIAN_POINT('Ctrl Pts',(1.16096893043593,-3.00658746794712,54.9664930099224));
#20544=CARTESIAN_POINT('Ctrl Pts',(1.12726707147582,-3.01938501066424,54.9642601882941));
#20545=CARTESIAN_POINT('Ctrl Pts',(1.0418162491028,-3.0502030482227,54.9585859648373));
#20546=CARTESIAN_POINT('Ctrl Pts',(0.989810825641516,-3.06747350113949,
54.9551207182374));
#20547=CARTESIAN_POINT('Ctrl Pts',(0.692133141392219,-3.15797103863363,
54.9352083142476));
#20548=CARTESIAN_POINT('Ctrl Pts',(0.438886276367857,-3.20299335167178,
54.9178667207973));
#20549=CARTESIAN_POINT('Ctrl Pts',(0.090953146238864,-3.22278640445546,
54.8943671064587));
#20550=CARTESIAN_POINT('Ctrl Pts',(-0.00131923124893615,-3.22406957593432,
54.8881781514758));
#20551=CARTESIAN_POINT('Ctrl Pts',(-0.134532326748332,-3.22020212874891,
54.8794025709591));
#20552=CARTESIAN_POINT('Ctrl Pts',(-0.175516451819975,-3.2182285451047,
54.8767247519752));
#20553=CARTESIAN_POINT('Ctrl Pts',(-0.249431867276678,-3.21325283959648,
54.8719475179539));
#20554=CARTESIAN_POINT('Ctrl Pts',(-0.282375700579359,-3.21052553760741,
54.8698371353294));
#20555=CARTESIAN_POINT('Ctrl Pts',(-0.335694192137568,-3.20528438975017,
54.8664582247901));
#20556=CARTESIAN_POINT('Ctrl Pts',(-0.356096438378675,-3.20308195494703,
54.8651740316997));
#20557=CARTESIAN_POINT('Ctrl Pts',(-0.397621854361298,-3.19819757159231,
54.8625799550361));
#20558=CARTESIAN_POINT('Ctrl Pts',(-0.41874206050948,-3.19550089837726,
54.8612708701532));
#20559=CARTESIAN_POINT('Ctrl Pts',(-0.456769780723612,-3.19026192831209,
54.8589298906642));
#20560=CARTESIAN_POINT('Ctrl Pts',(-0.473686125210811,-3.18779410613033,
54.8578942793142));
#20561=CARTESIAN_POINT('Ctrl Pts',(-0.490582094360392,-3.18519179504045,
54.8568649631546));
#20562=CARTESIAN_POINT('Origin',(-9.35406549764863E-15,0.,41.4527091182931));
#20563=CARTESIAN_POINT('',(-0.490581732222734,-3.18519185081674,53.3621044196136));
#20564=CARTESIAN_POINT('',(-0.490582106922591,-3.18519179310562,53.611790309282));
#20565=CARTESIAN_POINT('',(-0.490582094296226,-3.18519179505033,41.4527091182931));
#20566=CARTESIAN_POINT('Ctrl Pts',(-0.490581732222735,-3.18519185081674,
53.3621044196136));
#20567=CARTESIAN_POINT('Ctrl Pts',(-0.374900299471536,-3.20300905000696,
53.3687345167815));
#20568=CARTESIAN_POINT('Ctrl Pts',(-0.258278326006094,-3.21451969634228,
53.3754616507783));
#20569=CARTESIAN_POINT('Ctrl Pts',(-0.0891756247728096,-3.22193730412938,
53.3854530367755));
#20570=CARTESIAN_POINT('Ctrl Pts',(-0.0370773199011404,-3.22295781912657,
53.3885628761321));
#20571=CARTESIAN_POINT('Ctrl Pts',(0.0505799220086531,-3.22254925724566,
53.3938604005856));
#20572=CARTESIAN_POINT('Ctrl Pts',(0.0861327506792581,-3.22179500239537,
53.3960270005347));
#20573=CARTESIAN_POINT('Ctrl Pts',(0.157864795363987,-3.21908505349894,
53.4004379997426));
#20574=CARTESIAN_POINT('Ctrl Pts',(0.194037966799418,-3.21710723684919,
53.4026827748256));
#20575=CARTESIAN_POINT('Ctrl Pts',(0.285776141534282,-3.21053851694113,
53.4084305618543));
#20576=CARTESIAN_POINT('Ctrl Pts',(0.341267668412837,-3.20511487132255,
53.4119587205782));
#20577=CARTESIAN_POINT('Ctrl Pts',(0.621974377391368,-3.1703068545971,53.4300766347506));
#20578=CARTESIAN_POINT('Ctrl Pts',(0.84374348982526,-3.11861582141513,53.4453425679518));
#20579=CARTESIAN_POINT('Ctrl Pts',(1.20603461255976,-2.99267334392773,53.4712497543564));
#20580=CARTESIAN_POINT('Ctrl Pts',(1.34994018284468,-2.93057720253295,53.4818017772582));
#20581=CARTESIAN_POINT('Ctrl Pts',(1.51992444398366,-2.84203816900848,53.4941898577305));
#20582=CARTESIAN_POINT('Ctrl Pts',(1.55081028912439,-2.82530333740668,53.4964369833841));
#20583=CARTESIAN_POINT('Ctrl Pts',(1.59966518263867,-2.79778974164801,53.4999781652797));
#20584=CARTESIAN_POINT('Ctrl Pts',(1.61781259640974,-2.78733539329653,53.5012905642927));
#20585=CARTESIAN_POINT('Ctrl Pts',(1.65379236625133,-2.76613840555551,53.5038846022821));
#20586=CARTESIAN_POINT('Ctrl Pts',(1.67162508405082,-2.75539842840672,53.5051662926317));
#20587=CARTESIAN_POINT('Ctrl Pts',(1.7187467143476,-2.7263929733806,53.5085458099808));
#20588=CARTESIAN_POINT('Ctrl Pts',(1.74784918788139,-2.70782797559912,53.5106254682423));
#20589=CARTESIAN_POINT('Ctrl Pts',(1.95203358939378,-2.57291118251023,53.5252040514096));
#20590=CARTESIAN_POINT('Ctrl Pts',(2.11568044063282,-2.44012800840522,53.5368464993517));
#20591=CARTESIAN_POINT('Ctrl Pts',(2.35342340155963,-2.20519511858291,53.5555834994414));
#20592=CARTESIAN_POINT('Ctrl Pts',(2.43650073077047,-2.11304257350967,53.5625624770915));
#20593=CARTESIAN_POINT('Ctrl Pts',(2.55151311848112,-1.96964002528302,53.5731640445865));
#20594=CARTESIAN_POINT('Ctrl Pts',(2.58765620727688,-1.92190941472817,53.5766530157092));
#20595=CARTESIAN_POINT('Ctrl Pts',(2.65228519174817,-1.831430036197,53.5832212274882));
#20596=CARTESIAN_POINT('Ctrl Pts',(2.68111895828496,-1.78895316133468,53.586287033388));
#20597=CARTESIAN_POINT('Ctrl Pts',(2.72811504146043,-1.71603053916185,53.5915322092722));
#20598=CARTESIAN_POINT('Ctrl Pts',(2.74681233450099,-1.68594019340147,53.5936914869712));
#20599=CARTESIAN_POINT('Ctrl Pts',(2.78371044855742,-1.62431492661718,53.5981068330873));
#20600=CARTESIAN_POINT('Ctrl Pts',(2.80188042523399,-1.59276763937255,53.6003636018663));
#20601=CARTESIAN_POINT('Ctrl Pts',(2.8469732920476,-1.51131578268664,53.6061844720179));
#20602=CARTESIAN_POINT('Ctrl Pts',(2.87311972554678,-1.46099785088327,53.6097750314289));
#20603=CARTESIAN_POINT('Ctrl Pts',(2.99296252480382,-1.21469239530267,53.6273342301259));
#20604=CARTESIAN_POINT('Ctrl Pts',(3.06799622582896,-1.0102846682622,53.6419104095151));
#20605=CARTESIAN_POINT('Ctrl Pts',(3.16345648469369,-0.637726260737779,
53.6678897355573));
#20606=CARTESIAN_POINT('Ctrl Pts',(3.19231576705683,-0.472526182697438,
53.6791998258669));
#20607=CARTESIAN_POINT('Ctrl Pts',(3.211391719683,-0.27240994567064,53.6921704878165));
#20608=CARTESIAN_POINT('Ctrl Pts',(3.21405458684576,-0.238950357178618,
53.6943144413036));
#20609=CARTESIAN_POINT('Ctrl Pts',(3.21750898257664,-0.184874900676776,
53.6977330680708));
#20610=CARTESIAN_POINT('Ctrl Pts',(3.21862609495395,-0.16428302464723,53.6990240553682));
#20611=CARTESIAN_POINT('Ctrl Pts',(3.22048894117337,-0.122541122484632,
53.7016172094167));
#20612=CARTESIAN_POINT('Ctrl Pts',(3.22122416340241,-0.101391784046166,
53.7029188014019));
#20613=CARTESIAN_POINT('Ctrl Pts',(3.22265181082952,-0.0440668782097929,
53.7064171579824));
#20614=CARTESIAN_POINT('Ctrl Pts',(3.22294348085417,-0.00788338768629873,
53.7085934214253));
#20615=CARTESIAN_POINT('Ctrl Pts',(3.22091087406947,0.223585255126724,53.7223543320481));
#20616=CARTESIAN_POINT('Ctrl Pts',(3.20144825921741,0.418334366066101,53.7332172868747));
#20617=CARTESIAN_POINT('Ctrl Pts',(3.12782643783467,0.80017099915416,53.7550035225647));
#20618=CARTESIAN_POINT('Ctrl Pts',(3.07414827426386,0.986495907639312,53.765889717617));
#20619=CARTESIAN_POINT('Ctrl Pts',(2.98513654119631,1.21565465098643,53.7803979274953));
#20620=CARTESIAN_POINT('Ctrl Pts',(2.96500323350354,1.26396667973916,53.7835209828908));
#20621=CARTESIAN_POINT('Ctrl Pts',(2.9292128237517,1.34428315128466,53.7888342600876));
#20622=CARTESIAN_POINT('Ctrl Pts',(2.91418489856262,1.37655772798433,53.7910030962683));
#20623=CARTESIAN_POINT('Ctrl Pts',(2.88281461845869,1.44111279615364,53.7954130246769));
#20624=CARTESIAN_POINT('Ctrl Pts',(2.86645719797245,1.47338018828273,53.7976543979769));
#20625=CARTESIAN_POINT('Ctrl Pts',(2.82364600979348,1.55441908852602,53.8033813810989));
#20626=CARTESIAN_POINT('Ctrl Pts',(2.79647041606131,1.60279384209965,53.8068917680219));
#20627=CARTESIAN_POINT('Ctrl Pts',(2.6373161425683,1.86972176983358,53.826793277582));
#20628=CARTESIAN_POINT('Ctrl Pts',(2.48099472928078,2.07266014388038,53.8440672131516));
#20629=CARTESIAN_POINT('Ctrl Pts',(2.23804566940546,2.32071795622034,53.8674794253368));
#20630=CARTESIAN_POINT('Ctrl Pts',(2.17088931717789,2.38365716994643,53.8736517000749));
#20631=CARTESIAN_POINT('Ctrl Pts',(2.07006962176481,2.4703455686221,53.8824066804501));
#20632=CARTESIAN_POINT('Ctrl Pts',(2.0385023949133,2.49645824090771,53.8850801848841));
#20633=CARTESIAN_POINT('Ctrl Pts',(1.98060918254882,2.54251740934866,53.8898505961134));
#20634=CARTESIAN_POINT('Ctrl Pts',(1.95445829114228,2.56267448083339,53.8919584266217));
#20635=CARTESIAN_POINT('Ctrl Pts',(1.91156526781453,2.59469776626446,53.8953342840819));
#20636=CARTESIAN_POINT('Ctrl Pts',(1.89501194066152,2.60681186319998,53.8966179275757));
#20637=CARTESIAN_POINT('Ctrl Pts',(1.86103587841639,2.63118161225266,53.8992119728131));
#20638=CARTESIAN_POINT('Ctrl Pts',(1.84360522345807,2.64342411585323,53.9005215593472));
#20639=CARTESIAN_POINT('Ctrl Pts',(1.79568936228824,2.67637352895882,53.904067756508));
#20640=CARTESIAN_POINT('Ctrl Pts',(1.76496745901041,2.69673240764706,53.9062828977557));
#20641=CARTESIAN_POINT('Ctrl Pts',(1.57812122157672,2.81599092243489,53.9194498454236));
#20642=CARTESIAN_POINT('Ctrl Pts',(1.41405891733148,2.90184835727623,53.9297628923179));
#20643=CARTESIAN_POINT('Ctrl Pts',(1.05418868141317,3.05236355198481,53.9516129824375));
#20644=CARTESIAN_POINT('Ctrl Pts',(0.857740853359154,3.11327907632468,53.9631264156675));
#20645=CARTESIAN_POINT('Ctrl Pts',(0.606685744281197,3.16554496855344,53.9782760337901));
#20646=CARTESIAN_POINT('Ctrl Pts',(0.55628699586078,3.17478926653236,53.9813361596284));
#20647=CARTESIAN_POINT('Ctrl Pts',(0.470722120189921,3.18838391029212,53.9865745964519));
#20648=CARTESIAN_POINT('Ctrl Pts',(0.435664892260104,3.19336299559185,53.9887329422376));
#20649=CARTESIAN_POINT('Ctrl Pts',(0.364387697572853,3.20229077473168,53.9931489327869));
#20650=CARTESIAN_POINT('Ctrl Pts',(0.328168679064477,3.20620488208548,53.9954073207757));
#20651=CARTESIAN_POINT('Ctrl Pts',(0.235299020023553,3.21465102559397,54.0012380436795));
#20652=CARTESIAN_POINT('Ctrl Pts',(0.178582637278034,3.21829993001857,54.0048370150755));
#20653=CARTESIAN_POINT('Ctrl Pts',(-0.0936425913024253,3.22859589635261,
54.0223023276929));
#20654=CARTESIAN_POINT('Ctrl Pts',(-0.309331582753217,3.21510320014451,
54.0367654498928));
#20655=CARTESIAN_POINT('Ctrl Pts',(-0.689552710256647,3.15269038674251,
54.0627930308719));
#20656=CARTESIAN_POINT('Ctrl Pts',(-0.854660547309656,3.11199365571659,
54.0742648134468));
#20657=CARTESIAN_POINT('Ctrl Pts',(-1.04718040851872,3.04805246590306,54.0873464409867));
#20658=CARTESIAN_POINT('Ctrl Pts',(-1.07839609994139,3.03714877656227,54.0894573988245));
#20659=CARTESIAN_POINT('Ctrl Pts',(-1.12870615453252,3.01870188568448,54.0928369552198));
#20660=CARTESIAN_POINT('Ctrl Pts',(-1.14790539329239,3.01145345964324,54.0941212304812));
#20661=CARTESIAN_POINT('Ctrl Pts',(-1.18687701378047,2.99631334225085,54.0967151708548));
#20662=CARTESIAN_POINT('Ctrl Pts',(-1.20664286998425,2.98840822744233,54.0980240420114));
#20663=CARTESIAN_POINT('Ctrl Pts',(-1.26035268240814,2.96630784688494,54.1015659525811));
#20664=CARTESIAN_POINT('Ctrl Pts',(-1.29413517941262,2.95172585452798,54.1037776101112));
#20665=CARTESIAN_POINT('Ctrl Pts',(-1.4976881857728,2.85969678237579,54.1170481407055));
#20666=CARTESIAN_POINT('Ctrl Pts',(-1.66073633103185,2.76819541226212,54.1274549430065));
#20667=CARTESIAN_POINT('Ctrl Pts',(-1.98294952330506,2.54859882815103,54.1492968719715));
#20668=CARTESIAN_POINT('Ctrl Pts',(-2.13971016493408,2.41848595067246,54.1607072025964));
#20669=CARTESIAN_POINT('Ctrl Pts',(-2.31940654664432,2.23810359431552,54.1757474168319));
#20670=CARTESIAN_POINT('Ctrl Pts',(-2.35477126044923,2.20086489911293,54.1788141769598));
#20671=CARTESIAN_POINT('Ctrl Pts',(-2.41300560780607,2.13653378884541,54.1840604840629));
#20672=CARTESIAN_POINT('Ctrl Pts',(-2.43634587097903,2.10987946030708,54.1862199173468));
#20673=CARTESIAN_POINT('Ctrl Pts',(-2.48276663191232,2.05506992520306,54.1906351533523));
#20674=CARTESIAN_POINT('Ctrl Pts',(-2.50581888263873,2.02689765444235,54.1928916492378));
#20675=CARTESIAN_POINT('Ctrl Pts',(-2.56353242359264,1.95387599373125,54.1987108644417));
#20676=CARTESIAN_POINT('Ctrl Pts',(-2.59749553810984,1.90849316816169,54.2023000119246));
#20677=CARTESIAN_POINT('Ctrl Pts',(-2.77851758024688,1.6528162612098,54.2223819454901));
#20678=CARTESIAN_POINT('Ctrl Pts',(-2.90122981653283,1.42645928802078,54.2397617557206));
#20679=CARTESIAN_POINT('Ctrl Pts',(-3.04431400867241,1.06564356688565,54.2659236776472));
#20680=CARTESIAN_POINT('Ctrl Pts',(-3.08529931518377,0.940413963342759,
54.2747264005778));
#20681=CARTESIAN_POINT('Ctrl Pts',(-3.12653883470773,0.782230650267221,
54.2852522329607));
#20682=CARTESIAN_POINT('Ctrl Pts',(-3.13410940925886,0.751324339326221,
54.2872810868837));
#20683=CARTESIAN_POINT('Ctrl Pts',(-3.1457538571183,0.700543696118458,54.2905638374378));
#20684=CARTESIAN_POINT('Ctrl Pts',(-3.15009990823833,0.680734492413324,
54.2918318437902));
#20685=CARTESIAN_POINT('Ctrl Pts',(-3.15869655931377,0.639704535940049,
54.2944305536009));
#20686=CARTESIAN_POINT('Ctrl Pts',(-3.16292092423086,0.618479696918545,
54.2957598742098));
#20687=CARTESIAN_POINT('Ctrl Pts',(-3.17406895501523,0.559363377753016,
54.2994247886798));
#20688=CARTESIAN_POINT('Ctrl Pts',(-3.18052782925342,0.521386744293538,
54.3017364322697));
#20689=CARTESIAN_POINT('Ctrl Pts',(-3.21042212497873,0.324300025070463,
54.3135549037948));
#20690=CARTESIAN_POINT('Ctrl Pts',(-3.22260666222988,0.163699347225663,
54.3225942964115));
#20691=CARTESIAN_POINT('Ctrl Pts',(-3.22293798841606,-0.211402741709704,
54.3436183764822));
#20692=CARTESIAN_POINT('Ctrl Pts',(-3.20176299569259,-0.425117169876697,
54.3555594647547));
#20693=CARTESIAN_POINT('Ctrl Pts',(-3.14832387025797,-0.690952181915791,
54.3714961551642));
#20694=CARTESIAN_POINT('Ctrl Pts',(-3.13562869594029,-0.746451748433032,
54.3748817305995));
#20695=CARTESIAN_POINT('Ctrl Pts',(-3.11240559364864,-0.836885527360803,
54.3805105752936));
#20696=CARTESIAN_POINT('Ctrl Pts',(-3.10274228150948,-0.872029892382777,
54.3827262287743));
#20697=CARTESIAN_POINT('Ctrl Pts',(-3.0825239340578,-0.940965749010611,
54.3871316574012));
#20698=CARTESIAN_POINT('Ctrl Pts',(-3.07200403807014,-0.974762215777557,
54.3893200277684));
#20699=CARTESIAN_POINT('Ctrl Pts',(-3.04492280461057,-1.05696729886844,
54.3947160279171));
#20700=CARTESIAN_POINT('Ctrl Pts',(-3.02776170535773,-1.105166655917,54.3979427568696));
#20701=CARTESIAN_POINT('Ctrl Pts',(-2.93416920249864,-1.34946751933685,
54.4146306820711));
#20702=CARTESIAN_POINT('Ctrl Pts',(-2.83981774490436,-1.53812259221357,
54.428677858855));
#20703=CARTESIAN_POINT('Ctrl Pts',(-2.63264493851938,-1.86740695018094,
54.4549445615683));
#20704=CARTESIAN_POINT('Ctrl Pts',(-2.5251035904157,-2.01044489994952,54.4670611577171));
#20705=CARTESIAN_POINT('Ctrl Pts',(-2.38132006077559,-2.17182812616933,
54.4810660671223));
#20706=CARTESIAN_POINT('Ctrl Pts',(-2.3558970178997,-2.19937994876969,54.483469260114));
#20707=CARTESIAN_POINT('Ctrl Pts',(-2.31519314411685,-2.24197624436961,
54.4871956178509));
#20708=CARTESIAN_POINT('Ctrl Pts',(-2.3002337928999,-2.25732171682827,54.4885403541956));
#20709=CARTESIAN_POINT('Ctrl Pts',(-2.27072485665521,-2.2869943264476,54.4911430596378));
#20710=CARTESIAN_POINT('Ctrl Pts',(-2.25619025225862,-2.30133439509154,
54.4924018961524));
#20711=CARTESIAN_POINT('Ctrl Pts',(-2.21814473060734,-2.33816380012209,
54.4956406538933));
#20712=CARTESIAN_POINT('Ctrl Pts',(-2.1944270660587,-2.3604376792357,54.4976050818879));
#20713=CARTESIAN_POINT('Ctrl Pts',(-2.05529216987988,-2.48719276659433,
54.5088459730212));
#20714=CARTESIAN_POINT('Ctrl Pts',(-1.93275011846136,-2.58357144419009,
54.5176476741744));
#20715=CARTESIAN_POINT('Ctrl Pts',(-1.60915677813517,-2.80211466050229,
54.539565990347));
#20716=CARTESIAN_POINT('Ctrl Pts',(-1.40084925226597,-2.91184542007592,
54.5525842560118));
#20717=CARTESIAN_POINT('Ctrl Pts',(-1.13145026759469,-3.01810316397767,
54.5696355672569));
#20718=CARTESIAN_POINT('Ctrl Pts',(-1.07991989271876,-3.03692260685171,
54.5729027109954));
#20719=CARTESIAN_POINT('Ctrl Pts',(-0.993761133587291,-3.06591855891881,
54.5783886583007));
#20720=CARTESIAN_POINT('Ctrl Pts',(-0.959396265448393,-3.07684520973072,
54.5805827198383));
#20721=CARTESIAN_POINT('Ctrl Pts',(-0.890658133322215,-3.09743767161327,
54.5849866811192));
#20722=CARTESIAN_POINT('Ctrl Pts',(-0.856293208923901,-3.10711342220679,
54.587195895483));
#20723=CARTESIAN_POINT('Ctrl Pts',(-0.770634449312444,-3.12970244903156,
54.5927241086433));
#20724=CARTESIAN_POINT('Ctrl Pts',(-0.71917152955154,-3.14192722081825,
54.5960644315389));
#20725=CARTESIAN_POINT('Ctrl Pts',(-0.60879151596347,-3.16529357745695,
54.603273063545));
#20726=CARTESIAN_POINT('Ctrl Pts',(-0.549818244493652,-3.17606826451108,
54.6071509777578));
#20727=CARTESIAN_POINT('Ctrl Pts',(-0.490582094190866,-3.18519179506656,
54.6110712720502));
#20728=CARTESIAN_POINT('Ctrl Pts',(-0.490582094360392,-3.18519179504045,
54.8568649631546));
#20729=CARTESIAN_POINT('Ctrl Pts',(-0.510063376476227,-3.1821912949776,
54.85567814763));
#20730=CARTESIAN_POINT('Ctrl Pts',(-0.529517570778685,-3.1790119999361,
54.8544997008938));
#20731=CARTESIAN_POINT('Ctrl Pts',(-0.732390573842784,-3.14394346117165,
54.8422694795125));
#20732=CARTESIAN_POINT('Ctrl Pts',(-0.91276722127825,-3.0963927018116,54.831885054248));
#20733=CARTESIAN_POINT('Ctrl Pts',(-1.27892570161431,-2.96506151521871,
54.8100952785896));
#20734=CARTESIAN_POINT('Ctrl Pts',(-1.46289964096266,-2.87874184484615,
54.7987148588697));
#20735=CARTESIAN_POINT('Ctrl Pts',(-1.6821143513557,-2.74941589060746,54.7836861278856));
#20736=CARTESIAN_POINT('Ctrl Pts',(-1.72605068049512,-2.72204794868504,
54.7805960452093));
#20737=CARTESIAN_POINT('Ctrl Pts',(-1.79897870458099,-2.67414536361438,
54.775321967063));
#20738=CARTESIAN_POINT('Ctrl Pts',(-1.82832517116497,-2.65416742478404,
54.7731586085741));
#20739=CARTESIAN_POINT('Ctrl Pts',(-1.88352010341653,-2.6152430594055,54.769007688171));
#20740=CARTESIAN_POINT('Ctrl Pts',(-1.90942780558863,-2.59638779419708,
54.7670237600481));
#20741=CARTESIAN_POINT('Ctrl Pts',(-1.97686681233774,-2.54575131155642,
54.7617627103987));
#20742=CARTESIAN_POINT('Ctrl Pts',(-2.01791178265878,-2.51334113572709,
54.7584615388973));
#20743=CARTESIAN_POINT('Ctrl Pts',(-2.25332199710811,-2.31797047025283,
54.7389265420836));
#20744=CARTESIAN_POINT('Ctrl Pts',(-2.42866330342796,-2.13354162877199,
54.7218075171242));
#20745=CARTESIAN_POINT('Ctrl Pts',(-2.66617821405875,-1.81605233913119,
54.6950515112968));
#20746=CARTESIAN_POINT('Ctrl Pts',(-2.74410674070794,-1.69600646253892,
54.6854609395288));
#20747=CARTESIAN_POINT('Ctrl Pts',(-2.82951995409275,-1.54304005343017,
54.6741744675714));
#20748=CARTESIAN_POINT('Ctrl Pts',(-2.84480658860076,-1.51467205482868,
54.6721189459444));
#20749=CARTESIAN_POINT('Ctrl Pts',(-2.86905272395822,-1.46801513033065,
54.6688047921172));
#20750=CARTESIAN_POINT('Ctrl Pts',(-2.8782686717668,-1.44986257560209,54.6675315444779));
#20751=CARTESIAN_POINT('Ctrl Pts',(-2.89687209409043,-1.41234299582191,
54.664934744533));
#20752=CARTESIAN_POINT('Ctrl Pts',(-2.90623869747397,-1.39296710697062,
54.6636123773449));
#20753=CARTESIAN_POINT('Ctrl Pts',(-2.93157397840242,-1.33919000632293,
54.6599895853819));
#20754=CARTESIAN_POINT('Ctrl Pts',(-2.94713107045096,-1.30459748420348,
54.6577122165));
#20755=CARTESIAN_POINT('Ctrl Pts',(-3.0281355679944,-1.11562810595729,54.6455145409248));
#20756=CARTESIAN_POINT('Ctrl Pts',(-3.08207612340782,-0.956582217573359,
54.6361086581793));
#20757=CARTESIAN_POINT('Ctrl Pts',(-3.15960361010104,-0.651626454712516,
54.6184780420143));
#20758=CARTESIAN_POINT('Ctrl Pts',(-3.18602595702939,-0.506900414735007,
54.610271236269));
#20759=CARTESIAN_POINT('Ctrl Pts',(-3.20981994783154,-0.295752167679915,
54.5980734732127));
#20760=CARTESIAN_POINT('Ctrl Pts',(-3.21517049408673,-0.230415739795087,
54.5942700264858));
#20761=CARTESIAN_POINT('Ctrl Pts',(-3.2213343581676,-0.110156007277225,
54.5871800762855));
#20762=CARTESIAN_POINT('Ctrl Pts',(-3.22274295511204,-0.0552875741277878,
54.5839113801572));
#20763=CARTESIAN_POINT('Ctrl Pts',(-3.22275458631807,0.0356527003089716,
54.5784235007172));
#20764=CARTESIAN_POINT('Ctrl Pts',(-3.22215381187848,0.0717139417525594,
54.5762290953662));
#20765=CARTESIAN_POINT('Ctrl Pts',(-3.21975443429646,0.1434337548322,54.5718249619178));
#20766=CARTESIAN_POINT('Ctrl Pts',(-3.21796819882228,0.179087600705352,
54.5696159281677));
#20767=CARTESIAN_POINT('Ctrl Pts',(-3.21206791962979,0.267455490430315,
54.5640891827152));
#20768=CARTESIAN_POINT('Ctrl Pts',(-3.20724829203575,0.320110339395274,
54.5607501740726));
#20769=CARTESIAN_POINT('Ctrl Pts',(-3.19393262683197,0.434503559790764,
54.5533922080871));
#20770=CARTESIAN_POINT('Ctrl Pts',(-3.18493674747177,0.496161356330239,
54.5493597186413));
#20771=CARTESIAN_POINT('Ctrl Pts',(-3.15108149125626,0.688912539071098,
54.53654854483));
#20772=CARTESIAN_POINT('Ctrl Pts',(-3.11986814139888,0.818738439484068,
54.5276126017586));
#20773=CARTESIAN_POINT('Ctrl Pts',(-3.0245579085852,1.12904070008866,54.5057113017588));
#20774=CARTESIAN_POINT('Ctrl Pts',(-2.9522513469773,1.30648567058488,54.4927090700293));
#20775=CARTESIAN_POINT('Ctrl Pts',(-2.84789278301625,1.50895970258258,54.4779639939658));
#20776=CARTESIAN_POINT('Ctrl Pts',(-2.83060054181081,1.54115330783923,54.4756233212579));
#20777=CARTESIAN_POINT('Ctrl Pts',(-2.80239847153739,1.59158138895333,54.4719710151409));
#20778=CARTESIAN_POINT('Ctrl Pts',(-2.79184997181253,1.61001313807327,54.4706391266519));
#20779=CARTESIAN_POINT('Ctrl Pts',(-2.77073021605332,1.64608458134759,54.46804065288));
#20780=CARTESIAN_POINT('Ctrl Pts',(-2.76017092227311,1.66372981424799,54.4667735174723));
#20781=CARTESIAN_POINT('Ctrl Pts',(-2.7320883159667,1.70965425619625,54.4634828455621));
#20782=CARTESIAN_POINT('Ctrl Pts',(-2.7142942225495,1.73776618408051,54.4614757778645));
#20783=CARTESIAN_POINT('Ctrl Pts',(-2.60387768252931,1.90637211244367,54.4494506484581));
#20784=CARTESIAN_POINT('Ctrl Pts',(-2.50079314727974,2.03972547339855,54.4399849269798));
#20785=CARTESIAN_POINT('Ctrl Pts',(-2.24209595866702,2.32511494871561,54.4183922014856));
#20786=CARTESIAN_POINT('Ctrl Pts',(-2.08060457362502,2.47067376573019,54.406312723231));
#20787=CARTESIAN_POINT('Ctrl Pts',(-1.85998047245909,2.63245286301889,54.3902305071777));
#20788=CARTESIAN_POINT('Ctrl Pts',(-1.81335947187898,2.66478184606136,54.3868563247024));
#20789=CARTESIAN_POINT('Ctrl Pts',(-1.73545376162695,2.71581360477255,54.3812411922853));
#20790=CARTESIAN_POINT('Ctrl Pts',(-1.70466101112749,2.73524660051163,54.3790275759583));
#20791=CARTESIAN_POINT('Ctrl Pts',(-1.64327411118485,2.77254802506471,54.3746223128247));
#20792=CARTESIAN_POINT('Ctrl Pts',(-1.61270144054324,2.79044194733269,54.372432003279));
#20793=CARTESIAN_POINT('Ctrl Pts',(-1.53713120143195,2.83301581951627,54.367023890353));
#20794=CARTESIAN_POINT('Ctrl Pts',(-1.49182838723517,2.85713117437827,54.3637867882773));
#20795=CARTESIAN_POINT('Ctrl Pts',(-1.39249728128651,2.90700001102965,54.3566958924982));
#20796=CARTESIAN_POINT('Ctrl Pts',(-1.33828899831606,2.93235052330283,54.3528302732313));
#20797=CARTESIAN_POINT('Ctrl Pts',(-1.16978381634417,3.00550620152427,54.3408297034384));
#20798=CARTESIAN_POINT('Ctrl Pts',(-1.05341778478968,3.04824018565404,54.3325592847735));
#20799=CARTESIAN_POINT('Ctrl Pts',(-0.733490013640261,3.14521843162858,
54.3100382282056));
#20800=CARTESIAN_POINT('Ctrl Pts',(-0.526584642731852,3.18639690430633,
54.295677508164));
#20801=CARTESIAN_POINT('Ctrl Pts',(-0.282808764264148,3.21050251867335,
54.2798550563176));
#20802=CARTESIAN_POINT('Ctrl Pts',(-0.248430864767838,3.2133455378287,54.2776497292495));
#20803=CARTESIAN_POINT('Ctrl Pts',(-0.193246948454593,3.21701823022155,
54.2741582163811));
#20804=CARTESIAN_POINT('Ctrl Pts',(-0.172467866053886,3.21819911937743,
54.2728545185015));
#20805=CARTESIAN_POINT('Ctrl Pts',(-0.130752558560434,3.22016462015822,
54.2702612849897));
#20806=CARTESIAN_POINT('Ctrl Pts',(-0.109817238493129,3.220946544569,54.2689719399885));
#20807=CARTESIAN_POINT('Ctrl Pts',(-0.0537350537837422,3.22249373470219,
54.2655468686595));
#20808=CARTESIAN_POINT('Ctrl Pts',(-0.0185798613695318,3.222888198736,54.2634301934472));
#20809=CARTESIAN_POINT('Ctrl Pts',(0.176678525717378,3.22188386711047,54.251807808747));
#20810=CARTESIAN_POINT('Ctrl Pts',(0.336514746736353,3.20913067856127,54.2427872893362));
#20811=CARTESIAN_POINT('Ctrl Pts',(0.714580976968956,3.1503938644972,54.2213319423596));
#20812=CARTESIAN_POINT('Ctrl Pts',(0.93025994907462,3.09357628651168,54.2089587673856));
#20813=CARTESIAN_POINT('Ctrl Pts',(1.190965635434,2.99514273180092,54.1925705505967));
#20814=CARTESIAN_POINT('Ctrl Pts',(1.24303754449917,2.97390925094386,54.1892248412624));
#20815=CARTESIAN_POINT('Ctrl Pts',(1.32778326022004,2.9367376590655,54.1836441112269));
#20816=CARTESIAN_POINT('Ctrl Pts',(1.36079125085731,2.92158920297177,54.1814357259609));
#20817=CARTESIAN_POINT('Ctrl Pts',(1.42553752027605,2.89053974481266,54.1770311466058));
#20818=CARTESIAN_POINT('Ctrl Pts',(1.4572830684078,2.87466574363278,54.1748361207666));
#20819=CARTESIAN_POINT('Ctrl Pts',(1.53462280660184,2.83438257077156,54.1693978451491));
#20820=CARTESIAN_POINT('Ctrl Pts',(1.57990272702172,2.80939470326312,54.1661347926162));
#20821=CARTESIAN_POINT('Ctrl Pts',(1.79681482676243,2.68278852473457,54.1501055281509));
#20822=CARTESIAN_POINT('Ctrl Pts',(1.95933933349941,2.56648888628889,54.1368217239276));
#20823=CARTESIAN_POINT('Ctrl Pts',(2.25363033317695,2.3115687177846,54.1105503290812));
#20824=CARTESIAN_POINT('Ctrl Pts',(2.38593947859964,2.17474176621434,54.0976376248897));
#20825=CARTESIAN_POINT('Ctrl Pts',(2.52846936786938,1.99857493131814,54.0829677141026));
#20826=CARTESIAN_POINT('Ctrl Pts',(2.5510211094432,1.96970826753548,54.080621244722));
#20827=CARTESIAN_POINT('Ctrl Pts',(2.58587396159763,1.92349295118756,54.0769620639383));
#20828=CARTESIAN_POINT('Ctrl Pts',(2.59850329941778,1.90639710987125,54.0756289767073));
#20829=CARTESIAN_POINT('Ctrl Pts',(2.62300842312808,1.87252946796888,54.0730301452369));
#20830=CARTESIAN_POINT('Ctrl Pts',(2.63489460036788,1.8557667623581,54.0717638209651));
#20831=CARTESIAN_POINT('Ctrl Pts',(2.66556131925622,1.81162975712169,54.06847818322));
#20832=CARTESIAN_POINT('Ctrl Pts',(2.68408123997484,1.78407612360554,54.0664752433602));
#20833=CARTESIAN_POINT('Ctrl Pts',(2.72465926842631,1.7216422616976,54.0620320504714));
#20834=CARTESIAN_POINT('Ctrl Pts',(2.74648006607318,1.68661428479832,54.0596041790711));
#20835=CARTESIAN_POINT('Ctrl Pts',(2.81534292059383,1.57118958959713,54.0517806066921));
#20836=CARTESIAN_POINT('Ctrl Pts',(2.85957570286652,1.48916796449042,54.0464936342767));
#20837=CARTESIAN_POINT('Ctrl Pts',(3.0150776071079,1.16825951496468,54.0264157559186));
#20838=CARTESIAN_POINT('Ctrl Pts',(3.10044766980587,0.918008038861733,54.0119069145922));
#20839=CARTESIAN_POINT('Ctrl Pts',(3.16482492677151,0.610397900768834,53.9933333454291));
#20840=CARTESIAN_POINT('Ctrl Pts',(3.17405999750145,0.560397291396893,53.9902957253355));
#20841=CARTESIAN_POINT('Ctrl Pts',(3.1876475546923,0.475652127818242,53.9851051169721));
#20842=CARTESIAN_POINT('Ctrl Pts',(3.19262373802499,0.441016324498363,53.982971934843));
#20843=CARTESIAN_POINT('Ctrl Pts',(3.20162986433332,0.370151504111411,53.9785803447379));
#20844=CARTESIAN_POINT('Ctrl Pts',(3.20561104523082,0.333921515288071,53.9763207450685));
#20845=CARTESIAN_POINT('Ctrl Pts',(3.2142333548562,0.240958714274003,53.9704829742739));
#20846=CARTESIAN_POINT('Ctrl Pts',(3.21798729779291,0.184158253721435,53.9668780410474));
#20847=CARTESIAN_POINT('Ctrl Pts',(3.22678929045453,-0.0385166270848243,
53.9525897409715));
#20848=CARTESIAN_POINT('Ctrl Pts',(3.22052704324914,-0.204561837013675,
53.9415797016312));
#20849=CARTESIAN_POINT('Ctrl Pts',(3.17802142478831,-0.572981673708231,
53.9166144875728));
#20850=CARTESIAN_POINT('Ctrl Pts',(3.13515840014403,-0.773897507745744,
53.9026232342128));
#20851=CARTESIAN_POINT('Ctrl Pts',(3.06118143319533,-1.0084458949903,53.8866352535821));
#20852=CARTESIAN_POINT('Ctrl Pts',(3.04811822815049,-1.04726811696155,53.8840020891666));
#20853=CARTESIAN_POINT('Ctrl Pts',(3.02686170489738,-1.1066686551059,53.8800045119826));
#20854=CARTESIAN_POINT('Ctrl Pts',(3.01919088395622,-1.12742794218081,53.8786134254569));
#20855=CARTESIAN_POINT('Ctrl Pts',(3.00417328280183,-1.16681677203176,53.875987631624));
#20856=CARTESIAN_POINT('Ctrl Pts',(2.99686578374266,-1.18545939741121,53.8747509878917));
#20857=CARTESIAN_POINT('Ctrl Pts',(2.97802938070205,-1.232226598959,53.8716617481628));
#20858=CARTESIAN_POINT('Ctrl Pts',(2.96627514318384,-1.26025922380229,53.869821878414));
#20859=CARTESIAN_POINT('Ctrl Pts',(2.91177562314392,-1.38524611512165,53.8616540342483));
#20860=CARTESIAN_POINT('Ctrl Pts',(2.86465758822717,-1.48023143880938,53.8555423653064));
#20861=CARTESIAN_POINT('Ctrl Pts',(2.73985303670194,-1.70345333290227,53.8410199769803));
#20862=CARTESIAN_POINT('Ctrl Pts',(2.65774039708992,-1.82892479893098,53.8327152062218));
#20863=CARTESIAN_POINT('Ctrl Pts',(2.47627652318094,-2.06804080338671,53.8158098874259));
#20864=CARTESIAN_POINT('Ctrl Pts',(2.37708883478255,-2.18132532006941,53.8072274375089));
#20865=CARTESIAN_POINT('Ctrl Pts',(2.23515041867828,-2.32221477967414,53.7953934931294));
#20866=CARTESIAN_POINT('Ctrl Pts',(2.19913899695723,-2.35634593270274,53.7924263078995));
#20867=CARTESIAN_POINT('Ctrl Pts',(2.13656047167297,-2.41297267527477,53.7873185264838));
#20868=CARTESIAN_POINT('Ctrl Pts',(2.11039000659383,-2.43589442598669,53.785196182592));
#20869=CARTESIAN_POINT('Ctrl Pts',(2.05579745515643,-2.48216985387171,53.7807936536765));
#20870=CARTESIAN_POINT('Ctrl Pts',(2.02733641945124,-2.50546946201431,53.7785117220236));
#20871=CARTESIAN_POINT('Ctrl Pts',(1.95245301836596,-2.56466128010022,53.7725385313103));
#20872=CARTESIAN_POINT('Ctrl Pts',(1.9054397749277,-2.59978053377707,53.7688180155848));
#20873=CARTESIAN_POINT('Ctrl Pts',(1.7988001282533,-2.67499435617886,53.7604390202086));
#20874=CARTESIAN_POINT('Ctrl Pts',(1.73873974725404,-2.71441699719679,53.7557594517152));
#20875=CARTESIAN_POINT('Ctrl Pts',(1.525752251308,-2.84424795313825,53.7393137406151));
#20876=CARTESIAN_POINT('Ctrl Pts',(1.36671391899218,-2.9239956993436,53.7272704164231));
#20877=CARTESIAN_POINT('Ctrl Pts',(1.0774644457586,-3.04026035364349,53.7062516519805));
#20878=CARTESIAN_POINT('Ctrl Pts',(0.949983053072209,-3.08247487547531,
53.6972733566348));
#20879=CARTESIAN_POINT('Ctrl Pts',(0.789234370850497,-3.12478063720933,
53.6865672561343));
#20880=CARTESIAN_POINT('Ctrl Pts',(0.758116053302502,-3.13247588227786,
53.6845228700491));
#20881=CARTESIAN_POINT('Ctrl Pts',(0.709037547476687,-3.14383825763317,
53.681348053055));
#20882=CARTESIAN_POINT('Ctrl Pts',(0.691152879655012,-3.14781844613387,
53.6802013761708));
#20883=CARTESIAN_POINT('Ctrl Pts',(0.652802752370202,-3.15601055827438,
53.677765888194));
#20884=CARTESIAN_POINT('Ctrl Pts',(0.632328161527379,-3.16017645544471,
53.6764797611073));
#20885=CARTESIAN_POINT('Ctrl Pts',(0.577563562966301,-3.17076565425228,
53.673073883215));
#20886=CARTESIAN_POINT('Ctrl Pts',(0.543206429755999,-3.17683199116043,
53.6709728108066));
#20887=CARTESIAN_POINT('Ctrl Pts',(0.465206083339248,-3.18930179407254,
53.6662695297599));
#20888=CARTESIAN_POINT('Ctrl Pts',(0.421515837015358,-3.1953696779379,53.6636820495336));
#20889=CARTESIAN_POINT('Ctrl Pts',(0.273960462157292,-3.21278348609836,
53.6550605280975));
#20890=CARTESIAN_POINT('Ctrl Pts',(0.169667920374966,-3.2199762880829,53.6491601595463));
#20891=CARTESIAN_POINT('Ctrl Pts',(-0.120882067791962,-3.225856123177,53.6328426080335));
#20892=CARTESIAN_POINT('Ctrl Pts',(-0.306834800524082,-3.21349248787365,
53.6225167194536));
#20893=CARTESIAN_POINT('Ctrl Pts',(-0.490582106922524,-3.18519179310563,
53.611790309282));
#20894=CARTESIAN_POINT('Origin',(-9.35406549764863E-15,0.,41.4527091182931));
#20895=CARTESIAN_POINT('',(-0.49058209429419,-3.18519179505064,52.1162187418821));
#20896=CARTESIAN_POINT('',(-0.490582094296231,-3.18519179505033,52.3599056026743));
#20897=CARTESIAN_POINT('',(-0.490582094296226,-3.18519179505033,41.4527091182931));
#20898=CARTESIAN_POINT('',(-3.2227494359304,-0.00190675388112439,53.0831681868229));
#20899=CARTESIAN_POINT('Ctrl Pts',(-0.49058209429419,-3.18519179505064,
52.1162187418821));
#20900=CARTESIAN_POINT('Ctrl Pts',(-0.471422613079779,-3.18814273145403,
52.1174424045019));
#20901=CARTESIAN_POINT('Ctrl Pts',(-0.452236283182814,-3.19092083075083,
52.1186572587537));
#20902=CARTESIAN_POINT('Ctrl Pts',(-0.412634041374947,-3.19629068845668,
52.1211415364045));
#20903=CARTESIAN_POINT('Ctrl Pts',(-0.392216192911372,-3.19886034581764,
52.1224095510059));
#20904=CARTESIAN_POINT('Ctrl Pts',(-0.338644886686095,-3.20508183815937,
52.1257061957732));
#20905=CARTESIAN_POINT('Ctrl Pts',(-0.305455898587567,-3.20841500418907,
52.1277182390375));
#20906=CARTESIAN_POINT('Ctrl Pts',(-0.13201741738564,-3.22311757488889,
52.1381023948326));
#20907=CARTESIAN_POINT('Ctrl Pts',(0.00882799816034327,-3.22580931540793,
52.1460950759228));
#20908=CARTESIAN_POINT('Ctrl Pts',(0.402765974297692,-3.20752618248547,
52.1682731323922));
#20909=CARTESIAN_POINT('Ctrl Pts',(0.653824315681166,-3.16590415144211,
52.1822739342074));
#20910=CARTESIAN_POINT('Ctrl Pts',(0.947622086190241,-3.0807245706664,52.2003271277172));
#20911=CARTESIAN_POINT('Ctrl Pts',(0.997477051463299,-3.06494544381852,
52.2034474847888));
#20912=CARTESIAN_POINT('Ctrl Pts',(1.077224405187,-3.03755354990032,52.2085427635738));
#20913=CARTESIAN_POINT('Ctrl Pts',(1.10736691258954,-3.02669496231513,52.2104930201567));
#20914=CARTESIAN_POINT('Ctrl Pts',(1.17055289575816,-3.00286253064938,52.2146354414854));
#20915=CARTESIAN_POINT('Ctrl Pts',(1.20355375699964,-2.98978856354878,52.2168307065457));
#20916=CARTESIAN_POINT('Ctrl Pts',(1.2841205626578,-2.95632033169812,52.222271591795));
#20917=CARTESIAN_POINT('Ctrl Pts',(1.33142273408795,-2.935320857193,52.2255370668947));
#20918=CARTESIAN_POINT('Ctrl Pts',(1.56582986623484,-2.82442563199419,52.2420876233332));
#20919=CARTESIAN_POINT('Ctrl Pts',(1.74442046309859,-2.71775202842572,52.2559387553089));
#20920=CARTESIAN_POINT('Ctrl Pts',(2.05706302484094,-2.48742871141326,52.2821553253392));
#20921=CARTESIAN_POINT('Ctrl Pts',(2.19336162851785,-2.36811815089191,52.2944240922266));
#20922=CARTESIAN_POINT('Ctrl Pts',(2.34474162724589,-2.21126315177056,52.3085439493399));
#20923=CARTESIAN_POINT('Ctrl Pts',(2.37008017867017,-2.18408292919107,52.3109253266136));
#20924=CARTESIAN_POINT('Ctrl Pts',(2.40923730992446,-2.14059557481503,52.3146257739316));
#20925=CARTESIAN_POINT('Ctrl Pts',(2.42337272024541,-2.1245796170276,52.3159659556855));
#20926=CARTESIAN_POINT('Ctrl Pts',(2.45073704128388,-2.09294632683357,52.3185669320059));
#20927=CARTESIAN_POINT('Ctrl Pts',(2.46397827663471,-2.07734143938101,52.3198284849702));
#20928=CARTESIAN_POINT('Ctrl Pts',(2.49803778177659,-2.03641821003639,52.3230844289045));
#20929=CARTESIAN_POINT('Ctrl Pts',(2.51862068831802,-2.01090574148968,52.3250630046848));
#20930=CARTESIAN_POINT('Ctrl Pts',(2.6501908580659,-1.84263471737163,52.3378158705556));
#20931=CARTESIAN_POINT('Ctrl Pts',(2.74939748059288,-1.69104813762514,52.3479452698348));
#20932=CARTESIAN_POINT('Ctrl Pts',(2.93224542058372,-1.35262257976696,52.3694955054425));
#20933=CARTESIAN_POINT('Ctrl Pts',(3.01188534193679,-1.16455477356078,52.3808856889092));
#20934=CARTESIAN_POINT('Ctrl Pts',(3.09053479669109,-0.915431611605484,
52.3962329416021));
#20935=CARTESIAN_POINT('Ctrl Pts',(3.10636674075913,-0.860177565033137,
52.3996495968494));
#20936=CARTESIAN_POINT('Ctrl Pts',(3.12983707905995,-0.769138102149606,
52.405316108137));
#20937=CARTESIAN_POINT('Ctrl Pts',(3.13835870373939,-0.733592557472927,
52.4075375783617));
#20938=CARTESIAN_POINT('Ctrl Pts',(3.15392395705122,-0.663422353162895,
52.4119443270527));
#20939=CARTESIAN_POINT('Ctrl Pts',(3.16100639590858,-0.628811540833945,
52.4141280218646));
#20940=CARTESIAN_POINT('Ctrl Pts',(3.17687476915188,-0.544206240445368,
52.4194934457681));
#20941=CARTESIAN_POINT('Ctrl Pts',(3.18505103432578,-0.49410846541297,52.4226937637584));
#20942=CARTESIAN_POINT('Ctrl Pts',(3.21781154853035,-0.258499391474556,
52.4378614871394));
#20943=CARTESIAN_POINT('Ctrl Pts',(3.22738777920457,-0.0712925020199418,
52.4502801860719));
#20944=CARTESIAN_POINT('Ctrl Pts',(3.21321698339483,0.323302485876479,52.47688623264));
#20945=CARTESIAN_POINT('Ctrl Pts',(3.18569725825432,0.529746007867061,52.4910573598766));
#20946=CARTESIAN_POINT('Ctrl Pts',(3.13058648240641,0.766000504741335,52.5067321295767));
#20947=CARTESIAN_POINT('Ctrl Pts',(3.12213257273492,0.799760539931585,52.5089577330203));
#20948=CARTESIAN_POINT('Ctrl Pts',(3.10773492918348,0.853543759116961,52.5124733704233));
#20949=CARTESIAN_POINT('Ctrl Pts',(3.10214076886668,0.873656709152015,52.5137813150147));
#20950=CARTESIAN_POINT('Ctrl Pts',(3.09056019092132,0.913778624694611,52.51637488935));
#20951=CARTESIAN_POINT('Ctrl Pts',(3.08457392492454,0.933786606366464,52.5176604499905));
#20952=CARTESIAN_POINT('Ctrl Pts',(3.06808307899381,0.987014471805906,52.521063070057));
#20953=CARTESIAN_POINT('Ctrl Pts',(3.05723332281614,1.02012547178175,52.5231615135305));
#20954=CARTESIAN_POINT('Ctrl Pts',(3.03146237010262,1.09466514434225,52.5278578000113));
#20955=CARTESIAN_POINT('Ctrl Pts',(3.01622467845812,1.13597751431622,52.5304409803315));
#20956=CARTESIAN_POINT('Ctrl Pts',(2.96210634630069,1.27392776981211,52.5390403781021));
#20957=CARTESIAN_POINT('Ctrl Pts',(2.91938771394712,1.36899370582799,52.544923645375));
#20958=CARTESIAN_POINT('Ctrl Pts',(2.76378258770588,1.6747199972565,52.5641867635012));
#20959=CARTESIAN_POINT('Ctrl Pts',(2.632104793227,1.87488557525754,52.5774201669147));
#20960=CARTESIAN_POINT('Ctrl Pts',(2.44481861772149,2.10045974902195,52.5946910408471));
#20961=CARTESIAN_POINT('Ctrl Pts',(2.40906382022346,2.14137344544636,52.5979282411802));
#20962=CARTESIAN_POINT('Ctrl Pts',(2.34795212277716,2.20783415511511,52.6033781806802));
#20963=CARTESIAN_POINT('Ctrl Pts',(2.32317016978486,2.23389593065752,52.6055668877421));
#20964=CARTESIAN_POINT('Ctrl Pts',(2.2728662028248,2.28505526857974,52.6099713048634));
#20965=CARTESIAN_POINT('Ctrl Pts',(2.24735188199573,2.31015317928954,52.6121865212443));
#20966=CARTESIAN_POINT('Ctrl Pts',(2.18275376129814,2.37161398172644,52.617752212039));
#20967=CARTESIAN_POINT('Ctrl Pts',(2.14317564630202,2.40743940139083,52.6211246512535));
#20968=CARTESIAN_POINT('Ctrl Pts',(1.96265710835377,2.5628613358724,52.6363508871203));
#20969=CARTESIAN_POINT('Ctrl Pts',(1.81249063149865,2.67116852599916,52.6486355464533));
#20970=CARTESIAN_POINT('Ctrl Pts',(1.47933785067283,2.87037288540808,52.6748013366586));
#20971=CARTESIAN_POINT('Ctrl Pts',(1.29528497271156,2.95799385834272,52.6886617018734));
#20972=CARTESIAN_POINT('Ctrl Pts',(1.07102348504934,3.03978169568756,52.7040938779604));
#20973=CARTESIAN_POINT('Ctrl Pts',(1.03765650706262,3.05133303185523,52.7063530076903));
#20974=CARTESIAN_POINT('Ctrl Pts',(0.98416949440476,3.0688708211572,52.7099084523376));
#20975=CARTESIAN_POINT('Ctrl Pts',(0.964170067072682,3.0752128136938,52.7112233520003));
#20976=CARTESIAN_POINT('Ctrl Pts',(0.924241120709941,3.08744679691797,52.7138177524495));
#20977=CARTESIAN_POINT('Ctrl Pts',(0.904313770302774,3.0933422098082,52.715097370741));
#20978=CARTESIAN_POINT('Ctrl Pts',(0.851306376083945,3.10846817490518,52.7184644764938));
#20979=CARTESIAN_POINT('Ctrl Pts',(0.818132509615256,3.11736368583707,52.7205340342382));
#20980=CARTESIAN_POINT('Ctrl Pts',(0.742937299594117,3.1362440271104,52.7251534290824));
#20981=CARTESIAN_POINT('Ctrl Pts',(0.700844261146414,3.1459180025066,52.7276893167787));
#20982=CARTESIAN_POINT('Ctrl Pts',(0.559986181482525,3.17532279752959,52.7360472467679));
#20983=CARTESIAN_POINT('Ctrl Pts',(0.460488449175386,3.19127122764661,52.7417441007411));
#20984=CARTESIAN_POINT('Ctrl Pts',(0.115720369404362,3.23007025084176,52.7612400745245));
#20985=CARTESIAN_POINT('Ctrl Pts',(-0.131288548408443,3.22947345281254,
52.7748564860493));
#20986=CARTESIAN_POINT('Ctrl Pts',(-0.428791399848154,3.1945423148272,52.7925177033988));
#20987=CARTESIAN_POINT('Ctrl Pts',(-0.481601971918925,3.18700827166916,
52.7956982944682));
#20988=CARTESIAN_POINT('Ctrl Pts',(-0.565963785330671,3.17282839992237,
52.8008646722894));
#20989=CARTESIAN_POINT('Ctrl Pts',(-0.597645678632529,3.16701351262686,
52.8028243833263));
#20990=CARTESIAN_POINT('Ctrl Pts',(-0.663881736657569,3.15382729840659,
52.8069650742735));
#20991=CARTESIAN_POINT('Ctrl Pts',(-0.698412332702053,3.14636069853373,
52.8091488228204));
#20992=CARTESIAN_POINT('Ctrl Pts',(-0.782249639706248,3.12678435270964,
52.8145150367139));
#20993=CARTESIAN_POINT('Ctrl Pts',(-0.831405055510819,3.11407451040364,
52.8177161076703));
#20994=CARTESIAN_POINT('Ctrl Pts',(-1.06065445156192,3.04898408726272,52.8329117769836));
#20995=CARTESIAN_POINT('Ctrl Pts',(-1.23622932652036,2.98211504929666,52.8453599631252));
#20996=CARTESIAN_POINT('Ctrl Pts',(-1.59146554086719,2.81003490002589,52.8719588807387));
#20997=CARTESIAN_POINT('Ctrl Pts',(-1.76882088892803,2.70191438283583,52.8860910360824));
#20998=CARTESIAN_POINT('Ctrl Pts',(-1.96245645060557,2.5565792913504,52.9017354665703));
#20999=CARTESIAN_POINT('Ctrl Pts',(-1.98999928313984,2.53519941496186,52.9039653412491));
#21000=CARTESIAN_POINT('Ctrl Pts',(-2.03348107111656,2.50030170086807,52.9074860028827));
#21001=CARTESIAN_POINT('Ctrl Pts',(-2.04964418822886,2.48706908228006,52.9087947874549));
#21002=CARTESIAN_POINT('Ctrl Pts',(-2.0816962826965,2.46030357032108,52.9113883518853));
#21003=CARTESIAN_POINT('Ctrl Pts',(-2.09758475026516,2.4467716162721,52.9126730873425));
#21004=CARTESIAN_POINT('Ctrl Pts',(-2.13959235093509,2.41028445697734,52.916070820585));
#21005=CARTESIAN_POINT('Ctrl Pts',(-2.16547402154489,2.387058665748,52.9181652967321));
#21006=CARTESIAN_POINT('Ctrl Pts',(-2.22317772161475,2.3335651908511,52.9228510067565));
#21007=CARTESIAN_POINT('Ctrl Pts',(-2.25476754614464,2.3030565205436,52.9254276769711));
#21008=CARTESIAN_POINT('Ctrl Pts',(-2.35881271992539,2.198378676343,52.9339935554121));
#21009=CARTESIAN_POINT('Ctrl Pts',(-2.42831349264826,2.12135858208016,52.9398509016356));
#21010=CARTESIAN_POINT('Ctrl Pts',(-2.64591400805072,1.85547876684069,52.9591453033921));
#21011=CARTESIAN_POINT('Ctrl Pts',(-2.77662998547973,1.653474713881,52.9724311691208));
#21012=CARTESIAN_POINT('Ctrl Pts',(-2.90791878081266,1.39034650197362,52.9897555740468));
#21013=CARTESIAN_POINT('Ctrl Pts',(-2.93088808779307,1.34124924735414,52.9929852924918));
#21014=CARTESIAN_POINT('Ctrl Pts',(-2.96701069260175,1.25867257769772,52.9984262533494));
#21015=CARTESIAN_POINT('Ctrl Pts',(-2.98086155545157,1.22550941849734,53.0006136401906));
#21016=CARTESIAN_POINT('Ctrl Pts',(-3.00740145346462,1.15885137667292,53.0050182579616));
#21017=CARTESIAN_POINT('Ctrl Pts',(-3.02009244678333,1.12536281481107,53.0072350439398));
#21018=CARTESIAN_POINT('Ctrl Pts',(-3.05034677819123,1.04132844856807,53.0128104553458));
#21019=CARTESIAN_POINT('Ctrl Pts',(-3.06721374790806,0.990545146567159,
53.0161912120146));
#21020=CARTESIAN_POINT('Ctrl Pts',(-3.10126486782354,0.878796517847917,
53.0236592817187));
#21021=CARTESIAN_POINT('Ctrl Pts',(-3.11793146420971,0.81769777873726,53.0277608628059));
#21022=CARTESIAN_POINT('Ctrl Pts',(-3.19270799141907,0.507893286975151,
53.0486411883242));
#21023=CARTESIAN_POINT('Ctrl Pts',(-3.22290049581669,0.253411023710327,
53.0661558434012));
#21024=CARTESIAN_POINT('Ctrl Pts',(-3.2227494359304,-0.00190675388112439,
53.0831681868229));
#21025=CARTESIAN_POINT('Ctrl Pts',(-3.22274943328784,-0.00191121505285077,
53.0831684840798));
#21026=CARTESIAN_POINT('Ctrl Pts',(-3.22271772432663,-0.0553798378646609,
53.0867312056951));
#21027=CARTESIAN_POINT('Ctrl Pts',(-3.22135536909969,-0.108842478347912,
53.0902648959406));
#21028=CARTESIAN_POINT('Ctrl Pts',(-3.21686196289615,-0.197981605506103,
53.096084777586));
#21029=CARTESIAN_POINT('Ctrl Pts',(-3.2144657519642,-0.233683025948998,
53.0983963781368));
#21030=CARTESIAN_POINT('Ctrl Pts',(-3.20975897216,-0.289804597775859,53.1019922981067));
#21031=CARTESIAN_POINT('Ctrl Pts',(-3.20784689275809,-0.310254293233996,
53.1032946496888));
#21032=CARTESIAN_POINT('Ctrl Pts',(-3.20385690258654,-0.34893422260551,
53.105741222731));
#21033=CARTESIAN_POINT('Ctrl Pts',(-3.20181853808203,-0.367167883617922,
53.1068874336563));
#21034=CARTESIAN_POINT('Ctrl Pts',(-3.19703678975587,-0.406868017816232,
53.109366269031));
#21035=CARTESIAN_POINT('Ctrl Pts',(-3.19423271797125,-0.428326071733101,
53.1106955519831));
#21036=CARTESIAN_POINT('Ctrl Pts',(-3.18583780188757,-0.487891757877464,
53.1143602343152));
#21037=CARTESIAN_POINT('Ctrl Pts',(-3.17977950586519,-0.525931033073054,
53.1166716884514));
#21038=CARTESIAN_POINT('Ctrl Pts',(-3.14112999498181,-0.743427724020373,
53.1297686303432));
#21039=CARTESIAN_POINT('Ctrl Pts',(-3.09402954915463,-0.919987902043252,
53.1399460253711));
#21040=CARTESIAN_POINT('Ctrl Pts',(-2.96298774501041,-1.28398497584804,
53.1616162624548));
#21041=CARTESIAN_POINT('Ctrl Pts',(-2.87560000956937,-1.46929486605143,
53.1730872064711));
#21042=CARTESIAN_POINT('Ctrl Pts',(-2.74504509641757,-1.6892251166233,53.1881952150955));
#21043=CARTESIAN_POINT('Ctrl Pts',(-2.71778441415138,-1.73274392798073,
53.1912617793187));
#21044=CARTESIAN_POINT('Ctrl Pts',(-2.66997802716068,-1.80515649886275,
53.1965078529293));
#21045=CARTESIAN_POINT('Ctrl Pts',(-2.64997365764608,-1.83439693375694,
53.1986672529939));
#21046=CARTESIAN_POINT('Ctrl Pts',(-2.60844584599184,-1.89300102278889,
53.2030825077528));
#21047=CARTESIAN_POINT('Ctrl Pts',(-2.58689880660851,-1.92234153996346,
53.2053390570679));
#21048=CARTESIAN_POINT('Ctrl Pts',(-2.53054050729678,-1.99642057506568,
53.2111586017881));
#21049=CARTESIAN_POINT('Ctrl Pts',(-2.4950386409874,-2.04061557113202,53.2147480313735));
#21050=CARTESIAN_POINT('Ctrl Pts',(-2.31779890900502,-2.2497116196632,53.2323194259474));
#21051=CARTESIAN_POINT('Ctrl Pts',(-2.16080106458157,-2.40089702043185,
53.2469103446982));
#21052=CARTESIAN_POINT('Ctrl Pts',(-1.85752879741484,-2.63893599177738,
53.2729532070226));
#21053=CARTESIAN_POINT('Ctrl Pts',(-1.71731185694977,-2.73226020121365,
53.2843121299865));
#21054=CARTESIAN_POINT('Ctrl Pts',(-1.5415397390561,-2.83034772081998,53.2972929166255));
#21055=CARTESIAN_POINT('Ctrl Pts',(-1.51239002097139,-2.84603050042357,
53.2994062133198));
#21056=CARTESIAN_POINT('Ctrl Pts',(-1.46477749536448,-2.87070824632975,
53.3027885350636));
#21057=CARTESIAN_POINT('Ctrl Pts',(-1.44646178158218,-2.87998043990741,
53.3040732818903));
#21058=CARTESIAN_POINT('Ctrl Pts',(-1.40898335572586,-2.89850585647834,
53.3066671423694));
#21059=CARTESIAN_POINT('Ctrl Pts',(-1.38981528382808,-2.90774548959518,
53.3079754779408));
#21060=CARTESIAN_POINT('Ctrl Pts',(-1.33729906453871,-2.9324220430405,53.3115141862648));
#21061=CARTESIAN_POINT('Ctrl Pts',(-1.30377521447105,-2.94747998672584,
53.3137232423185));
#21062=CARTESIAN_POINT('Ctrl Pts',(-1.09744848097736,-3.03594664262729,
53.3270599832969));
#21063=CARTESIAN_POINT('Ctrl Pts',(-0.91874247139775,-3.09472019893946,
53.3375269287872));
#21064=CARTESIAN_POINT('Ctrl Pts',(-0.654739885777959,-3.15664153724001,
53.3527166130787));
#21065=CARTESIAN_POINT('Ctrl Pts',(-0.572898969281294,-3.17251338916061,
53.3573865382102));
#21066=CARTESIAN_POINT('Ctrl Pts',(-0.490581732222734,-3.18519185081674,
53.3621044196136));
#21067=CARTESIAN_POINT('',(-3.22274878139355,0.00280259281299765,53.3277091182931));
#21068=CARTESIAN_POINT('Ctrl Pts',(-0.490582106922522,-3.18519179310563,
53.6117903092821));
#21069=CARTESIAN_POINT('Ctrl Pts',(-0.542014919510384,-3.17727012960677,
53.6087878737367));
#21070=CARTESIAN_POINT('Ctrl Pts',(-0.593275039676424,-3.16809975755217,
53.6057559209604));
#21071=CARTESIAN_POINT('Ctrl Pts',(-0.697634432052406,-3.14680549719471,
53.5994822420388));
#21072=CARTESIAN_POINT('Ctrl Pts',(-0.750664989935348,-3.13457815352351,
53.5962400949983));
#21073=CARTESIAN_POINT('Ctrl Pts',(-0.838201641574686,-3.11204596025405,
53.5907841464142));
#21074=CARTESIAN_POINT('Ctrl Pts',(-0.87289108300727,-3.10249464900551,
53.5885944928083));
#21075=CARTESIAN_POINT('Ctrl Pts',(-0.941740120137199,-3.08229183778636,
53.5841899883102));
#21076=CARTESIAN_POINT('Ctrl Pts',(-0.975896674804988,-3.07164824554058,
53.5819756621852));
#21077=CARTESIAN_POINT('Ctrl Pts',(-1.06048476309417,-3.04373629956317,
53.5764158496298));
#21078=CARTESIAN_POINT('Ctrl Pts',(-1.11067689086895,-3.02578170096815,
53.5730485014055));
#21079=CARTESIAN_POINT('Ctrl Pts',(-1.34001434028316,-2.93726857360369,
53.5573364486652));
#21080=CARTESIAN_POINT('Ctrl Pts',(-1.5130314919546,-2.85199950145234,53.5445188741822));
#21081=CARTESIAN_POINT('Ctrl Pts',(-1.84303283713041,-2.65084565155453,
53.5184485190678));
#21082=CARTESIAN_POINT('Ctrl Pts',(-1.99923645699547,-2.53511652309719,
53.5052505247895));
#21083=CARTESIAN_POINT('Ctrl Pts',(-2.17119508503107,-2.38187901746128,
53.4903444127689));
#21084=CARTESIAN_POINT('Ctrl Pts',(-2.19789219749092,-2.35726661471363,
53.4880191149323));
#21085=CARTESIAN_POINT('Ctrl Pts',(-2.23950172106203,-2.31758462999663,
53.4843850485082));
#21086=CARTESIAN_POINT('Ctrl Pts',(-2.2546904625627,-2.30281077217671,53.4830563438441));
#21087=CARTESIAN_POINT('Ctrl Pts',(-2.28435786558828,-2.27337878579174,
53.4804587726769));
#21088=CARTESIAN_POINT('Ctrl Pts',(-2.29884370906879,-2.25872964319822,
53.4791894359282));
#21089=CARTESIAN_POINT('Ctrl Pts',(-2.33648500443717,-2.21992676938085,
53.4758851561427));
#21090=CARTESIAN_POINT('Ctrl Pts',(-2.35940721955533,-2.19554886255723,
53.4738669397837));
#21091=CARTESIAN_POINT('Ctrl Pts',(-2.41003588117067,-2.13999616012176,
53.4693834933687));
#21092=CARTESIAN_POINT('Ctrl Pts',(-2.43752551789892,-2.10863134854571,
53.4669309945015));
#21093=CARTESIAN_POINT('Ctrl Pts',(-2.52550648138278,-2.00422722741648,
53.4589876534119));
#21094=CARTESIAN_POINT('Ctrl Pts',(-2.58338646591933,-1.9290479896424,53.4536091394));
#21095=CARTESIAN_POINT('Ctrl Pts',(-2.78507248332578,-1.64168971448005,
53.4338519998825));
#21096=CARTESIAN_POINT('Ctrl Pts',(-2.90672641004,-1.41517026243518,53.4197251268083));
#21097=CARTESIAN_POINT('Ctrl Pts',(-3.01959072066893,-1.12738148000629,
53.4014916866001));
#21098=CARTESIAN_POINT('Ctrl Pts',(-3.0376918180448,-1.07765721281974,53.3983356144902));
#21099=CARTESIAN_POINT('Ctrl Pts',(-3.06480770888264,-0.997047815542967,
53.3931980953715));
#21100=CARTESIAN_POINT('Ctrl Pts',(-3.0745987976094,-0.966433007509562,
53.3912421439505));
#21101=CARTESIAN_POINT('Ctrl Pts',(-3.09420701175458,-0.901805666908098,
53.3871005917486));
#21102=CARTESIAN_POINT('Ctrl Pts',(-3.10392485207667,-0.867767738204134,
53.3849120876854));
#21103=CARTESIAN_POINT('Ctrl Pts',(-3.12631366810605,-0.784154451084484,
53.379515579172));
#21104=CARTESIAN_POINT('Ctrl Pts',(-3.13836806270366,-0.734425477669683,
53.3762884692533));
#21105=CARTESIAN_POINT('Ctrl Pts',(-3.19830959240318,-0.458620681204706,
53.3582846235088));
#21106=CARTESIAN_POINT('Ctrl Pts',(-3.22294714079275,-0.228227449020224,
53.3427859443142));
#21107=CARTESIAN_POINT('Ctrl Pts',(-3.22274881214297,0.00276700761489099,
53.3271823260263));
#21108=CARTESIAN_POINT('Ctrl Pts',(-3.22274878139355,0.00280259281299765,
53.3277091182931));
#21109=CARTESIAN_POINT('Ctrl Pts',(-3.22262670745773,0.143177472133502,
53.3190327436128));
#21110=CARTESIAN_POINT('Ctrl Pts',(-3.21332957379828,0.283164167668086,
53.3103563689325));
#21111=CARTESIAN_POINT('Ctrl Pts',(-3.19502939606302,0.421787530390862,
53.3016799942521));
#21112=CARTESIAN_POINT('Ctrl Pts',(-3.18475329542461,0.499628721158624,
53.296807948708));
#21113=CARTESIAN_POINT('Ctrl Pts',(-3.17163920981312,0.577040641109694,
53.2919359031639));
#21114=CARTESIAN_POINT('Ctrl Pts',(-3.15572373989173,0.653854142744276,
53.2870638576197));
#21115=CARTESIAN_POINT('Ctrl Pts',(-3.13554371359198,0.751249852127526,
53.2808863455702));
#21116=CARTESIAN_POINT('Ctrl Pts',(-3.11081578012451,0.8478782970476,53.2747088335206));
#21117=CARTESIAN_POINT('Ctrl Pts',(-3.08161241256265,0.943282832049788,
53.268531321471));
#21118=CARTESIAN_POINT('Ctrl Pts',(-3.05244806418123,1.03855989521991,53.262362063314));
#21119=CARTESIAN_POINT('Ctrl Pts',(-3.01882029357804,1.13261588800971,53.2561928051569));
#21120=CARTESIAN_POINT('Ctrl Pts',(-2.98085259523344,1.22500423182539,53.2500235469999));
#21121=CARTESIAN_POINT('Ctrl Pts',(-2.94292446595288,1.317296290629,53.2438607183021));
#21122=CARTESIAN_POINT('Ctrl Pts',(-2.90066556548995,1.40792375713449,53.2376978896043));
#21123=CARTESIAN_POINT('Ctrl Pts',(-2.85424892698835,1.4964560218349,53.2315350609066));
#21124=CARTESIAN_POINT('Ctrl Pts',(-2.8078653971926,1.5849251370095,53.225376628117));
#21125=CARTESIAN_POINT('Ctrl Pts',(-2.75733022663391,1.67130163902001,53.2192181953275));
#21126=CARTESIAN_POINT('Ctrl Pts',(-2.70286383602891,1.75517652855407,53.213059762538));
#21127=CARTESIAN_POINT('Ctrl Pts',(-2.64841743736294,1.8390206317324,53.2069035902069));
#21128=CARTESIAN_POINT('Ctrl Pts',(-2.59004292187591,1.92036458391123,53.2007474178758));
#21129=CARTESIAN_POINT('Ctrl Pts',(-2.52800531551196,1.99882632743402,53.1945912455447));
#21130=CARTESIAN_POINT('Ctrl Pts',(-2.46597396908345,2.07728015373565,53.1884356944052));
#21131=CARTESIAN_POINT('Ctrl Pts',(-2.40028053564343,2.15285200967157,53.1822801432658));
#21132=CARTESIAN_POINT('Ctrl Pts',(-2.33123118856794,2.22519183621281,53.1761245921263));
#21133=CARTESIAN_POINT('Ctrl Pts',(-2.26217043203404,2.29754361591912,53.1699680238664));
#21134=CARTESIAN_POINT('Ctrl Pts',(-2.18975295971744,2.36666199184607,53.1638114556064));
#21135=CARTESIAN_POINT('Ctrl Pts',(-2.11432204988025,2.43223350685954,53.1576548873465));
#21136=CARTESIAN_POINT('Ctrl Pts',(-2.03881132895827,2.49787440104071,53.1514918050144));
#21137=CARTESIAN_POINT('Ctrl Pts',(-1.9602811318023,2.55996065599349,53.1453287226823));
#21138=CARTESIAN_POINT('Ctrl Pts',(-1.87910798997542,2.6182189985772,53.1391656403501));
#21139=CARTESIAN_POINT('Ctrl Pts',(-1.79788902548743,2.67651022829857,53.1329990789259));
#21140=CARTESIAN_POINT('Ctrl Pts',(-1.71402450854919,2.73096900614671,53.1268325175018));
#21141=CARTESIAN_POINT('Ctrl Pts',(-1.6279183862366,2.78136644300115,53.1206659560776));
#21142=CARTESIAN_POINT('Ctrl Pts',(-1.54167251566397,2.83184567373878,53.1144893864658));
#21143=CARTESIAN_POINT('Ctrl Pts',(-1.45317815752836,2.87825019745168,53.1083128168539));
#21144=CARTESIAN_POINT('Ctrl Pts',(-1.36286225037172,2.92039792648395,53.1021362472421));
#21145=CARTESIAN_POINT('Ctrl Pts',(-1.30153121563375,2.94901928361566,53.0979419096403));
#21146=CARTESIAN_POINT('Ctrl Pts',(-1.23936062752267,2.97567866694849,53.0937475720386));
#21147=CARTESIAN_POINT('Ctrl Pts',(-1.17648823748014,3.0003321465416,53.0895532344368));
#21148=CARTESIAN_POINT('Ctrl Pts',(-1.08388844404121,3.03664231570056,53.0833757247975));
#21149=CARTESIAN_POINT('Ctrl Pts',(-0.98944653174153,3.06872416127268,53.0771982151581));
#21150=CARTESIAN_POINT('Ctrl Pts',(-0.893584562560482,3.09638889548028,
53.0710207055188));
#21151=CARTESIAN_POINT('Ctrl Pts',(-0.797850676486028,3.12401666627966,
53.0648514497744));
#21152=CARTESIAN_POINT('Ctrl Pts',(-0.700700917939257,3.14723893772386,
53.0586821940301));
#21153=CARTESIAN_POINT('Ctrl Pts',(-0.602576792875929,3.16591515539936,
53.0525129382857));
#21154=CARTESIAN_POINT('Ctrl Pts',(-0.504554930552762,3.18457190914391,
53.0463501119999));
#21155=CARTESIAN_POINT('Ctrl Pts',(-0.405561144255584,3.19869194827091,
53.0401872857141));
#21156=CARTESIAN_POINT('Ctrl Pts',(-0.306050630364382,3.2081849345313,53.0340244594283));
#21157=CARTESIAN_POINT('Ctrl Pts',(-0.206611096568207,3.21767114951656,
53.0278660290398));
#21158=CARTESIAN_POINT('Ctrl Pts',(-0.106655998286694,3.22253683273671,
53.0217075986512));
#21159=CARTESIAN_POINT('Ctrl Pts',(-0.00664832232328756,3.22274314246579,
53.0155491682627));
#21160=CARTESIAN_POINT('Ctrl Pts',(0.0933226458389801,3.22294937646892,
53.0093929983251));
#21161=CARTESIAN_POINT('Ctrl Pts',(0.19334572030702,3.21849963457444,53.0032368283874));
#21162=CARTESIAN_POINT('Ctrl Pts',(0.292956109397393,3.20940715404991,52.9970806584497));
#21163=CARTESIAN_POINT('Ctrl Pts',(0.392556447416537,3.20031559099162,52.9909251096933));
#21164=CARTESIAN_POINT('Ctrl Pts',(0.491743751176398,3.1865822602719,52.9847695609368));
#21165=CARTESIAN_POINT('Ctrl Pts',(0.590057548787154,3.16827234492543,52.9786140121804));
#21166=CARTESIAN_POINT('Ctrl Pts',(0.688387591623784,3.14995940407574,52.9724574462902));
#21167=CARTESIAN_POINT('Ctrl Pts',(0.785843415434532,3.1270684558414,52.9663008804));
#21168=CARTESIAN_POINT('Ctrl Pts',(0.881974932271338,3.09971575815347,52.9601443145098));
#21169=CARTESIAN_POINT('Ctrl Pts',(0.978208163440187,3.07233411926638,52.9539812345126));
#21170=CARTESIAN_POINT('Ctrl Pts',(1.07311387208691,3.04048142343067,52.9478181545155));
#21171=CARTESIAN_POINT('Ctrl Pts',(1.16625745873088,3.0043237346289,52.9416550745183));
#21172=CARTESIAN_POINT('Ctrl Pts',(1.25945362567591,2.96814563452206,52.935488515413));
#21173=CARTESIAN_POINT('Ctrl Pts',(1.35088529327482,2.92765787710775,52.9293219563078));
#21174=CARTESIAN_POINT('Ctrl Pts',(1.44014005775924,2.88307373761705,52.9231553972026));
#21175=CARTESIAN_POINT('Ctrl Pts',(1.52953968144246,2.83841723870933,52.9169788298606));
#21176=CARTESIAN_POINT('Ctrl Pts',(1.61675496724579,2.78965129091158,52.9108022625187));
#21177=CARTESIAN_POINT('Ctrl Pts',(1.7014001489357,2.73703399608071,52.9046256951767));
#21178=CARTESIAN_POINT('Ctrl Pts',(1.75888069683518,2.70130283128805,52.9004313338691));
#21179=CARTESIAN_POINT('Ctrl Pts',(1.81517665591439,2.66379654871379,52.8962369725616));
#21180=CARTESIAN_POINT('Ctrl Pts',(1.87017596998735,2.62460652361108,52.892042611254));
#21181=CARTESIAN_POINT('Ctrl Pts',(1.95117970363851,2.56688692458135,52.88586509919));
#21182=CARTESIAN_POINT('Ctrl Pts',(2.02964841309519,2.50531430026754,52.879687587126));
#21183=CARTESIAN_POINT('Ctrl Pts',(2.10519338421395,2.44013900783578,52.8735100750621));
#21184=CARTESIAN_POINT('Ctrl Pts',(2.18063741804477,2.37505079753749,52.867340816907));
#21185=CARTESIAN_POINT('Ctrl Pts',(2.25316515312644,2.30636976803818,52.861171558752));
#21186=CARTESIAN_POINT('Ctrl Pts',(2.32241765031869,2.23438891421976,52.855002300597));
#21187=CARTESIAN_POINT('Ctrl Pts',(2.3915979739655,2.16248307738463,52.8488394719175));
#21188=CARTESIAN_POINT('Ctrl Pts',(2.45750954733497,2.08728456446029,52.842676643238));
#21189=CARTESIAN_POINT('Ctrl Pts',(2.51982801044539,2.00912527241951,52.8365138145585));
#21190=CARTESIAN_POINT('Ctrl Pts',(2.58210202193359,1.93102173122927,52.830355381811));
#21191=CARTESIAN_POINT('Ctrl Pts',(2.64078774953701,1.84996194792784,52.8241969490636));
#21192=CARTESIAN_POINT('Ctrl Pts',(2.69559970826759,1.7663124795142,52.8180385163162));
#21193=CARTESIAN_POINT('Ctrl Pts',(2.75039154808751,1.6826937149145,52.8118823440419));
#21194=CARTESIAN_POINT('Ctrl Pts',(2.80131220720641,1.59648751629959,52.8057261717675));
#21195=CARTESIAN_POINT('Ctrl Pts',(2.84811883367611,1.50809040569833,52.7995699994932));
#21196=CARTESIAN_POINT('Ctrl Pts',(2.89492073698975,1.41970221505949,52.793414448425));
#21197=CARTESIAN_POINT('Ctrl Pts',(2.93760923031824,1.32912393514834,52.7872588973568));
#21198=CARTESIAN_POINT('Ctrl Pts',(2.9759873293797,1.23677685047523,52.7811033462886));
#21199=CARTESIAN_POINT('Ctrl Pts',(3.01437176980688,1.14441450692658,52.7749467781142));
#21200=CARTESIAN_POINT('Ctrl Pts',(3.04844423488406,1.05028317838321,52.7687902099399));
#21201=CARTESIAN_POINT('Ctrl Pts',(3.07805619173572,0.954823356970983,52.7626336417655));
#21202=CARTESIAN_POINT('Ctrl Pts',(3.10769947997009,0.859262532838365,52.7564705595403));
#21203=CARTESIAN_POINT('Ctrl Pts',(3.13287270768393,0.762370823919694,52.750307477315));
#21204=CARTESIAN_POINT('Ctrl Pts',(3.15347751953469,0.664602961390698,52.7441443950898));
#21205=CARTESIAN_POINT('Ctrl Pts',(3.17409396286887,0.566779908584761,52.7379778337845));
#21206=CARTESIAN_POINT('Ctrl Pts',(3.19013678486609,0.468080144975986,52.7318112724793));
#21207=CARTESIAN_POINT('Ctrl Pts',(3.20155929892123,0.368965605430828,52.7256447111741));
#21208=CARTESIAN_POINT('Ctrl Pts',(3.21300035142143,0.269690205549891,52.7194681416992));
#21209=CARTESIAN_POINT('Ctrl Pts',(3.21980608988906,0.169999117734282,52.7132915722244));
#21210=CARTESIAN_POINT('Ctrl Pts',(3.22198192598891,0.0703564574201773,
52.7071150027495));
#21211=CARTESIAN_POINT('Ctrl Pts',(3.22345947636126,0.00269187098393442,
52.7029206645234));
#21212=CARTESIAN_POINT('Ctrl Pts',(3.22280308774812,-0.0649503896133836,
52.6987263262972));
#21213=CARTESIAN_POINT('Ctrl Pts',(3.22002806994389,-0.132426550485002,
52.6945319880711));
#21214=CARTESIAN_POINT('Ctrl Pts',(3.21594096084956,-0.231806968992186,
52.6883544717025));
#21215=CARTESIAN_POINT('Ctrl Pts',(3.20724170618463,-0.331169256470755,
52.6821769553339));
#21216=CARTESIAN_POINT('Ctrl Pts',(3.19392762109117,-0.430051059446254,
52.6759994389653));
#21217=CARTESIAN_POINT('Ctrl Pts',(3.18063132513885,-0.528800745018493,
52.6698301764654));
#21218=CARTESIAN_POINT('Ctrl Pts',(3.16273251235513,-0.627070796217695,
52.6636609139655));
#21219=CARTESIAN_POINT('Ctrl Pts',(3.1402804769695,-0.72440050280501,52.6574916514657));
#21220=CARTESIAN_POINT('Ctrl Pts',(3.11785184049886,-0.821628774957042,
52.6513288184073));
#21221=CARTESIAN_POINT('Ctrl Pts',(3.09087951293835,-0.917918230806609,
52.645165985349));
#21222=CARTESIAN_POINT('Ctrl Pts',(3.05946426354687,-1.0128158680528,52.6390031522906));
#21223=CARTESIAN_POINT('Ctrl Pts',(3.02807142240255,-1.10764581557021,52.632844715132));
#21224=CARTESIAN_POINT('Ctrl Pts',(2.99224209627347,-1.20108550804784,52.6266862779734));
#21225=CARTESIAN_POINT('Ctrl Pts',(2.95212732349995,-1.29269556676929,52.6205278408148));
#21226=CARTESIAN_POINT('Ctrl Pts',(2.91202727485667,-1.38427200001207,52.614371664111));
#21227=CARTESIAN_POINT('Ctrl Pts',(2.86764507901428,-1.47401973734669,52.6082154874072));
#21228=CARTESIAN_POINT('Ctrl Pts',(2.81918016427108,-1.56151873632064,52.6020593107034));
#21229=CARTESIAN_POINT('Ctrl Pts',(2.77072013991374,-1.64900890614737,52.5959037551929));
#21230=CARTESIAN_POINT('Ctrl Pts',(2.71817842590117,-1.73425040963265,52.5897481996823));
#21231=CARTESIAN_POINT('Ctrl Pts',(2.66180025029488,-1.81684809217228,52.5835926441718));
#21232=CARTESIAN_POINT('Ctrl Pts',(2.6054127590379,-1.89945942274416,52.5774360715478));
#21233=CARTESIAN_POINT('Ctrl Pts',(2.54518779139796,-1.9794257065864,52.5712794989237));
#21234=CARTESIAN_POINT('Ctrl Pts',(2.48141313430962,-2.05638187586247,52.5651229262997));
#21235=CARTESIAN_POINT('Ctrl Pts',(2.41757099968903,-2.13341946952608,52.558959839641));
#21236=CARTESIAN_POINT('Ctrl Pts',(2.3501719533757,-2.20744025486283,52.5527967529822));
#21237=CARTESIAN_POINT('Ctrl Pts',(2.27954312278993,-2.27811341110163,52.5466336663235));
#21238=CARTESIAN_POINT('Ctrl Pts',(2.20887442205615,-2.34882646251038,52.5404671005873));
#21239=CARTESIAN_POINT('Ctrl Pts',(2.13497262636165,-2.41618782936041,52.534300534851));
#21240=CARTESIAN_POINT('Ctrl Pts',(2.05819912582431,-2.47990603067052,52.5281339691147));
#21241=CARTESIAN_POINT('Ctrl Pts',(1.9813010245793,-2.54372764439402,52.5219573952579));
#21242=CARTESIAN_POINT('Ctrl Pts',(1.90152225611161,-2.60389402243564,52.515780821401));
#21243=CARTESIAN_POINT('Ctrl Pts',(1.81925450076102,-2.66015612774151,52.5096042475441));
#21244=CARTESIAN_POINT('Ctrl Pts',(1.76338935956113,-2.6983617460147,52.5054099533255));
#21245=CARTESIAN_POINT('Ctrl Pts',(1.70637706542877,-2.73476790802879,52.5012156591069));
#21246=CARTESIAN_POINT('Ctrl Pts',(1.64834639751306,-2.76930888784651,52.4970213648882));
#21247=CARTESIAN_POINT('Ctrl Pts',(1.56289523468098,-2.82017107842255,52.4908451940614));
#21248=CARTESIAN_POINT('Ctrl Pts',(1.47494049959711,-2.86716211889021,52.4846690232346));
#21249=CARTESIAN_POINT('Ctrl Pts',(1.38486771824877,-2.91002731352344,52.4784928524078));
#21250=CARTESIAN_POINT('Ctrl Pts',(1.29490670478629,-2.95283931836826,52.4723243453563));
#21251=CARTESIAN_POINT('Ctrl Pts',(1.2028332546352,-2.99153546474498,52.4661558383048));
#21252=CARTESIAN_POINT('Ctrl Pts',(1.10906001329222,-3.0259053933354,52.4599873312532));
#21253=CARTESIAN_POINT('Ctrl Pts',(1.01537816395696,-3.06024182477104,52.4538248360686));
#21254=CARTESIAN_POINT('Ctrl Pts',(0.920000220491095,-3.09026026975514,
52.4476623408839));
#21255=CARTESIAN_POINT('Ctrl Pts',(0.823360576297346,-3.11579763847065,
52.4414998456993));
#21256=CARTESIAN_POINT('Ctrl Pts',(0.726789391592974,-3.1413169165233,52.435341716024));
#21257=CARTESIAN_POINT('Ctrl Pts',(0.628958700957384,-3.16236131916738,
52.4291835863488));
#21258=CARTESIAN_POINT('Ctrl Pts',(0.53031895751404,-3.17881729040869,52.4230254566735));
#21259=CARTESIAN_POINT('Ctrl Pts',(0.431709789962919,-3.19526816070401,
52.4168692358669));
#21260=CARTESIAN_POINT('Ctrl Pts',(0.332292494402997,-3.20713335100443,
52.4107130150602));
#21261=CARTESIAN_POINT('Ctrl Pts',(0.232527846560202,-3.21435037963724,
52.4045567942536));
#21262=CARTESIAN_POINT('Ctrl Pts',(0.13278130284569,-3.22156609860761,52.3984016906063));
#21263=CARTESIAN_POINT('Ctrl Pts',(0.0326879648162029,-3.22413530683116,
52.392246586959));
#21264=CARTESIAN_POINT('Ctrl Pts',(-0.067287323570641,-3.22204748236067,
52.3860914833117));
#21265=CARTESIAN_POINT('Ctrl Pts',(-0.167298174937415,-3.21995891521405,
52.3799341901851));
#21266=CARTESIAN_POINT('Ctrl Pts',(-0.267190459316207,-3.21321001964345,
52.3737768970585));
#21267=CARTESIAN_POINT('Ctrl Pts',(-0.366501012415672,-3.20184237126038,
52.3676196039319));
#21268=CARTESIAN_POINT('Ctrl Pts',(-0.407973875882795,-3.19709515241385,
52.3650482701794));
#21269=CARTESIAN_POINT('Ctrl Pts',(-0.449345351154687,-3.19154306339272,
52.3624769364268));
#21270=CARTESIAN_POINT('Ctrl Pts',(-0.490582094296232,-3.18519179505033,
52.3599056026743));
#21271=CARTESIAN_POINT('Origin',(-9.35406549764863E-15,0.,41.4527091182931));
#21272=CARTESIAN_POINT('',(-0.490581718709063,-3.18519185289811,50.8612231915357));
#21273=CARTESIAN_POINT('',(-0.49058209429631,-3.18519179505032,51.1068136617517));
#21274=CARTESIAN_POINT('',(-0.490582094296226,-3.18519179505033,41.4527091182931));
#21275=CARTESIAN_POINT('Ctrl Pts',(-0.490581718709059,-3.18519185289811,
50.8612231915357));
#21276=CARTESIAN_POINT('Ctrl Pts',(-0.346603507787341,-3.20736730776321,
50.8708079128671));
#21277=CARTESIAN_POINT('Ctrl Pts',(-0.201224047347916,-3.2197648351351,
50.8806253624206));
#21278=CARTESIAN_POINT('Ctrl Pts',(0.1150624159999,-3.22520666569334,50.9019986000714));
#21279=CARTESIAN_POINT('Ctrl Pts',(0.285543187370928,-3.21460291450712,
50.9135292413597));
#21280=CARTESIAN_POINT('Ctrl Pts',(0.488056539100501,-3.18576120491405,
50.9267353279802));
#21281=CARTESIAN_POINT('Ctrl Pts',(0.521641609968407,-3.18043454307468,
50.9289084276596));
#21282=CARTESIAN_POINT('Ctrl Pts',(0.575570297106993,-3.17100404577209,
50.9323637964471));
#21283=CARTESIAN_POINT('Ctrl Pts',(0.595968704995193,-3.16723367992426,
50.9336628875048));
#21284=CARTESIAN_POINT('Ctrl Pts',(0.634376982659992,-3.1597502221884,50.936092228012));
#21285=CARTESIAN_POINT('Ctrl Pts',(0.652394097027578,-3.15607946690025,
50.9372248275988));
#21286=CARTESIAN_POINT('Ctrl Pts',(0.702356005513021,-3.14545423736711,
50.9403485842437));
#21287=CARTESIAN_POINT('Ctrl Pts',(0.734228799388278,-3.13816739117671,
50.9423220171601));
#21288=CARTESIAN_POINT('Ctrl Pts',(0.926956716171972,-3.09100819109944,
50.9541675753366));
#21289=CARTESIAN_POINT('Ctrl Pts',(1.08466822331222,-3.03925775677906,50.9634977044365));
#21290=CARTESIAN_POINT('Ctrl Pts',(1.43189930086637,-2.89482545794972,50.9845750620373));
#21291=CARTESIAN_POINT('Ctrl Pts',(1.61769665727226,-2.79524588710479,50.9962710778001));
#21292=CARTESIAN_POINT('Ctrl Pts',(1.84387196464562,-2.64387598105526,51.0121969983384));
#21293=CARTESIAN_POINT('Ctrl Pts',(1.89427575841785,-2.60799974044836,51.0158626894327));
#21294=CARTESIAN_POINT('Ctrl Pts',(1.97332125325968,-2.54823621668385,51.021822659834));
#21295=CARTESIAN_POINT('Ctrl Pts',(2.00263616536732,-2.5252629162438,51.0240817384394));
#21296=CARTESIAN_POINT('Ctrl Pts',(2.0584374705346,-2.47995015881982,51.0284812358785));
#21297=CARTESIAN_POINT('Ctrl Pts',(2.08497475014839,-2.45768137749764,51.0306186339193));
#21298=CARTESIAN_POINT('Ctrl Pts',(2.14702063563997,-2.40388731594316,51.0357272300583));
#21299=CARTESIAN_POINT('Ctrl Pts',(2.18220082050033,-2.37199726669711,51.0387132513175));
#21300=CARTESIAN_POINT('Ctrl Pts',(2.3053730472564,-2.25528448618121,51.0494995720332));
#21301=CARTESIAN_POINT('Ctrl Pts',(2.389220932612,-2.16625726332375,51.0574750639635));
#21302=CARTESIAN_POINT('Ctrl Pts',(2.58347978933681,-1.93496740901208,51.0775535106357));
#21303=CARTESIAN_POINT('Ctrl Pts',(2.68741904657515,-1.7878030636864,51.0898063567217));
#21304=CARTESIAN_POINT('Ctrl Pts',(2.83427673859514,-1.53788784604615,51.1092852271069));
#21305=CARTESIAN_POINT('Ctrl Pts',(2.88513103190173,-1.44022461591109,51.1165977823114));
#21306=CARTESIAN_POINT('Ctrl Pts',(2.94360296329596,-1.31234650712155,51.1256407533031));
#21307=CARTESIAN_POINT('Ctrl Pts',(2.95591738980371,-1.2843692243956,51.1275876747268));
#21308=CARTESIAN_POINT('Ctrl Pts',(2.97561886967302,-1.23782427249649,51.1307699319569));
#21309=CARTESIAN_POINT('Ctrl Pts',(2.98323443214233,-1.21935597565351,51.1320179641752));
#21310=CARTESIAN_POINT('Ctrl Pts',(2.99886244208603,-1.18043384541739,51.1346161762013));
#21311=CARTESIAN_POINT('Ctrl Pts',(3.00683829787248,-1.15996703580725,51.1359643526674));
#21312=CARTESIAN_POINT('Ctrl Pts',(3.02878747762368,-1.10189528038919,51.1397430450231));
#21313=CARTESIAN_POINT('Ctrl Pts',(3.0422692744859,-1.06410750346113,51.1421471368228));
#21314=CARTESIAN_POINT('Ctrl Pts',(3.12061738068006,-0.830833547553012,
51.1567111321666));
#21315=CARTESIAN_POINT('Ctrl Pts',(3.16733195316815,-0.629733207815807,
51.1681063791059));
#21316=CARTESIAN_POINT('Ctrl Pts',(3.21651895832334,-0.260478884034092,
51.1889981250994));
#21317=CARTESIAN_POINT('Ctrl Pts',(3.22567868455243,-0.0939853738832021,
51.1984062918477));
#21318=CARTESIAN_POINT('Ctrl Pts',(3.22065257180319,0.129495373666211,51.2115439284476));
#21319=CARTESIAN_POINT('Ctrl Pts',(3.21785579060651,0.186482089594798,51.2149366843071));
#21320=CARTESIAN_POINT('Ctrl Pts',(3.21079058959678,0.279776647418364,51.2205771230478));
#21321=CARTESIAN_POINT('Ctrl Pts',(3.20741426102531,0.316140433246197,51.2227971000573));
#21322=CARTESIAN_POINT('Ctrl Pts',(3.19958700258732,0.387284891404672,51.2271861862824));
#21323=CARTESIAN_POINT('Ctrl Pts',(3.19518494281967,0.422065874680274,51.2293534789949));
#21324=CARTESIAN_POINT('Ctrl Pts',(3.18299535808989,0.50720207704881,51.2347143525462));
#21325=CARTESIAN_POINT('Ctrl Pts',(3.17457956266573,0.557456302039472,51.2379270350474));
#21326=CARTESIAN_POINT('Ctrl Pts',(3.11563230704754,0.864568132425557,51.257868077414));
#21327=CARTESIAN_POINT('Ctrl Pts',(3.03515583084424,1.11464158858787,51.27555112519));
#21328=CARTESIAN_POINT('Ctrl Pts',(2.88623442755968,1.43682427464072,51.2994778972471));
#21329=CARTESIAN_POINT('Ctrl Pts',(2.84345176478616,1.51973580875641,51.3057347663267));
#21330=CARTESIAN_POINT('Ctrl Pts',(2.77661474829883,1.63653122452382,51.3145955464418));
#21331=CARTESIAN_POINT('Ctrl Pts',(2.75540952640791,1.6719876049724,51.3172917694867));
#21332=CARTESIAN_POINT('Ctrl Pts',(2.71592255916043,1.73521955886606,51.3220990328241));
#21333=CARTESIAN_POINT('Ctrl Pts',(2.69788166009409,1.76313839828696,51.3242211714526));
#21334=CARTESIAN_POINT('Ctrl Pts',(2.66796672148072,1.80789804311074,51.3276164868225));
#21335=CARTESIAN_POINT('Ctrl Pts',(2.65635780657193,1.82491233640051,51.3289054704183));
#21336=CARTESIAN_POINT('Ctrl Pts',(2.63240932739258,1.85929897064144,51.3315052694796));
#21337=CARTESIAN_POINT('Ctrl Pts',(2.62005909514223,1.87666244326464,51.3328153336423));
#21338=CARTESIAN_POINT('Ctrl Pts',(2.58590029482987,1.92369249444011,51.3363600838525));
#21339=CARTESIAN_POINT('Ctrl Pts',(2.5637534790662,1.95311072473937,51.3385733875717));
#21340=CARTESIAN_POINT('Ctrl Pts',(2.42667250734329,2.1288483460997,51.3518136277443));
#21341=CARTESIAN_POINT('Ctrl Pts',(2.29973613525833,2.26538379113368,51.3621933499323));
#21342=CARTESIAN_POINT('Ctrl Pts',(2.01063772102105,2.52684504155757,51.384030565213));
#21343=CARTESIAN_POINT('Ctrl Pts',(1.84696527851101,2.64883337279974,51.395463614612));
#21344=CARTESIAN_POINT('Ctrl Pts',(1.62901682843735,2.78119683519003,51.410527483014));
#21345=CARTESIAN_POINT('Ctrl Pts',(1.58452130994426,2.80678525154454,51.4135928571634));
#21346=CARTESIAN_POINT('Ctrl Pts',(1.50830482397528,2.84822571859362,51.418838267375));
#21347=CARTESIAN_POINT('Ctrl Pts',(1.47689808388018,2.86463698952662,51.4209982456831));
#21348=CARTESIAN_POINT('Ctrl Pts',(1.41266704353984,2.89686321598575,51.4254159398403));
#21349=CARTESIAN_POINT('Ctrl Pts',(1.37983247801889,2.91264601838906,51.4276743714946));
#21350=CARTESIAN_POINT('Ctrl Pts',(1.29516182583676,2.95159217654632,51.4335016314827));
#21351=CARTESIAN_POINT('Ctrl Pts',(1.24297011679141,2.97394774250894,51.4370969994106));
#21352=CARTESIAN_POINT('Ctrl Pts',(0.988677768890194,3.0750068848551,51.454639813883));
#21353=CARTESIAN_POINT('Ctrl Pts',(0.779595516522362,3.13454234023561,51.4691922759406));
#21354=CARTESIAN_POINT('Ctrl Pts',(0.39979282705659,3.20231809729583,51.4952551462515));
#21355=CARTESIAN_POINT('Ctrl Pts',(0.231338474068705,3.2188767490565,51.506672442795));
#21356=CARTESIAN_POINT('Ctrl Pts',(0.0293193802694555,3.22278597400439,
51.5197022294294));
#21357=CARTESIAN_POINT('Ctrl Pts',(-0.00372164682127379,3.22291721981298,
51.5218116568994));
#21358=CARTESIAN_POINT('Ctrl Pts',(-0.0572742518132538,3.2223063324279,
51.5251893829077));
#21359=CARTESIAN_POINT('Ctrl Pts',(-0.077786379463264,3.22187643959687,
51.5264733312751));
#21360=CARTESIAN_POINT('Ctrl Pts',(-0.119561239700812,3.22060171287252,
51.5290663577978));
#21361=CARTESIAN_POINT('Ctrl Pts',(-0.14082231175952,3.21974213535921,51.5303746427153));
#21362=CARTESIAN_POINT('Ctrl Pts',(-0.198812265089489,3.21682209151492,
51.5339156026212));
#21363=CARTESIAN_POINT('Ctrl Pts',(-0.235517922746272,3.21434320657835,
51.5361268811256));
#21364=CARTESIAN_POINT('Ctrl Pts',(-0.458029135002967,3.19548382103351,
51.5493923809504));
#21365=CARTESIAN_POINT('Ctrl Pts',(-0.642186449231802,3.16362442705648,
51.5597945833701));
#21366=CARTESIAN_POINT('Ctrl Pts',(-1.01918283315119,3.06410422450463,51.5816340366025));
#21367=CARTESIAN_POINT('Ctrl Pts',(-1.21042222813626,2.99371599481762,51.5930465330263));
#21368=CARTESIAN_POINT('Ctrl Pts',(-1.44004501231891,2.88357842866269,51.6080893068275));
#21369=CARTESIAN_POINT('Ctrl Pts',(-1.48580352517005,2.86026950510811,51.6111558005791));
#21370=CARTESIAN_POINT('Ctrl Pts',(-1.56214170148145,2.81905739919269,51.6164006095534));
#21371=CARTESIAN_POINT('Ctrl Pts',(-1.59301917340379,2.80172466075089,51.6185587832939));
#21372=CARTESIAN_POINT('Ctrl Pts',(-1.65501558965293,2.76556744084902,51.6229704193284));
#21373=CARTESIAN_POINT('Ctrl Pts',(-1.6861139120703,2.74671796440172,51.6252245574796));
#21374=CARTESIAN_POINT('Ctrl Pts',(-1.76476684405288,2.69720534457655,51.631035075565));
#21375=CARTESIAN_POINT('Ctrl Pts',(-1.81184340207097,2.66580973280929,51.6346177844948));
#21376=CARTESIAN_POINT('Ctrl Pts',(-2.03673184592032,2.50712109071081,51.6522606835108));
#21377=CARTESIAN_POINT('Ctrl Pts',(-2.20207695971448,2.36321030941291,51.6669386121071));
#21378=CARTESIAN_POINT('Ctrl Pts',(-2.46596731120831,2.08161405691009,51.69300981072));
#21379=CARTESIAN_POINT('Ctrl Pts',(-2.57070504651076,1.95079388933501,51.7043098415843));
#21380=CARTESIAN_POINT('Ctrl Pts',(-2.68341493073205,1.78507579751925,51.7172344133315));
#21381=CARTESIAN_POINT('Ctrl Pts',(-2.70159267324075,1.75744374533985,51.7193460893101));
#21382=CARTESIAN_POINT('Ctrl Pts',(-2.7303511136458,1.71222695149777,51.7227258778065));
#21383=CARTESIAN_POINT('Ctrl Pts',(-2.7411945696428,1.69481289319038,51.7240097005034));
#21384=CARTESIAN_POINT('Ctrl Pts',(-2.76294500248613,1.65912783394793,51.7266025944916));
#21385=CARTESIAN_POINT('Ctrl Pts',(-2.77383868125454,1.64085017146012,51.7279108788143));
#21386=CARTESIAN_POINT('Ctrl Pts',(-2.80304538038821,1.59072426953281,51.731448954046));
#21387=CARTESIAN_POINT('Ctrl Pts',(-2.82099667124735,1.55866774595962,51.733657445387));
#21388=CARTESIAN_POINT('Ctrl Pts',(-2.9465997406804,1.32509043253427,51.749413133658));
#21389=CARTESIAN_POINT('Ctrl Pts',(-3.03311178645538,1.11291174552003,51.761975992925));
#21390=CARTESIAN_POINT('Ctrl Pts',(-3.12715878885688,0.786931921859993,
51.7810388781258));
#21391=CARTESIAN_POINT('Ctrl Pts',(-3.15235230131314,0.679011595659373,
51.7873069667753));
#21392=CARTESIAN_POINT('Ctrl Pts',(-3.18595249730045,0.492037487787791,
51.7982993464871));
#21393=CARTESIAN_POINT('Ctrl Pts',(-3.19708423195664,0.413576107576438,
51.8029506050496));
#21394=CARTESIAN_POINT('Ctrl Pts',(-3.20952927375639,0.29442544989722,51.8101175680425));
#21395=CARTESIAN_POINT('Ctrl Pts',(-3.21298216889166,0.253987917458752,
51.8125676195864));
#21396=CARTESIAN_POINT('Ctrl Pts',(-3.21771480389859,0.182705541190045,
51.8169226661762));
#21397=CARTESIAN_POINT('Ctrl Pts',(-3.21931672008742,0.151886886554207,
51.8188173963318));
#21398=CARTESIAN_POINT('Ctrl Pts',(-3.22200518489214,0.0803620702082446,
51.8232443299988));
#21399=CARTESIAN_POINT('Ctrl Pts',(-3.22276327758165,0.0396495831764976,
51.82578640537));
#21400=CARTESIAN_POINT('Ctrl Pts',(-3.22272338396855,-0.0810807397634633,
51.8333946720167));
#21401=CARTESIAN_POINT('Ctrl Pts',(-3.21971698248088,-0.161061791120952,
51.8385268269826));
#21402=CARTESIAN_POINT('Ctrl Pts',(-3.20533209376363,-0.353009526920111,
51.8510656580518));
#21403=CARTESIAN_POINT('Ctrl Pts',(-3.19106031479194,-0.464650453387044,
51.8585434419437));
#21404=CARTESIAN_POINT('Ctrl Pts',(-3.131004613375,-0.795664927442708,51.8811449957779));
#21405=CARTESIAN_POINT('Ctrl Pts',(-3.06816503194015,-1.0112582683208,51.8964783897741));
#21406=CARTESIAN_POINT('Ctrl Pts',(-2.96930069525715,-1.25330621883191,
51.9134191186105));
#21407=CARTESIAN_POINT('Ctrl Pts',(-2.95451939493151,-1.28776493137933,
51.9158226554828));
#21408=CARTESIAN_POINT('Ctrl Pts',(-2.93034641479588,-1.34150921001089,
51.9195497804402));
#21409=CARTESIAN_POINT('Ctrl Pts',(-2.92135826160687,-1.36097135862665,
51.9208949327615));
#21410=CARTESIAN_POINT('Ctrl Pts',(-2.90342884304259,-1.3987979188145,51.923498401907));
#21411=CARTESIAN_POINT('Ctrl Pts',(-2.89450603912762,-1.4171695318841,51.9247575849345));
#21412=CARTESIAN_POINT('Ctrl Pts',(-2.87090960728617,-1.46460072022845,
51.9279978236705));
#21413=CARTESIAN_POINT('Ctrl Pts',(-2.8559687982564,-1.49352591214228,51.9299633657896));
#21414=CARTESIAN_POINT('Ctrl Pts',(-2.76662488307548,-1.66024912815791,
51.9412599735414));
#21415=CARTESIAN_POINT('Ctrl Pts',(-2.68268737323053,-1.79271851829971,
51.9501106139534));
#21416=CARTESIAN_POINT('Ctrl Pts',(-2.45045738311239,-2.10615280965664,
51.972005068897));
#21417=CARTESIAN_POINT('Ctrl Pts',(-2.29151660715481,-2.27806122643698,
51.9849552002255));
#21418=CARTESIAN_POINT('Ctrl Pts',(-2.07390624900671,-2.46739874427539,
52.0019366578584));
#21419=CARTESIAN_POINT('Ctrl Pts',(-2.03148992694457,-2.50243718078142,
52.0052128068452));
#21420=CARTESIAN_POINT('Ctrl Pts',(-1.95979693775776,-2.5586355573769,52.0107096367362));
#21421=CARTESIAN_POINT('Ctrl Pts',(-1.93102338649137,-2.58042021217952,
52.0129053629018));
#21422=CARTESIAN_POINT('Ctrl Pts',(-1.87309028198291,-2.62277011839903,
52.0173093869278));
#21423=CARTESIAN_POINT('Ctrl Pts',(-1.84394297457001,-2.64334342139428,
52.0195169432223));
#21424=CARTESIAN_POINT('Ctrl Pts',(-1.77086616487369,-2.69312701778929,
52.0250345151969));
#21425=CARTESIAN_POINT('Ctrl Pts',(-1.72655088265893,-2.72174973819913,
52.0283656720968));
#21426=CARTESIAN_POINT('Ctrl Pts',(-1.62857106013073,-2.781677801534,52.0357029435847));
#21427=CARTESIAN_POINT('Ctrl Pts',(-1.57466414675696,-2.81254460048031,
52.0397224537275));
#21428=CARTESIAN_POINT('Ctrl Pts',(-1.40294072168675,-2.90438768757778,
52.0524687891351));
#21429=CARTESIAN_POINT('Ctrl Pts',(-1.2822384618318,-2.95965705729563,52.0613510735051));
#21430=CARTESIAN_POINT('Ctrl Pts',(-0.978661125312268,-3.07660118106556,
52.0832985959682));
#21431=CARTESIAN_POINT('Ctrl Pts',(-0.792976734036559,-3.12960856421699,
52.0964054959467));
#21432=CARTESIAN_POINT('Ctrl Pts',(-0.567880417754941,-3.17253149297339,
52.1112373287149));
#21433=CARTESIAN_POINT('Ctrl Pts',(-0.531986622331881,-3.17874735268946,
52.113570359628));
#21434=CARTESIAN_POINT('Ctrl Pts',(-0.494189929094215,-3.18463454861332,
52.1159882262296));
#21435=CARTESIAN_POINT('Ctrl Pts',(-0.492386130713441,-3.18491393801041,
52.1161035231083));
#21436=CARTESIAN_POINT('Ctrl Pts',(-0.49058209429419,-3.18519179505064,
52.1162187418821));
#21437=CARTESIAN_POINT('',(-3.22274931785554,-0.00209684566102432,52.0777091182931));
#21438=CARTESIAN_POINT('Ctrl Pts',(-0.490582094296232,-3.18519179505033,
52.3599056026743));
#21439=CARTESIAN_POINT('Ctrl Pts',(-0.589440239020645,-3.16996569916734,
52.353741263183));
#21440=CARTESIAN_POINT('Ctrl Pts',(-0.68752304555204,-3.15014310743925,
52.3475769236916));
#21441=CARTESIAN_POINT('Ctrl Pts',(-0.784379920417554,-3.12583840000499,
52.3414125842003));
#21442=CARTESIAN_POINT('Ctrl Pts',(-0.881301117565013,-3.10151755190703,
52.3352441509945));
#21443=CARTESIAN_POINT('Ctrl Pts',(-0.976994347927334,-3.07270878719306,
52.3290757177888));
#21444=CARTESIAN_POINT('Ctrl Pts',(-1.07102569701638,-3.03957587811698,
52.322907284583));
#21445=CARTESIAN_POINT('Ctrl Pts',(-1.16519852671715,-3.00639311689808,
52.3167295702842));
#21446=CARTESIAN_POINT('Ctrl Pts',(-1.25770408491926,-2.96887339055742,
52.3105518559853));
#21447=CARTESIAN_POINT('Ctrl Pts',(-1.34813007879941,-2.92722784441805,
52.3043741416865));
#21448=CARTESIAN_POINT('Ctrl Pts',(-1.37185933936709,-2.91629937160376,
52.3027530083595));
#21449=CARTESIAN_POINT('Ctrl Pts',(-1.39544553924316,-2.90508702448003,
52.3011318750324));
#21450=CARTESIAN_POINT('Ctrl Pts',(-1.41888154641625,-2.89359512021628,
52.2995107417054));
#21451=CARTESIAN_POINT('Ctrl Pts',(-1.50818724395349,-2.84980384985502,
52.2933332200183));
#21452=CARTESIAN_POINT('Ctrl Pts',(-1.59561763230012,-2.80179885452189,
52.2871556983311));
#21453=CARTESIAN_POINT('Ctrl Pts',(-1.68074848388976,-2.74976400740178,
52.280978176644));
#21454=CARTESIAN_POINT('Ctrl Pts',(-1.76576558933375,-2.69779868576144,
52.2748089089478));
#21455=CARTESIAN_POINT('Ctrl Pts',(-1.84848889858135,-2.64181443927142,
52.2686396412516));
#21456=CARTESIAN_POINT('Ctrl Pts',(-1.92851663570881,-2.58204205006317,
52.2624703735555));
#21457=CARTESIAN_POINT('Ctrl Pts',(-2.00846096847379,-2.52233195523178,
52.2563075354281));
#21458=CARTESIAN_POINT('Ctrl Pts',(-2.08571496917602,-2.45884182514739,
52.2501446973007));
#21459=CARTESIAN_POINT('Ctrl Pts',(-2.15990466079608,-2.39184644548337,
52.2439818591733));
#21460=CARTESIAN_POINT('Ctrl Pts',(-2.23404143102699,-2.32489885532327,
52.2378234171547));
#21461=CARTESIAN_POINT('Ctrl Pts',(-2.305117917431,-2.25445127668952,52.231664975136));
#21462=CARTESIAN_POINT('Ctrl Pts',(-2.37279286988877,-2.18081901108393,
52.2255065331174));
#21463=CARTESIAN_POINT('Ctrl Pts',(-2.44044298084045,-2.10721377374076,
52.2193503516837));
#21464=CARTESIAN_POINT('Ctrl Pts',(-2.50469374599709,-2.0304264912499,52.21319417025));
#21465=CARTESIAN_POINT('Ctrl Pts',(-2.56524111306123,-1.95080895896048,
52.2070379888162));
#21466=CARTESIAN_POINT('Ctrl Pts',(-2.62578236922915,-1.87119946227195,
52.2008824287107));
#21467=CARTESIAN_POINT('Ctrl Pts',(-2.68262070816888,-1.78876062884767,
52.1947268686052));
#21468=CARTESIAN_POINT('Ctrl Pts',(-2.735493312346,-1.70387614004375,52.1885713084996));
#21469=CARTESIAN_POINT('Ctrl Pts',(-2.78837465172301,-1.61897762728566,
52.1824147314204));
#21470=CARTESIAN_POINT('Ctrl Pts',(-2.83728872571689,-1.53163302452011,
52.1762581543411));
#21471=CARTESIAN_POINT('Ctrl Pts',(-2.88201740350844,-1.44225283788057,
52.1701015772619));
#21472=CARTESIAN_POINT('Ctrl Pts',(-2.92679340522606,-1.35277808503532,
52.1639384863885));
#21473=CARTESIAN_POINT('Ctrl Pts',(-2.96737497435138,-1.26126383629905,
52.1577753955151));
#21474=CARTESIAN_POINT('Ctrl Pts',(-3.00359117726584,-1.1681428004961,52.1516123046418));
#21475=CARTESIAN_POINT('Ctrl Pts',(-3.03982782354858,-1.07496919961244,
52.145445734819));
#21476=CARTESIAN_POINT('Ctrl Pts',(-3.07169405802658,-0.980187416157667,
52.1392791649963));
#21477=CARTESIAN_POINT('Ctrl Pts',(-3.09906875876202,-0.884245662112788,
52.1331125951736));
#21478=CARTESIAN_POINT('Ctrl Pts',(-3.12648788655829,-0.78814820188564,
52.1269360174762));
#21479=CARTESIAN_POINT('Ctrl Pts',(-3.14940082251084,-0.690887433118548,
52.1207594397788));
#21480=CARTESIAN_POINT('Ctrl Pts',(-3.16773749635297,-0.592922184354288,
52.1145828620815));
#21481=CARTESIAN_POINT('Ctrl Pts',(-3.18018914169148,-0.526398203854166,
52.1103886142285));
#21482=CARTESIAN_POINT('Ctrl Pts',(-3.19053166669938,-0.45954954615121,
52.1061943663755));
#21483=CARTESIAN_POINT('Ctrl Pts',(-3.19875681761807,-0.392520552636372,
52.1020001185225));
#21484=CARTESIAN_POINT('Ctrl Pts',(-3.21463548048016,-0.263121007202109,
52.0939031184461));
#21485=CARTESIAN_POINT('Ctrl Pts',(-3.22266431702142,-0.132738974111897,
52.0858061183696));
#21486=CARTESIAN_POINT('Ctrl Pts',(-3.22274931785554,-0.00209684566102432,
52.0777091182931));
#21487=CARTESIAN_POINT('Ctrl Pts',(-0.49058209429631,-3.18519179505032,
51.1068136617517));
#21488=CARTESIAN_POINT('Ctrl Pts',(-0.490290107655991,-3.18523676672761,
51.1068316447501));
#21489=CARTESIAN_POINT('Ctrl Pts',(-0.489998114782029,-3.18528169838757,
51.1068496298593));
#21490=CARTESIAN_POINT('Ctrl Pts',(-0.468096712346372,-3.18864877873823,
51.1081987512924));
#21491=CARTESIAN_POINT('Ctrl Pts',(-0.446454779646167,-3.19175087250692,
51.1095409714125));
#21492=CARTESIAN_POINT('Ctrl Pts',(-0.404815837904996,-3.19728751664578,
51.1121436895462));
#21493=CARTESIAN_POINT('Ctrl Pts',(-0.384824715757757,-3.19975517514846,
51.1134024422831));
#21494=CARTESIAN_POINT('Ctrl Pts',(-0.333899886945455,-3.2055571173243,
51.1166302994167));
#21495=CARTESIAN_POINT('Ctrl Pts',(-0.302939026454846,-3.20863107052092,
51.1186126466662));
#21496=CARTESIAN_POINT('Ctrl Pts',(-0.154965786186221,-3.22116193810289,
51.1281666872916));
#21497=CARTESIAN_POINT('Ctrl Pts',(-0.0375478319452818,-3.22466801702292,
51.1359823598414));
#21498=CARTESIAN_POINT('Ctrl Pts',(0.259554203716849,-3.21731020474563,
51.1559707327345));
#21499=CARTESIAN_POINT('Ctrl Pts',(0.438645180692646,-3.19781966457959,
51.1681998515738));
#21500=CARTESIAN_POINT('Ctrl Pts',(0.727511777596534,-3.1416460708504,51.1876991900715));
#21501=CARTESIAN_POINT('Ctrl Pts',(0.838610496093273,-3.11383214988942,
51.1951478109563));
#21502=CARTESIAN_POINT('Ctrl Pts',(0.988197115764423,-3.06779277200161,
51.2050859567072));
#21503=CARTESIAN_POINT('Ctrl Pts',(1.02814512885269,-3.05463645800857,51.2077314169602));
#21504=CARTESIAN_POINT('Ctrl Pts',(1.10068721352603,-3.02916131506546,51.2125215864282));
#21505=CARTESIAN_POINT('Ctrl Pts',(1.13336040919608,-3.01708882000855,51.214673918202));
#21506=CARTESIAN_POINT('Ctrl Pts',(1.1999816092941,-2.99123777817153,51.2190542336476));
#21507=CARTESIAN_POINT('Ctrl Pts',(1.23390331379865,-2.97740526120672,51.2212800514071));
#21508=CARTESIAN_POINT('Ctrl Pts',(1.32089412138698,-2.94019021743242,51.2269811971863));
#21509=CARTESIAN_POINT('Ctrl Pts',(1.37358228803536,-2.91594789076526,51.2304273539274));
#21510=CARTESIAN_POINT('Ctrl Pts',(1.58200656681976,-2.81314609925882,51.2440732512367));
#21511=CARTESIAN_POINT('Ctrl Pts',(1.73190786415949,-2.72342405145618,51.2538997102635));
#21512=CARTESIAN_POINT('Ctrl Pts',(2.04042777626394,-2.50293940724075,51.2751490872247));
#21513=CARTESIAN_POINT('Ctrl Pts',(2.1952856898368,-2.368280410139,51.2865044750282));
#21514=CARTESIAN_POINT('Ctrl Pts',(2.36051924651906,-2.19437969419563,51.3007821596266));
#21515=CARTESIAN_POINT('Ctrl Pts',(2.38431388412331,-2.16850188626445,51.3028985868121));
#21516=CARTESIAN_POINT('Ctrl Pts',(2.42159804535607,-2.12659796658401,51.3063227184349));
#21517=CARTESIAN_POINT('Ctrl Pts',(2.43536348757143,-2.11081989564496,51.3076113502371));
#21518=CARTESIAN_POINT('Ctrl Pts',(2.46249915356084,-2.07909798131315,51.3102034803851));
#21519=CARTESIAN_POINT('Ctrl Pts',(2.47587064688338,-2.06315655691087,51.311506787569));
#21520=CARTESIAN_POINT('Ctrl Pts',(2.51097698385488,-2.0204701974759,51.3149958302204));
#21521=CARTESIAN_POINT('Ctrl Pts',(2.53243823152593,-1.99350485725825,51.317199033236));
#21522=CARTESIAN_POINT('Ctrl Pts',(2.57993098342679,-1.93182709324429,51.3222268375603));
#21523=CARTESIAN_POINT('Ctrl Pts',(2.60570204253932,-1.89692285624048,51.3250640883028));
#21524=CARTESIAN_POINT('Ctrl Pts',(2.68939254143697,-1.77864818238451,51.3346249068805));
#21525=CARTESIAN_POINT('Ctrl Pts',(2.74407525939569,-1.69306545881416,51.3414551200959));
#21526=CARTESIAN_POINT('Ctrl Pts',(2.91638846445753,-1.39304303545962,51.3648122754991));
#21527=CARTESIAN_POINT('Ctrl Pts',(3.01365172664422,-1.16783184519339,51.3812963766599));
#21528=CARTESIAN_POINT('Ctrl Pts',(3.10003600224227,-0.882476852655956,
51.4003571228152));
#21529=CARTESIAN_POINT('Ctrl Pts',(3.11428020503107,-0.830811627159511,
51.403743220065));
#21530=CARTESIAN_POINT('Ctrl Pts',(3.13502534927322,-0.747511954259369,
51.4091021868561));
#21531=CARTESIAN_POINT('Ctrl Pts',(3.14235038933667,-0.716095114170127,
51.4111008261522));
#21532=CARTESIAN_POINT('Ctrl Pts',(3.15670181977314,-0.650075002280733,
51.415255608819));
#21533=CARTESIAN_POINT('Ctrl Pts',(3.1636337704346,-0.61545544660668,51.4174085180746));
#21534=CARTESIAN_POINT('Ctrl Pts',(3.17911033525125,-0.530974151325396,
51.4226035957965));
#21535=CARTESIAN_POINT('Ctrl Pts',(3.18705271958366,-0.481010864800697,
51.4256266401028));
#21536=CARTESIAN_POINT('Ctrl Pts',(3.21809515478472,-0.250914287982896,
51.4393523052373));
#21537=CARTESIAN_POINT('Ctrl Pts',(3.22712156888969,-0.0692120845311815,
51.4496181978966));
#21538=CARTESIAN_POINT('Ctrl Pts',(3.21351051033534,0.321159625871323,51.4715234059123));
#21539=CARTESIAN_POINT('Ctrl Pts',(3.18593029833733,0.528792442210811,51.4830862323664));
#21540=CARTESIAN_POINT('Ctrl Pts',(3.12998248802018,0.768581636709448,51.497705460616));
#21541=CARTESIAN_POINT('Ctrl Pts',(3.12088027545296,0.804744772095314,51.4999458853901));
#21542=CARTESIAN_POINT('Ctrl Pts',(3.10557133090353,0.861395420711091,51.5035235629975));
#21543=CARTESIAN_POINT('Ctrl Pts',(3.09978416848768,0.881993997396937,51.5048387240409));
#21544=CARTESIAN_POINT('Ctrl Pts',(3.08806406623339,0.922169342552654,51.50743457907));
#21545=CARTESIAN_POINT('Ctrl Pts',(3.08214905722959,0.94175001238857,51.5087143087785));
#21546=CARTESIAN_POINT('Ctrl Pts',(3.0662916496347,0.992493342557641,51.5120663669271));
#21547=CARTESIAN_POINT('Ctrl Pts',(3.05606062919632,1.02356277558895,51.514153918756));
#21548=CARTESIAN_POINT('Ctrl Pts',(2.99048064656726,1.21296090783879,51.5270733460814));
#21549=CARTESIAN_POINT('Ctrl Pts',(2.92331800224965,1.3669129551894,51.5383971390847));
#21550=CARTESIAN_POINT('Ctrl Pts',(2.74161808155065,1.70808059803781,51.5645073229794));
#21551=CARTESIAN_POINT('Ctrl Pts',(2.61932502007288,1.89028368108255,51.5792006897566));
#21552=CARTESIAN_POINT('Ctrl Pts',(2.44336519088943,2.10220883763423,51.5968563902201));
#21553=CARTESIAN_POINT('Ctrl Pts',(2.4061004205941,2.14476032631172,51.6004375258929));
#21554=CARTESIAN_POINT('Ctrl Pts',(2.34305528999035,2.21303699275526,51.6062474625127));
#21555=CARTESIAN_POINT('Ctrl Pts',(2.31792591084968,2.23934375802175,51.6085025191718));
#21556=CARTESIAN_POINT('Ctrl Pts',(2.26744178830494,2.29043263662587,51.6129174383105));
#21557=CARTESIAN_POINT('Ctrl Pts',(2.2421129261613,2.31523297034333,51.6150779515386));
#21558=CARTESIAN_POINT('Ctrl Pts',(2.17902922843028,2.37499392599764,51.6203313436629));
#21559=CARTESIAN_POINT('Ctrl Pts',(2.14083583868097,2.40947854845139,51.623403979037));
#21560=CARTESIAN_POINT('Ctrl Pts',(2.05631498153327,2.48219489121072,51.6299894891352));
#21561=CARTESIAN_POINT('Ctrl Pts',(2.00971132950778,2.52007613681449,51.6334887955878));
#21562=CARTESIAN_POINT('Ctrl Pts',(1.8631835979615,2.63252799328865,51.6441392890125));
#21563=CARTESIAN_POINT('Ctrl Pts',(1.75996882270117,2.7026226154538,51.6511553475141));
#21564=CARTESIAN_POINT('Ctrl Pts',(1.47365435942886,2.87368797625666,51.6698507839225));
#21565=CARTESIAN_POINT('Ctrl Pts',(1.28439195996141,2.96311594629629,51.6814201138146));
#21566=CARTESIAN_POINT('Ctrl Pts',(1.0551891854481,3.04530727265274,51.6959219249024));
#21567=CARTESIAN_POINT('Ctrl Pts',(1.02235465232164,3.0564867656135,51.6980112112522));
#21568=CARTESIAN_POINT('Ctrl Pts',(0.969502823696837,3.07353487511818,51.7014025669018));
#21569=CARTESIAN_POINT('Ctrl Pts',(0.949596993810202,3.0797431466081,51.7026862376561));
#21570=CARTESIAN_POINT('Ctrl Pts',(0.90961467911149,3.09178844680354,51.7052798980192));
#21571=CARTESIAN_POINT('Ctrl Pts',(0.889538842442377,3.09762413076188,51.7065898759589));
#21572=CARTESIAN_POINT('Ctrl Pts',(0.835749975787081,3.11269358323241,51.7101174358386));
#21573=CARTESIAN_POINT('Ctrl Pts',(0.801942000068785,3.12157462909925,51.7123531330496));
#21574=CARTESIAN_POINT('Ctrl Pts',(0.725051079468145,3.14044168467961,51.717469508535));
#21575=CARTESIAN_POINT('Ctrl Pts',(0.681893810142788,3.15009420773003,51.7203634611653));
#21576=CARTESIAN_POINT('Ctrl Pts',(0.535673901478936,3.17965214954521,51.7302143335137));
#21577=CARTESIAN_POINT('Ctrl Pts',(0.431844089580025,3.19540967775533,51.7372837866577));
#21578=CARTESIAN_POINT('Ctrl Pts',(0.0914729767297211,3.23017175029711,
51.7603879707462));
#21579=CARTESIAN_POINT('Ctrl Pts',(-0.146468486493921,3.22815085417305,
51.7763622917443));
#21580=CARTESIAN_POINT('Ctrl Pts',(-0.436209392761729,3.19355806952478,
51.7950334414112));
#21581=CARTESIAN_POINT('Ctrl Pts',(-0.490190750646011,3.18571897372396,
51.7984822437652));
#21582=CARTESIAN_POINT('Ctrl Pts',(-0.579431127491248,3.17043734628283,
51.804137093452));
#21583=CARTESIAN_POINT('Ctrl Pts',(-0.614809173474371,3.16376725511623,
51.8063666532724));
#21584=CARTESIAN_POINT('Ctrl Pts',(-0.685081857004411,3.1492948879866,51.8107732613681));
#21585=CARTESIAN_POINT('Ctrl Pts',(-0.719973131141142,3.1415019163951,51.8129502549527));
#21586=CARTESIAN_POINT('Ctrl Pts',(-0.806417913065924,3.12067853628499,
51.8183207485106));
#21587=CARTESIAN_POINT('Ctrl Pts',(-0.857793158825484,3.10694958964908,
51.8214917587533));
#21588=CARTESIAN_POINT('Ctrl Pts',(-1.09846725678583,3.03620910082595,51.8362843219656));
#21589=CARTESIAN_POINT('Ctrl Pts',(-1.28260132638872,2.9631300959435,51.84738499997));
#21590=CARTESIAN_POINT('Ctrl Pts',(-1.62686334038401,2.78835429070109,51.8690118830049));
#21591=CARTESIAN_POINT('Ctrl Pts',(-1.78701603336566,2.68852411073114,51.8795097837651));
#21592=CARTESIAN_POINT('Ctrl Pts',(-1.96686007627628,2.55321904865113,51.8928804843974));
#21593=CARTESIAN_POINT('Ctrl Pts',(-1.99582374975928,2.53064287779629,51.8950879438696));
#21594=CARTESIAN_POINT('Ctrl Pts',(-2.04094594220585,2.49421525743405,51.8986246515297));
#21595=CARTESIAN_POINT('Ctrl Pts',(-2.05736467762032,2.48068954407287,51.899932620253));
#21596=CARTESIAN_POINT('Ctrl Pts',(-2.08936686590869,2.45378999269332,51.9025264395873));
#21597=CARTESIAN_POINT('Ctrl Pts',(-2.10495861574456,2.44042790951428,51.9038115225685));
#21598=CARTESIAN_POINT('Ctrl Pts',(-2.14536402887971,2.40512532676235,51.9071956129615));
#21599=CARTESIAN_POINT('Ctrl Pts',(-2.16996854438321,2.38295005672354,51.9093103695604));
#21600=CARTESIAN_POINT('Ctrl Pts',(-2.31836503331676,2.24500084198258,51.9223768133586));
#21601=CARTESIAN_POINT('Ctrl Pts',(-2.43319689165671,2.11999730758702,51.9338273301582));
#21602=CARTESIAN_POINT('Ctrl Pts',(-2.67066272947989,1.81665502342507,51.9598499172809));
#21603=CARTESIAN_POINT('Ctrl Pts',(-2.78628762603418,1.63379986941337,51.9743292393177));
#21604=CARTESIAN_POINT('Ctrl Pts',(-2.90817058466921,1.3899238463634,51.9918082234132));
#21605=CARTESIAN_POINT('Ctrl Pts',(-2.93221893885977,1.33844581121686,51.9954061772336));
#21606=CARTESIAN_POINT('Ctrl Pts',(-2.96943423327285,1.25295837911296,52.0012358369022));
#21607=CARTESIAN_POINT('Ctrl Pts',(-2.98340652612153,1.21931539711588,52.0034941545762));
#21608=CARTESIAN_POINT('Ctrl Pts',(-3.00983145913836,1.15251295564747,52.0079104130502));
#21609=CARTESIAN_POINT('Ctrl Pts',(-3.02231377212018,1.11937086890504,52.0100690902119));
#21610=CARTESIAN_POINT('Ctrl Pts',(-3.05151870996004,1.03777540743443,52.0153090801155));
#21611=CARTESIAN_POINT('Ctrl Pts',(-3.06763686240202,0.98911513283617,52.0183704041163));
#21612=CARTESIAN_POINT('Ctrl Pts',(-3.14257448439993,0.743391774206481,
52.0335468520173));
#21613=CARTESIAN_POINT('Ctrl Pts',(-3.1835990865213,0.541399705689971,52.0450832042486));
#21614=CARTESIAN_POINT('Ctrl Pts',(-3.21693512294275,0.224218463995345,
52.0629479811517));
#21615=CARTESIAN_POINT('Ctrl Pts',(-3.22282683556096,0.111039161045053,
52.0692837228589));
#21616=CARTESIAN_POINT('Ctrl Pts',(-3.22274924355897,-0.00220808517695452,
52.0757655954735));
#21617=CARTESIAN_POINT('Origin',(-9.07107736682793E-15,0.,39.1419356690201));
#21618=CARTESIAN_POINT('',(-3.9329991429617,-0.00259643266821552,59.9877721469517));
#21619=CARTESIAN_POINT('',(-1.9005600208235,-3.44330663857395,60.199854037326));
#21620=CARTESIAN_POINT('Ctrl Pts',(-3.93299914296127,-0.00259643332659257,
59.9877721469851));
#21621=CARTESIAN_POINT('Ctrl Pts',(-3.93287035264033,-0.197684139483549,
59.9976703740445));
#21622=CARTESIAN_POINT('Ctrl Pts',(-3.91822346530484,-0.39225107737111,
60.007568601104));
#21623=CARTESIAN_POINT('Ctrl Pts',(-3.88930500305625,-0.584632870442379,
60.0174668281635));
#21624=CARTESIAN_POINT('Ctrl Pts',(-3.87231073497013,-0.697688251404115,
60.0232836355296));
#21625=CARTESIAN_POINT('Ctrl Pts',(-3.85035239201043,-0.810203799500005,
60.0291004428958));
#21626=CARTESIAN_POINT('Ctrl Pts',(-3.82347367061698,-0.921703905871498,
60.0349172502619));
#21627=CARTESIAN_POINT('Ctrl Pts',(-3.79662898496787,-1.03306282289629,
60.0407266919738));
#21628=CARTESIAN_POINT('Ctrl Pts',(-3.76487640454396,-1.14340844800533,
60.0465361336857));
#21629=CARTESIAN_POINT('Ctrl Pts',(-3.72831122421556,-1.25227170190353,
60.0523455753976));
#21630=CARTESIAN_POINT('Ctrl Pts',(-3.69178210763556,-1.36102758543014,
60.0581492873348));
#21631=CARTESIAN_POINT('Ctrl Pts',(-3.65044996275524,-1.46830360724953,
60.063952999272));
#21632=CARTESIAN_POINT('Ctrl Pts',(-3.6044606494612,-1.5736430429058,60.0697567112092));
#21633=CARTESIAN_POINT('Ctrl Pts',(-3.55850265691398,-1.6789107377693,60.0755564705631));
#21634=CARTESIAN_POINT('Ctrl Pts',(-3.50789397143091,-1.78224408377972,
60.081356229917));
#21635=CARTESIAN_POINT('Ctrl Pts',(-3.45282933167017,-1.88320434535348,
60.0871559892709));
#21636=CARTESIAN_POINT('Ctrl Pts',(-3.39778369812136,-1.9841297592984,60.0929537467692));
#21637=CARTESIAN_POINT('Ctrl Pts',(-3.33828536876333,-2.08268334678356,
60.0987515042675));
#21638=CARTESIAN_POINT('Ctrl Pts',(-3.27457566431122,-2.17844972829322,
60.1045492617658));
#21639=CARTESIAN_POINT('Ctrl Pts',(-3.210871814503,-2.27420730929021,60.1103464864755));
#21640=CARTESIAN_POINT('Ctrl Pts',(-3.14295759308554,-2.36717784261953,
60.1161437111852));
#21641=CARTESIAN_POINT('Ctrl Pts',(-3.07111794389987,-2.45697447578446,
60.1219409358949));
#21642=CARTESIAN_POINT('Ctrl Pts',(-2.99926670133485,-2.546785600201,60.1277390961524));
#21643=CARTESIAN_POINT('Ctrl Pts',(-2.92348903631433,-2.63342147777904,
60.1335372564098));
#21644=CARTESIAN_POINT('Ctrl Pts',(-2.84410997024081,-2.71652857102164,
60.1393354166673));
#21645=CARTESIAN_POINT('Ctrl Pts',(-2.76465456865678,-2.79971558486175,
60.1451391527717));
#21646=CARTESIAN_POINT('Ctrl Pts',(-2.68159114425714,-2.87936673488443,
60.1509428888762));
#21647=CARTESIAN_POINT('Ctrl Pts',(-2.59528131529041,-2.95516562894613,
60.1567466249806));
#21648=CARTESIAN_POINT('Ctrl Pts',(-2.50892457566129,-3.03100572082239,
60.162553515501));
#21649=CARTESIAN_POINT('Ctrl Pts',(-2.41931824729355,-3.10298912474427,
60.1683604060214));
#21650=CARTESIAN_POINT('Ctrl Pts',(-2.32685530004097,-3.170841120692,60.1741672965419));
#21651=CARTESIAN_POINT('Ctrl Pts',(-2.23426054396859,-3.23878984177961,
60.1799824649661));
#21652=CARTESIAN_POINT('Ctrl Pts',(-2.13880139026995,-3.30259516485508,
60.1857976333904));
#21653=CARTESIAN_POINT('Ctrl Pts',(-2.04089794694587,-3.36202685446624,
60.1916128018147));
#21654=CARTESIAN_POINT('Ctrl Pts',(-1.99464847917838,-3.39010231248604,
60.1943598803184));
#21655=CARTESIAN_POINT('Ctrl Pts',(-1.94785387496363,-3.41720242601197,
60.1971069588222));
#21656=CARTESIAN_POINT('Ctrl Pts',(-1.9005600208235,-3.44330663857395,60.199854037326));
#21657=CARTESIAN_POINT('',(-3.89175630324296,-0.568086152065691,60.1999356690201));
#21658=CARTESIAN_POINT('Origin',(-1.16499385964724E-14,0.,60.1999356690201));
#21659=CARTESIAN_POINT('',(-3.93059892528386,-0.000146120431290349,60.171099191055));
#21660=CARTESIAN_POINT('Origin',(0.0100450429162835,0.000746738084422618,
60.1858575446646));
#21661=CARTESIAN_POINT('',(-3.92955718600433,-0.000499007535493628,58.9210993909857));
#21662=CARTESIAN_POINT('Ctrl Pts',(-3.93059892528386,-0.000146120431290349,
60.171099191055));
#21663=CARTESIAN_POINT('Ctrl Pts',(-3.92287704520062,1.1109806906551,60.1148744759824));
#21664=CARTESIAN_POINT('Ctrl Pts',(-2.86359348088526,3.52391769303499,59.9928128865155));
#21665=CARTESIAN_POINT('Ctrl Pts',(1.23859575814269,4.47568193655585,59.8049144226543));
#21666=CARTESIAN_POINT('Ctrl Pts',(4.42193931558343,1.40645034585021,59.6074037994715));
#21667=CARTESIAN_POINT('Ctrl Pts',(3.59560445921063,-2.93448714587229,59.4098931762886));
#21668=CARTESIAN_POINT('Ctrl Pts',(-0.494193783132457,-4.61514490705407,
59.2123825531056));
#21669=CARTESIAN_POINT('Ctrl Pts',(-3.4976014503324,-2.5464335831811,59.0494513447149));
#21670=CARTESIAN_POINT('Ctrl Pts',(-3.92754117139867,-0.620745692192471,
58.9523570107183));
#21671=CARTESIAN_POINT('Ctrl Pts',(-3.92679976020224,-0.000501837635528756,
58.921099551116));
#21672=CARTESIAN_POINT('',(-3.93299855748857,0.00336850010244687,57.6710991910917));
#21673=CARTESIAN_POINT('Ctrl Pts',(-3.93299996879044,-0.000495474015325462,
58.921099191055));
#21674=CARTESIAN_POINT('Ctrl Pts',(-3.93301517740518,0.120228276276205,
58.915024855076));
#21675=CARTESIAN_POINT('Ctrl Pts',(-3.92746761809961,0.240871097188488,
58.9089505190969));
#21676=CARTESIAN_POINT('Ctrl Pts',(-3.91640559202178,0.3609102918741,58.9028761831179));
#21677=CARTESIAN_POINT('Ctrl Pts',(-3.90533220422532,0.481072777857684,
58.8967956082369));
#21678=CARTESIAN_POINT('Ctrl Pts',(-3.88873309117169,0.600630037137997,
58.8907150333559));
#21679=CARTESIAN_POINT('Ctrl Pts',(-3.86670805303361,0.719067335237196,
58.8846344584749));
#21680=CARTESIAN_POINT('Ctrl Pts',(-3.84463785679102,0.837747466236466,
58.8785414165446));
#21681=CARTESIAN_POINT('Ctrl Pts',(-3.81711956975119,0.955302685984484,
58.8724483746144));
#21682=CARTESIAN_POINT('Ctrl Pts',(-3.78430378778388,1.07123006014799,58.8663553326841));
#21683=CARTESIAN_POINT('Ctrl Pts',(-3.75145232548691,1.18728348119134,58.8602556658395));
#21684=CARTESIAN_POINT('Ctrl Pts',(-3.71329199556078,1.30170517931389,58.8541559989948));
#21685=CARTESIAN_POINT('Ctrl Pts',(-3.67002215593741,1.41401074074019,58.8480563321502));
#21686=CARTESIAN_POINT('Ctrl Pts',(-3.62665914886438,1.52655811546717,58.8419435316677));
#21687=CARTESIAN_POINT('Ctrl Pts',(-3.57816478743509,1.6369799095776,58.8358307311853));
#21688=CARTESIAN_POINT('Ctrl Pts',(-3.52478565957446,1.74481375913256,58.8297179307028));
#21689=CARTESIAN_POINT('Ctrl Pts',(-3.48881819467131,1.81747343632637,58.8255990560485));
#21690=CARTESIAN_POINT('Ctrl Pts',(-3.4506338904148,1.88895865836186,58.8214801813942));
#21691=CARTESIAN_POINT('Ctrl Pts',(-3.41031921957498,1.95913547785689,58.8173613067399));
#21692=CARTESIAN_POINT('Ctrl Pts',(-3.35279979340985,2.05926107241989,58.8114846543544));
#21693=CARTESIAN_POINT('Ctrl Pts',(-3.29077262038089,2.15701597551455,58.8056080019689));
#21694=CARTESIAN_POINT('Ctrl Pts',(-3.22445836314778,2.25196742079596,58.7997313495834));
#21695=CARTESIAN_POINT('Ctrl Pts',(-3.15822898990627,2.34679732573266,58.7938622194674));
#21696=CARTESIAN_POINT('Ctrl Pts',(-3.08772367999684,2.43883057417248,58.7879930893513));
#21697=CARTESIAN_POINT('Ctrl Pts',(-3.01320858671637,2.52765959198204,58.7821239592353));
#21698=CARTESIAN_POINT('Ctrl Pts',(-2.93876903204692,2.61639856064413,58.7762607788661));
#21699=CARTESIAN_POINT('Ctrl Pts',(-2.86032804329177,2.70193944562605,58.7703975984968));
#21700=CARTESIAN_POINT('Ctrl Pts',(-2.77819421823987,2.7839047910693,58.7645344181275));
#21701=CARTESIAN_POINT('Ctrl Pts',(-2.69374468321311,2.86818109631402,58.7585059291871));
#21702=CARTESIAN_POINT('Ctrl Pts',(-2.6053912299711,2.94867687489402,58.7524774402467));
#21703=CARTESIAN_POINT('Ctrl Pts',(-2.51351297430408,3.02501926076597,58.7464489513062));
#21704=CARTESIAN_POINT('Ctrl Pts',(-2.4242550254769,3.09918441248804,58.7405923908672));
#21705=CARTESIAN_POINT('Ctrl Pts',(-2.33167094470829,3.1694295916815,58.7347358304281));
#21706=CARTESIAN_POINT('Ctrl Pts',(-2.23614404117579,3.23545187371317,58.728879269989));
#21707=CARTESIAN_POINT('Ctrl Pts',(-2.14063102923534,3.30146455473638,58.7230235612152));
#21708=CARTESIAN_POINT('Ctrl Pts',(-2.04217638487188,3.3632553251924,58.7171678524414));
#21709=CARTESIAN_POINT('Ctrl Pts',(-1.94119363630154,3.42056373517326,58.7113121436677));
#21710=CARTESIAN_POINT('Ctrl Pts',(-1.84020122523329,3.47787762868868,58.7054558745925));
#21711=CARTESIAN_POINT('Ctrl Pts',(-1.73668058797224,3.53070810546995,58.6995996055173));
#21712=CARTESIAN_POINT('Ctrl Pts',(-1.63107053890545,3.57884030058827,58.6937433364422));
#21713=CARTESIAN_POINT('Ctrl Pts',(-1.52002420268137,3.62945010495387,58.6875856153684));
#21714=CARTESIAN_POINT('Ctrl Pts',(-1.40666808240071,3.67486484255668,58.6814278942946));
#21715=CARTESIAN_POINT('Ctrl Pts',(-1.29153552513395,3.71489232513097,58.6752701732209));
#21716=CARTESIAN_POINT('Ctrl Pts',(-1.18187620852402,3.75301695719783,58.6694051815899));
#21717=CARTESIAN_POINT('Ctrl Pts',(-1.0706058879835,3.78625469001799,58.6635401899589));
#21718=CARTESIAN_POINT('Ctrl Pts',(-0.958199284731031,3.81449120207938,
58.6576751983279));
#21719=CARTESIAN_POINT('Ctrl Pts',(-0.845715406440705,3.84274712561193,
58.6518061747501));
#21720=CARTESIAN_POINT('Ctrl Pts',(-0.732094093138896,3.8659948998238,58.6459371511722));
#21721=CARTESIAN_POINT('Ctrl Pts',(-0.617818407258544,3.88417165115711,
58.6400681275944));
#21722=CARTESIAN_POINT('Ctrl Pts',(-0.503380588905055,3.90237419136777,
58.634190777142));
#21723=CARTESIAN_POINT('Ctrl Pts',(-0.388286953575217,3.91549130603822,
58.6283134266895));
#21724=CARTESIAN_POINT('Ctrl Pts',(-0.273023805755644,3.92351207484961,
58.6224360762371));
#21725=CARTESIAN_POINT('Ctrl Pts',(-0.256122737773672,3.92468816245015,
58.6215742786771));
#21726=CARTESIAN_POINT('Ctrl Pts',(-0.239218020856951,3.92575476767173,
58.620712481117));
#21727=CARTESIAN_POINT('Ctrl Pts',(-0.222311181945052,3.92671195001393,
58.619850683557));
#21728=CARTESIAN_POINT('Ctrl Pts',(-0.10700287394539,3.93324014117381,58.6139730372979));
#21729=CARTESIAN_POINT('Ctrl Pts',(0.00878214788636485,3.93469566846353,
58.6080953910388));
#21730=CARTESIAN_POINT('Ctrl Pts',(0.12456068974397,3.9310270457694,58.6022177447797));
#21731=CARTESIAN_POINT('Ctrl Pts',(0.240191292869419,3.92736311074348,58.5963476088202));
#21732=CARTESIAN_POINT('Ctrl Pts',(0.355815023882455,3.91858806008751,58.5904774728607));
#21733=CARTESIAN_POINT('Ctrl Pts',(0.470944954097746,3.90470227420861,58.5846073369012));
#21734=CARTESIAN_POINT('Ctrl Pts',(0.585958402026291,3.89083053722289,58.5787431400303));
#21735=CARTESIAN_POINT('Ctrl Pts',(0.700478635806685,3.87185839966145,58.5728789431595));
#21736=CARTESIAN_POINT('Ctrl Pts',(0.814020779895871,3.84783824632711,58.5670147462886));
#21737=CARTESIAN_POINT('Ctrl Pts',(0.930736634853405,3.82314668571657,58.5609866343755));
#21738=CARTESIAN_POINT('Ctrl Pts',(1.0464184703894,3.7931207520833,58.5549585224624));
#21739=CARTESIAN_POINT('Ctrl Pts',(1.16054710083434,3.7578743229045,58.5489304105493));
#21740=CARTESIAN_POINT('Ctrl Pts',(1.2714474159559,3.72362489672985,58.5430728136593));
#21741=CARTESIAN_POINT('Ctrl Pts',(1.38088079823322,3.68444648681156,58.5372152167694));
#21742=CARTESIAN_POINT('Ctrl Pts',(1.48838400030628,3.64049475588583,58.5313576198794));
#21743=CARTESIAN_POINT('Ctrl Pts',(1.59587167488188,3.59654937323975,58.5255008690463));
#21744=CARTESIAN_POINT('Ctrl Pts',(1.7014293419421,3.5478321966265,58.5196441182132));
#21745=CARTESIAN_POINT('Ctrl Pts',(1.80461282742488,3.49454740175227,58.51378736738));
#21746=CARTESIAN_POINT('Ctrl Pts',(1.90780626312105,3.44125746850656,58.5079300517674));
#21747=CARTESIAN_POINT('Ctrl Pts',(2.00862469561104,3.3833992306576,58.5020727361547));
#21748=CARTESIAN_POINT('Ctrl Pts',(2.10664832181308,3.32122294466994,58.4962154205421));
#21749=CARTESIAN_POINT('Ctrl Pts',(2.20967519125197,3.255873106607,58.4900591405281));
#21750=CARTESIAN_POINT('Ctrl Pts',(2.30961398712476,3.18575304982132,58.4839028605141));
#21751=CARTESIAN_POINT('Ctrl Pts',(2.40601279290025,3.11120417851357,58.4777465805001));
#21752=CARTESIAN_POINT('Ctrl Pts',(2.4978668396267,3.04016994262838,58.4718805406927));
#21753=CARTESIAN_POINT('Ctrl Pts',(2.58650678668462,2.96511527905143,58.4660145008853));
#21754=CARTESIAN_POINT('Ctrl Pts',(2.67157741437195,2.88637542932614,58.4601484610779));
#21755=CARTESIAN_POINT('Ctrl Pts',(2.75670652072071,2.80758145279894,58.454278388878));
#21756=CARTESIAN_POINT('Ctrl Pts',(2.83826113280519,2.72509753832912,58.4484083166782));
#21757=CARTESIAN_POINT('Ctrl Pts',(2.91592456261376,2.63929402400447,58.4425382444783));
#21758=CARTESIAN_POINT('Ctrl Pts',(2.99369808532546,2.55336887768372,58.4366598510738));
#21759=CARTESIAN_POINT('Ctrl Pts',(3.06756915737192,2.46411505804202,58.4307814576694));
#21760=CARTESIAN_POINT('Ctrl Pts',(3.13726283111843,2.37193400592906,58.4249030642649));
#21761=CARTESIAN_POINT('Ctrl Pts',(3.14739174133141,2.35853689898954,58.4240487296347));
#21762=CARTESIAN_POINT('Ctrl Pts',(3.15743249326628,2.34507800797624,58.4231943950044));
#21763=CARTESIAN_POINT('Ctrl Pts',(3.16738432269095,2.33155861010859,58.4223400603742));
#21764=CARTESIAN_POINT('Ctrl Pts',(3.23584973491808,2.23854946489792,58.4164625106149));
#21765=CARTESIAN_POINT('Ctrl Pts',(3.30032708879234,2.14236967624017,58.4105849608556));
#21766=CARTESIAN_POINT('Ctrl Pts',(3.36050927456826,2.04339580491412,58.4047074110963));
#21767=CARTESIAN_POINT('Ctrl Pts',(3.42061456906435,1.94454838674922,58.3988373707407));
#21768=CARTESIAN_POINT('Ctrl Pts',(3.47643539673698,1.84291433477424,58.392967330385));
#21769=CARTESIAN_POINT('Ctrl Pts',(3.5277060482717,1.73890167548002,58.3870972900293));
#21770=CARTESIAN_POINT('Ctrl Pts',(3.57892483490984,1.6349942343887,58.3812331877498));
#21771=CARTESIAN_POINT('Ctrl Pts',(3.62560242006638,1.5287133401183,58.3753690854704));
#21772=CARTESIAN_POINT('Ctrl Pts',(3.6675177727531,1.42049371224939,58.3695049831909));
#21773=CARTESIAN_POINT('Ctrl Pts',(3.71060568748356,1.30924669179295,58.3634768354409));
#21774=CARTESIAN_POINT('Ctrl Pts',(3.74866075799241,1.19595124278602,58.3574486876909));
#21775=CARTESIAN_POINT('Ctrl Pts',(3.78149470033579,1.08110444977914,58.3514205399409));
#21776=CARTESIAN_POINT('Ctrl Pts',(3.81339919314155,0.969508691860899,58.3455630344818));
#21777=CARTESIAN_POINT('Ctrl Pts',(3.84037406709065,0.856448664069443,58.3397055290227));
#21778=CARTESIAN_POINT('Ctrl Pts',(3.86229661013189,0.74239739719614,58.3338480235635));
#21779=CARTESIAN_POINT('Ctrl Pts',(3.88421599171271,0.628362577710646,58.327991362818));
#21780=CARTESIAN_POINT('Ctrl Pts',(3.9010844133856,0.51333720836378,58.3221347020726));
#21781=CARTESIAN_POINT('Ctrl Pts',(3.91283021632444,0.397804849415293,58.3162780413271));
#21782=CARTESIAN_POINT('Ctrl Pts',(3.92457715486367,0.28226132063941,58.3104208143516));
#21783=CARTESIAN_POINT('Ctrl Pts',(3.93120044840834,0.166211115206717,58.3045635873761));
#21784=CARTESIAN_POINT('Ctrl Pts',(3.93268034856764,0.0501425566743083,
58.2987063604006));
#21785=CARTESIAN_POINT('Ctrl Pts',(3.9342358410513,-0.0718547072982891,
58.2925499501331));
#21786=CARTESIAN_POINT('Ctrl Pts',(3.930108598929,-0.193871740764238,58.2863935398657));
#21787=CARTESIAN_POINT('Ctrl Pts',(3.92033767649031,-0.315343467175775,
58.2802371295982));
#21788=CARTESIAN_POINT('Ctrl Pts',(3.91102773847,-0.431084253289698,58.2743711739142));
#21789=CARTESIAN_POINT('Ctrl Pts',(3.89659460221075,-0.546329601463841,
58.2685052182301));
#21790=CARTESIAN_POINT('Ctrl Pts',(3.87712498607451,-0.660598851313416,
58.2626392625461));
#21791=CARTESIAN_POINT('Ctrl Pts',(3.85764198086495,-0.774946683059798,
58.2567692728991));
#21792=CARTESIAN_POINT('Ctrl Pts',(3.83311568603728,-0.888316677816104,
58.2508992832521));
#21793=CARTESIAN_POINT('Ctrl Pts',(3.80368326664931,-1.00024127439931,58.245029293605));
#21794=CARTESIAN_POINT('Ctrl Pts',(3.77420911060816,-1.11232458569804,58.239150980017));
#21795=CARTESIAN_POINT('Ctrl Pts',(3.73981506972742,-1.22295801685179,58.233272666429));
#21796=CARTESIAN_POINT('Ctrl Pts',(3.70068716363292,-1.33169197524145,58.227394352841));
#21797=CARTESIAN_POINT('Ctrl Pts',(3.6949962015805,-1.34750679624183,58.2265393809577));
#21798=CARTESIAN_POINT('Ctrl Pts',(3.68920517855682,-1.3632814753923,58.2256844090745));
#21799=CARTESIAN_POINT('Ctrl Pts',(3.68331474828411,-1.37901467181196,58.2248294371912));
#21800=CARTESIAN_POINT('Ctrl Pts',(3.64282202938542,-1.48716974207072,58.2189520845137));
#21801=CARTESIAN_POINT('Ctrl Pts',(3.59749515991606,-1.59371713921449,58.2130747318362));
#21802=CARTESIAN_POINT('Ctrl Pts',(3.5474816969102,-1.69819392593632,58.2071973791587));
#21803=CARTESIAN_POINT('Ctrl Pts',(3.4975321651715,-1.80253716195077,58.2013275393903));
#21804=CARTESIAN_POINT('Ctrl Pts',(3.4429081306282,-1.90481468264517,58.1954576996219));
#21805=CARTESIAN_POINT('Ctrl Pts',(3.38380612520998,-2.0045810302882,58.1895878598536));
#21806=CARTESIAN_POINT('Ctrl Pts',(3.3247639414653,-2.10424639675748,58.1837239614003));
#21807=CARTESIAN_POINT('Ctrl Pts',(3.26125301177638,-2.20140529327224,58.1778600629471));
#21808=CARTESIAN_POINT('Ctrl Pts',(3.19351663681391,-2.29563509521715,58.1719961644938));
#21809=CARTESIAN_POINT('Ctrl Pts',(3.12388208013346,-2.39250550625047,58.1659679415569));
#21810=CARTESIAN_POINT('Ctrl Pts',(3.04978194281888,-2.48627982715329,58.1599397186201));
#21811=CARTESIAN_POINT('Ctrl Pts',(2.97152969563647,-2.57652872445671,58.1539114956832));
#21812=CARTESIAN_POINT('Ctrl Pts',(2.8954962623307,-2.66421864725272,58.148054200805));
#21813=CARTESIAN_POINT('Ctrl Pts',(2.8155433064224,-2.7485800521487,58.1421969059269));
#21814=CARTESIAN_POINT('Ctrl Pts',(2.73199993873066,-2.82925172700762,58.1363396110487));
#21815=CARTESIAN_POINT('Ctrl Pts',(2.64846864993749,-2.90991173816414,58.1304831630322));
#21816=CARTESIAN_POINT('Ctrl Pts',(2.56134827829891,-2.98688279362739,58.1246267150157));
#21817=CARTESIAN_POINT('Ctrl Pts',(2.47100464841073,-3.05984068662611,58.1187702669991));
#21818=CARTESIAN_POINT('Ctrl Pts',(2.38065231330698,-3.13280560960786,58.1129132546745));
#21819=CARTESIAN_POINT('Ctrl Pts',(2.28707642349239,-3.20175634222721,58.1070562423499));
#21820=CARTESIAN_POINT('Ctrl Pts',(2.19067515603937,-3.26640955189514,58.1011992300252));
#21821=CARTESIAN_POINT('Ctrl Pts',(2.0893412712699,-3.33437090833333,58.0950425286905));
#21822=CARTESIAN_POINT('Ctrl Pts',(1.984885638255,-3.39758302382534,58.0888858273558));
#21823=CARTESIAN_POINT('Ctrl Pts',(1.87780296866296,-3.4557698145103,58.082729126021));
#21824=CARTESIAN_POINT('Ctrl Pts',(1.77578098223335,-3.51120672126896,58.076863387873));
#21825=CARTESIAN_POINT('Ctrl Pts',(1.67137499028506,-3.56208229837883,58.0709976497249));
#21826=CARTESIAN_POINT('Ctrl Pts',(1.56503492400638,-3.60820657482915,58.0651319115768));
#21827=CARTESIAN_POINT('Ctrl Pts',(1.45862174356419,-3.65436256404784,58.0592621404377));
#21828=CARTESIAN_POINT('Ctrl Pts',(1.35027222518725,-3.69576060091199,58.0533923692985));
#21829=CARTESIAN_POINT('Ctrl Pts',(1.24045289060374,-3.7322601230612,58.0475225981594));
#21830=CARTESIAN_POINT('Ctrl Pts',(1.13047782222282,-3.76881140485009,58.0416445031513));
#21831=CARTESIAN_POINT('Ctrl Pts',(1.01902917364397,-3.80045019873225,58.0357664081432));
#21832=CARTESIAN_POINT('Ctrl Pts',(0.906585108639878,-3.82708667798267,
58.0298883131351));
#21833=CARTESIAN_POINT('Ctrl Pts',(0.890200836386732,-3.83096789063616,
58.0290318134262));
#21834=CARTESIAN_POINT('Ctrl Pts',(0.873795440348021,-3.83474298618914,
58.0281753137173));
#21835=CARTESIAN_POINT('Ctrl Pts',(0.857370408780441,-3.83841177860683,
58.0273188140084));
#21836=CARTESIAN_POINT('Ctrl Pts',(0.744658315171258,-3.86358781998696,
58.0214413290875));
#21837=CARTESIAN_POINT('Ctrl Pts',(0.63065162914066,-3.88383636445048,58.0155638441665));
#21838=CARTESIAN_POINT('Ctrl Pts',(0.515818730214368,-3.89902808883958,
58.0096863592455));
#21839=CARTESIAN_POINT('Ctrl Pts',(0.401132583598046,-3.91420039875192,
58.0038163855387));
#21840=CARTESIAN_POINT('Ctrl Pts',(0.285622729257893,-3.92432868717897,
57.9979464118318));
#21841=CARTESIAN_POINT('Ctrl Pts',(0.169769661463749,-3.92933420085979,
57.9920764381249));
#21842=CARTESIAN_POINT('Ctrl Pts',(0.0540338247757839,-3.93433464948782,
57.9862124042134));
#21843=CARTESIAN_POINT('Ctrl Pts',(-0.0620441248003556,-3.93422261693617,
57.9803483703019));
#21844=CARTESIAN_POINT('Ctrl Pts',(-0.177977267250961,-3.92897099662773,
57.9744843363903));
#21845=CARTESIAN_POINT('Ctrl Pts',(-0.297155467544944,-3.92357237942683,
57.9684561636584));
#21846=CARTESIAN_POINT('Ctrl Pts',(-0.416180194610486,-3.91274213832423,
57.9624279909266));
#21847=CARTESIAN_POINT('Ctrl Pts',(-0.534520622811124,-3.89650827072003,
57.9563998181947));
#21848=CARTESIAN_POINT('Ctrl Pts',(-0.649509225308236,-3.88073420451702,
57.9505423849524));
#21849=CARTESIAN_POINT('Ctrl Pts',(-0.763851336782283,-3.85985856348936,
57.9446849517101));
#21850=CARTESIAN_POINT('Ctrl Pts',(-0.877064594808982,-3.83395966287239,
57.9388275184679));
#21851=CARTESIAN_POINT('Ctrl Pts',(-0.990261500798051,-3.8080645029816,
57.9329709312481));
#21852=CARTESIAN_POINT('Ctrl Pts',(-1.10232947555789,-3.77714761821882,
57.9271143440284));
#21853=CARTESIAN_POINT('Ctrl Pts',(-1.21279709346778,-3.74133829131718,
57.9212577568086));
#21854=CARTESIAN_POINT('Ctrl Pts',(-1.32327536840394,-3.70552550982001,
57.9154006045925));
#21855=CARTESIAN_POINT('Ctrl Pts',(-1.43215258716842,-3.66481947512755,
57.9095434523764));
#21856=CARTESIAN_POINT('Ctrl Pts',(-1.53897388377433,-3.61939889830626,
57.9036863001603));
#21857=CARTESIAN_POINT('Ctrl Pts',(-1.65125477755385,-3.57165689251232,
57.8975297910491));
#21858=CARTESIAN_POINT('Ctrl Pts',(-1.76126356701952,-3.51870587739157,
57.8913732819378));
#21859=CARTESIAN_POINT('Ctrl Pts',(-1.86849879628884,-3.46080933428399,
57.8852167728266));
#21860=CARTESIAN_POINT('Ctrl Pts',(-1.97067176686375,-3.40564591610858,
57.879350894341));
#21861=CARTESIAN_POINT('Ctrl Pts',(-2.0703267274518,-3.34599349803455,57.8734850158554));
#21862=CARTESIAN_POINT('Ctrl Pts',(-2.16705873116568,-3.28212514320807,
57.8676191373699));
#21863=CARTESIAN_POINT('Ctrl Pts',(-2.26385724369535,-3.21821287521447,
57.8617492257555));
#21864=CARTESIAN_POINT('Ctrl Pts',(-2.35772846466131,-3.15007914011432,
57.8558793141411));
#21865=CARTESIAN_POINT('Ctrl Pts',(-2.44829976530984,-3.07803789112217,
57.8500094025267));
#21866=CARTESIAN_POINT('Ctrl Pts',(-2.53899949121711,-3.00589449149317,
57.8441311676917));
#21867=CARTESIAN_POINT('Ctrl Pts',(-2.62638965040602,-2.92983279183208,
57.8382529328567));
#21868=CARTESIAN_POINT('Ctrl Pts',(-2.71013374720078,-2.85020421589112,
57.8323746980217));
#21869=CARTESIAN_POINT('Ctrl Pts',(-2.72232163654136,-2.83861528832415,
57.8315191956229));
#21870=CARTESIAN_POINT('Ctrl Pts',(-2.73443236750762,-2.8269508679733,57.8306636932242));
#21871=CARTESIAN_POINT('Ctrl Pts',(-2.74646497456436,-2.8152120956495,57.8298081908255));
#21872=CARTESIAN_POINT('Ctrl Pts',(-2.82794572414756,-2.73572109560111,
57.8240150176262));
#21873=CARTESIAN_POINT('Ctrl Pts',(-2.90612486115895,-2.65254083708072,
57.8182218444269));
#21874=CARTESIAN_POINT('Ctrl Pts',(-2.98064291111864,-2.56598067732363,
57.8124286712277));
#21875=CARTESIAN_POINT('Ctrl Pts',(-3.05639009447922,-2.47799275632479,
57.8065399428887));
#21876=CARTESIAN_POINT('Ctrl Pts',(-3.12835396610249,-2.38651268154054,
57.8006512145497));
#21877=CARTESIAN_POINT('Ctrl Pts',(-3.19619303340045,-2.29190730467933,
57.7947624862107));
#21878=CARTESIAN_POINT('Ctrl Pts',(-3.26276773572902,-2.19906515554492,
57.788983510292));
#21879=CARTESIAN_POINT('Ctrl Pts',(-3.3253697733291,-2.10321354037534,57.7832045343732));
#21880=CARTESIAN_POINT('Ctrl Pts',(-3.38371523795364,-2.00473444337159,
57.7774255584545));
#21881=CARTESIAN_POINT('Ctrl Pts',(-3.44202433386364,-1.90631673174185,
57.7716501847683));
#21882=CARTESIAN_POINT('Ctrl Pts',(-3.49608191299239,-1.80527515762795,
57.765874811082));
#21883=CARTESIAN_POINT('Ctrl Pts',(-3.54564713371219,-1.70202097613356,
57.7600994373957));
#21884=CARTESIAN_POINT('Ctrl Pts',(-3.59519422532281,-1.59880456116783,
57.7543261761258));
#21885=CARTESIAN_POINT('Ctrl Pts',(-3.64025204133391,-1.49337753088417,
57.7485529148558));
#21886=CARTESIAN_POINT('Ctrl Pts',(-3.68062591401499,-1.3861752706932,57.7427796535858));
#21887=CARTESIAN_POINT('Ctrl Pts',(-3.72239921064247,-1.27525720619475,
57.7368062817113));
#21888=CARTESIAN_POINT('Ctrl Pts',(-3.75915775084489,-1.16243904347894,
57.7308329098368));
#21889=CARTESIAN_POINT('Ctrl Pts',(-3.79074071049323,-1.04822414864825,
57.7248595379623));
#21890=CARTESIAN_POINT('Ctrl Pts',(-3.82127793970969,-0.937790976386587,
57.7190839479556));
#21891=CARTESIAN_POINT('Ctrl Pts',(-3.84697683654312,-0.826052543186788,
57.7133083579489));
#21892=CARTESIAN_POINT('Ctrl Pts',(-3.86774353520111,-0.713476661082976,
57.7075327679422));
#21893=CARTESIAN_POINT('Ctrl Pts',(-3.88957694992897,-0.595118131265251,
57.7014605051338));
#21894=CARTESIAN_POINT('Ctrl Pts',(-3.90595789921607,-0.475834354316848,
57.6953882423254));
#21895=CARTESIAN_POINT('Ctrl Pts',(-3.91683895899895,-0.356176317668844,
57.6893159795169));
#21896=CARTESIAN_POINT('Ctrl Pts',(-3.92772001878182,-0.236518281020859,
57.6832437167085));
#21897=CARTESIAN_POINT('Ctrl Pts',(-3.93310120987238,-0.116486528897887,
57.6771714539001));
#21898=CARTESIAN_POINT('Ctrl Pts',(-3.93299855748857,0.00336850010244591,
57.6710991910917));
#21899=CARTESIAN_POINT('',(-3.93299907365457,-0.00269937629320533,56.4210991910142));
#21900=CARTESIAN_POINT('Ctrl Pts',(-3.93299855748795,0.00336850082684063,
57.671099191055));
#21901=CARTESIAN_POINT('Ctrl Pts',(-3.9328558021228,0.170046994925479,57.6626546924876));
#21902=CARTESIAN_POINT('Ctrl Pts',(-3.92211403768641,0.336283765188421,
57.6542101939203));
#21903=CARTESIAN_POINT('Ctrl Pts',(-3.90096089477367,0.50099211315819,57.6457656953529));
#21904=CARTESIAN_POINT('Ctrl Pts',(-3.88971518144716,0.588556541356485,
57.6412763194495));
#21905=CARTESIAN_POINT('Ctrl Pts',(-3.87552761345545,0.675689581232063,
57.636786943546));
#21906=CARTESIAN_POINT('Ctrl Pts',(-3.858431409569,0.762230973951766,57.6322975676426));
#21907=CARTESIAN_POINT('Ctrl Pts',(-3.8360492483995,0.875530008787236,57.6264201263294));
#21908=CARTESIAN_POINT('Ctrl Pts',(-3.8086358013275,0.988028091084555,57.6205426850162));
#21909=CARTESIAN_POINT('Ctrl Pts',(-3.77626146368769,1.0992444486407,57.614665243703));
#21910=CARTESIAN_POINT('Ctrl Pts',(-3.74392850205911,1.21031866616882,57.6087953140516));
#21911=CARTESIAN_POINT('Ctrl Pts',(-3.70664737336858,1.32011402420501,57.6029253844003));
#21912=CARTESIAN_POINT('Ctrl Pts',(-3.6645396368435,1.42815904226489,57.5970554547489));
#21913=CARTESIAN_POINT('Ctrl Pts',(-3.6224745120357,1.53609472213322,57.5911914652835));
#21914=CARTESIAN_POINT('Ctrl Pts',(-3.57559264416276,1.64228320328672,57.5853274758181));
#21915=CARTESIAN_POINT('Ctrl Pts',(-3.52406544918945,1.74626793758267,57.5794634863526));
#21916=CARTESIAN_POINT('Ctrl Pts',(-3.47109542180087,1.8531643876321,57.5734352971071));
#21917=CARTESIAN_POINT('Ctrl Pts',(-3.41321619063103,1.95773142287339,57.5674071078616));
#21918=CARTESIAN_POINT('Ctrl Pts',(-3.35066730421711,2.05949450507899,57.561378918616));
#21919=CARTESIAN_POINT('Ctrl Pts',(-3.28989066153756,2.15837425881672,57.5555215305027));
#21920=CARTESIAN_POINT('Ctrl Pts',(-3.22470565853247,2.25460644459599,57.5496641423894));
#21921=CARTESIAN_POINT('Ctrl Pts',(-3.15537835721852,2.34778117012575,57.5438067542762));
#21922=CARTESIAN_POINT('Ctrl Pts',(-3.08606107138802,2.44094243501441,57.5379502123601));
#21923=CARTESIAN_POINT('Ctrl Pts',(-3.01260292340981,2.53104678712965,57.5320936704441));
#21924=CARTESIAN_POINT('Ctrl Pts',(-2.93531221328044,2.61771488336044,57.5262371285281));
#21925=CARTESIAN_POINT('Ctrl Pts',(-2.85801404835942,2.70439133884422,57.5203800217409));
#21926=CARTESIAN_POINT('Ctrl Pts',(-2.77688286100864,2.78763057171334,57.5145229149536));
#21927=CARTESIAN_POINT('Ctrl Pts',(-2.69226551450583,2.86708831384782,57.5086658081663));
#21928=CARTESIAN_POINT('Ctrl Pts',(-2.60332180850111,2.95060861256073,57.5025092361908));
#21929=CARTESIAN_POINT('Ctrl Pts',(-2.51052639543604,3.02995015524354,57.4963526642153));
#21930=CARTESIAN_POINT('Ctrl Pts',(-2.4143225195777,3.10476017937941,57.4901960922397));
#21931=CARTESIAN_POINT('Ctrl Pts',(-2.32266178896912,3.17603736450276,57.4843302590777));
#21932=CARTESIAN_POINT('Ctrl Pts',(-2.22790754001856,3.24320104916634,57.4784644259157));
#21933=CARTESIAN_POINT('Ctrl Pts',(-2.1304728699342,3.30599067610216,57.4725985927537));
#21934=CARTESIAN_POINT('Ctrl Pts',(-2.03297120669935,3.36882347529813,57.4667287264211));
#21935=CARTESIAN_POINT('Ctrl Pts',(-1.93278580784402,3.42727602089232,57.4608588600886));
#21936=CARTESIAN_POINT('Ctrl Pts',(-1.83035416860492,3.48113381206047,57.454988993756));
#21937=CARTESIAN_POINT('Ctrl Pts',(-1.72777727987114,3.5350679743285,57.449110803871));
#21938=CARTESIAN_POINT('Ctrl Pts',(-1.62294816661977,3.58439420652273,57.443232613986));
#21939=CARTESIAN_POINT('Ctrl Pts',(-1.51632405508477,3.62894617760739,57.437354424101));
#21940=CARTESIAN_POINT('Ctrl Pts',(-1.5008002719141,3.63543265734436,57.436498597554));
#21941=CARTESIAN_POINT('Ctrl Pts',(-1.48523846411807,3.6418180214223,57.4356427710069));
#21942=CARTESIAN_POINT('Ctrl Pts',(-1.46964006652609,3.64810184546172,57.4347869444598));
#21943=CARTESIAN_POINT('Ctrl Pts',(-1.36251680246636,3.69125651810747,57.4289094860445));
#21944=CARTESIAN_POINT('Ctrl Pts',(-1.2533155386513,3.72975956588389,57.4230320276292));
#21945=CARTESIAN_POINT('Ctrl Pts',(-1.14247741335656,3.76340728063947,57.4171545692138));
#21946=CARTESIAN_POINT('Ctrl Pts',(-1.03178093991715,3.79701199339361,57.4112846222292));
#21947=CARTESIAN_POINT('Ctrl Pts',(-0.919452156525088,3.82577359489109,
57.4054146752445));
#21948=CARTESIAN_POINT('Ctrl Pts',(-0.80595237216699,3.84953630633592,57.3995447282598));
#21949=CARTESIAN_POINT('Ctrl Pts',(-0.692567441683296,3.87327497157228,
57.3936807212525));
#21950=CARTESIAN_POINT('Ctrl Pts',(-0.578014268759466,3.8920247249762,57.3878167142452));
#21951=CARTESIAN_POINT('Ctrl Pts',(-0.46276889460642,3.90567970399324,57.3819527072379));
#21952=CARTESIAN_POINT('Ctrl Pts',(-0.344296973369605,3.91971698410523,
57.3759245244895));
#21953=CARTESIAN_POINT('Ctrl Pts',(-0.225093942451591,3.92836986148459,
57.3698963417412));
#21954=CARTESIAN_POINT('Ctrl Pts',(-0.105688128444879,3.93157971043521,
57.3638681589928));
#21955=CARTESIAN_POINT('Ctrl Pts',(0.0103349531106322,3.93469862528602,
57.3580107529321));
#21956=CARTESIAN_POINT('Ctrl Pts',(0.126549042989509,3.93267875871053,57.3521533468714));
#21957=CARTESIAN_POINT('Ctrl Pts',(0.242465467586941,3.92551900989256,57.3462959408106));
#21958=CARTESIAN_POINT('Ctrl Pts',(0.358365148542804,3.91836029527028,57.3404393808277));
#21959=CARTESIAN_POINT('Ctrl Pts',(0.473966838107189,3.90606320018148,57.3345828208447));
#21960=CARTESIAN_POINT('Ctrl Pts',(0.588784372830718,3.8886786910608,57.3287262608618));
#21961=CARTESIAN_POINT('Ctrl Pts',(0.703612983784414,3.87129250488944,57.3228691359075));
#21962=CARTESIAN_POINT('Ctrl Pts',(0.817656881652661,3.84881799082884,57.3170120109533));
#21963=CARTESIAN_POINT('Ctrl Pts',(0.930438211397646,3.82135757745479,57.3111548859991));
#21964=CARTESIAN_POINT('Ctrl Pts',(1.04898503590869,3.79249336018926,57.3049983389389));
#21965=CARTESIAN_POINT('Ctrl Pts',(1.16613629525132,3.75812010673744,57.2988417918787));
#21966=CARTESIAN_POINT('Ctrl Pts',(1.28135437336183,3.71841632551635,57.2926852448185));
#21967=CARTESIAN_POINT('Ctrl Pts',(1.39113216272645,3.6805872503977,57.2868193934047));
#21968=CARTESIAN_POINT('Ctrl Pts',(1.49915478884817,3.63791974173285,57.2809535419908));
#21969=CARTESIAN_POINT('Ctrl Pts',(1.60497832242048,3.59061743778982,57.2750876905769));
#21970=CARTESIAN_POINT('Ctrl Pts',(1.71087461733806,3.5432826100862,57.2692178059653));
#21971=CARTESIAN_POINT('Ctrl Pts',(1.81456844114516,3.49130682586045,57.2633479213537));
#21972=CARTESIAN_POINT('Ctrl Pts',(1.91564110956707,3.43493932105599,57.257478036742));
#21973=CARTESIAN_POINT('Ctrl Pts',(2.0168570987733,3.37849188727444,57.2515998286491));
#21974=CARTESIAN_POINT('Ctrl Pts',(2.1154441667018,3.31764052242658,57.2457216205561));
#21975=CARTESIAN_POINT('Ctrl Pts',(2.21101319397238,3.25267730586359,57.2398434124632));
#21976=CARTESIAN_POINT('Ctrl Pts',(2.22492527986198,3.2432205406929,57.2389877154011));
#21977=CARTESIAN_POINT('Ctrl Pts',(2.23877346964332,3.23367670964208,57.2381320183389));
#21978=CARTESIAN_POINT('Ctrl Pts',(2.25255662447517,3.22404678215639,57.2372763212768));
#21979=CARTESIAN_POINT('Ctrl Pts',(2.34722781773659,3.15790251132625,57.231398867027));
#21980=CARTESIAN_POINT('Ctrl Pts',(2.4391383294844,3.08747638841646,57.2255214127772));
#21981=CARTESIAN_POINT('Ctrl Pts',(2.527876527007,3.01302659533682,57.2196439585274));
#21982=CARTESIAN_POINT('Ctrl Pts',(2.61650131605382,2.9386719499815,57.2137740157343));
#21983=CARTESIAN_POINT('Ctrl Pts',(2.70196154059394,2.8603041240086,57.2079040729412));
#21984=CARTESIAN_POINT('Ctrl Pts',(2.78387469118082,2.77822437967181,57.2020341301481));
#21985=CARTESIAN_POINT('Ctrl Pts',(2.86570495101809,2.69622769466661,57.1961701273531));
#21986=CARTESIAN_POINT('Ctrl Pts',(2.94399498712891,2.61052685334184,57.1903061245581));
#21987=CARTESIAN_POINT('Ctrl Pts',(3.01839604878882,2.5214627287858,57.1844421217631));
#21988=CARTESIAN_POINT('Ctrl Pts',(3.09488020627214,2.42990496903508,57.1784139374436));
#21989=CARTESIAN_POINT('Ctrl Pts',(3.16725405893758,2.3347930928646,57.172385753124));
#21990=CARTESIAN_POINT('Ctrl Pts',(3.23517985254074,2.23653757440254,57.1663575688045));
#21991=CARTESIAN_POINT('Ctrl Pts',(3.30118126296445,2.1410657005177,57.1605001669799));
#21992=CARTESIAN_POINT('Ctrl Pts',(3.36298301382916,2.04262627764838,57.1546427651554));
#21993=CARTESIAN_POINT('Ctrl Pts',(3.42031719664761,1.94162799586238,57.1487853633309));
#21994=CARTESIAN_POINT('Ctrl Pts',(3.47764309776422,1.84064430288911,57.1429288075855));
#21995=CARTESIAN_POINT('Ctrl Pts',(3.53050251048839,1.73710284463135,57.1370722518401));
#21996=CARTESIAN_POINT('Ctrl Pts',(3.57867250704671,1.63143865569869,57.1312156960947));
#21997=CARTESIAN_POINT('Ctrl Pts',(3.62684715050414,1.52576427347434,57.1253585753747));
#21998=CARTESIAN_POINT('Ctrl Pts',(3.67033130738617,1.41796712884944,57.1195014546547));
#21999=CARTESIAN_POINT('Ctrl Pts',(3.70894969170015,1.30850341399527,57.1136443339347));
#22000=CARTESIAN_POINT('Ctrl Pts',(3.74954235499959,1.19344361023822,57.107487780948));
#22001=CARTESIAN_POINT('Ctrl Pts',(3.78475840837375,1.0765428071426,57.1013312279613));
#22002=CARTESIAN_POINT('Ctrl Pts',(3.81445363598056,0.958348819039591,57.0951746749745));
#22003=CARTESIAN_POINT('Ctrl Pts',(3.84274668712548,0.845735822948172,57.089308827747));
#22004=CARTESIAN_POINT('Ctrl Pts',(3.86602834745813,0.731949401313737,57.0834429805194));
#22005=CARTESIAN_POINT('Ctrl Pts',(3.88422663529618,0.617472627454558,57.0775771332918));
#22006=CARTESIAN_POINT('Ctrl Pts',(3.90243743583728,0.502917142131395,57.0717072528494));
#22007=CARTESIAN_POINT('Ctrl Pts',(3.91555785758935,0.387670768125196,57.065837372407));
#22008=CARTESIAN_POINT('Ctrl Pts',(3.92356790214797,0.272220346840702,57.0599674919646));
#22009=CARTESIAN_POINT('Ctrl Pts',(3.93158930500471,0.156606216067098,57.0540892879914));
#22010=CARTESIAN_POINT('Ctrl Pts',(3.93448586071822,0.0407878711960379,
57.0482110840183));
#22011=CARTESIAN_POINT('Ctrl Pts',(3.93228960745753,-0.0747492012093419,
57.0423328800452));
#22012=CARTESIAN_POINT('Ctrl Pts',(3.93196988498466,-0.0915686633171382,
57.0414771527281));
#22013=CARTESIAN_POINT('Ctrl Pts',(3.93154232262271,-0.108382176773632,
57.0406214254111));
#22014=CARTESIAN_POINT('Ctrl Pts',(3.9310071101537,-0.125188257919694,57.039765698094));
#22015=CARTESIAN_POINT('Ctrl Pts',(3.92733107263806,-0.240618649326302,
57.033888245862));
#22016=CARTESIAN_POINT('Ctrl Pts',(3.9185604458126,-0.356076202066446,57.02801079363));
#22017=CARTESIAN_POINT('Ctrl Pts',(3.90468657600241,-0.471075092937918,
57.022133341398));
#22018=CARTESIAN_POINT('Ctrl Pts',(3.8908304372731,-0.585927012945289,57.0162634006666));
#22019=CARTESIAN_POINT('Ctrl Pts',(3.87188407528563,-0.700321030955226,
57.0103934599351));
#22020=CARTESIAN_POINT('Ctrl Pts',(3.84789083010248,-0.813772179183578,
57.0045235192037));
#22021=CARTESIAN_POINT('Ctrl Pts',(3.82392186469027,-0.92710852143751,56.9986595185114));
#22022=CARTESIAN_POINT('Ctrl Pts',(3.79491625992438,-1.03950349058538,56.9927955178191));
#22023=CARTESIAN_POINT('Ctrl Pts',(3.76096897627802,-1.1504787522915,56.9869315171268));
#22024=CARTESIAN_POINT('Ctrl Pts',(3.72607121279863,-1.26456117713076,56.9809033320345));
#22025=CARTESIAN_POINT('Ctrl Pts',(3.68595100804219,-1.37714277801046,56.9748751469422));
#22026=CARTESIAN_POINT('Ctrl Pts',(3.64076762548157,-1.48771640350074,56.9688469618499));
#22027=CARTESIAN_POINT('Ctrl Pts',(3.59686434043458,-1.59515735022638,56.962989562217));
#22028=CARTESIAN_POINT('Ctrl Pts',(3.54818108370429,-1.70070216370797,56.9571321625841));
#22029=CARTESIAN_POINT('Ctrl Pts',(3.49491378453669,-1.80390316776022,56.9512747629511));
#22030=CARTESIAN_POINT('Ctrl Pts',(3.44165417989455,-1.90708926430326,56.9454182094267));
#22031=CARTESIAN_POINT('Ctrl Pts',(3.38381203870854,-2.00793185820569,56.9395616559022));
#22032=CARTESIAN_POINT('Ctrl Pts',(3.32162993049593,-2.10600655384391,56.9337051023777));
#22033=CARTESIAN_POINT('Ctrl Pts',(3.25944182393749,-2.20409071017684,56.9278479839056));
#22034=CARTESIAN_POINT('Ctrl Pts',(3.19291313900253,-2.29940608907504,56.9219908654335));
#22035=CARTESIAN_POINT('Ctrl Pts',(3.12233019496086,-2.39155663818268,56.9161337469614));
#22036=CARTESIAN_POINT('Ctrl Pts',(3.04813879009114,-2.48841826375861,56.9099771909572));
#22037=CARTESIAN_POINT('Ctrl Pts',(2.96946792831302,-2.58178249751481,56.903820634953));
#22038=CARTESIAN_POINT('Ctrl Pts',(2.88669764384709,-2.67122925130128,56.8976640789488));
#22039=CARTESIAN_POINT('Ctrl Pts',(2.807835752015,-2.75645235120187,56.8917982340167));
#22040=CARTESIAN_POINT('Ctrl Pts',(2.72525307953862,-2.8381192281285,56.8859323890847));
#22041=CARTESIAN_POINT('Ctrl Pts',(2.63931490051718,-2.91590566649677,56.8800665441526));
#22042=CARTESIAN_POINT('Ctrl Pts',(2.55331763269417,-2.99374558874696,56.8741966660219));
#22043=CARTESIAN_POINT('Ctrl Pts',(2.46396058114437,-3.06769949738339,56.8683267878912));
#22044=CARTESIAN_POINT('Ctrl Pts',(2.37164057700697,-3.137484657093,56.8624569097604));
#22045=CARTESIAN_POINT('Ctrl Pts',(2.27918966256364,-3.20736877256733,56.8565787081082));
#22046=CARTESIAN_POINT('Ctrl Pts',(2.18376775017054,-3.27307211086288,56.850700506456));
#22047=CARTESIAN_POINT('Ctrl Pts',(2.08579896637717,-3.33435626048865,56.8448223048037));
#22048=CARTESIAN_POINT('Ctrl Pts',(2.07153675914799,-3.34327795174564,56.8439665615062));
#22049=CARTESIAN_POINT('Ctrl Pts',(2.05722061393766,-3.35210606738391,56.8431108182086));
#22050=CARTESIAN_POINT('Ctrl Pts',(2.04285187715921,-3.36083995572342,56.8422550749111));
#22051=CARTESIAN_POINT('Ctrl Pts',(1.94416387664794,-3.42082643819612,56.8363776205261));
#22052=CARTESIAN_POINT('Ctrl Pts',(1.84266969904448,-3.47656074588849,56.8305001661411));
#22053=CARTESIAN_POINT('Ctrl Pts',(1.73877152162544,-3.52777020164073,56.8246227117562));
#22054=CARTESIAN_POINT('Ctrl Pts',(1.63500612754906,-3.57891421098305,56.8187527688412));
#22055=CARTESIAN_POINT('Ctrl Pts',(1.52884321051815,-3.6255446882666,56.8128828259262));
#22056=CARTESIAN_POINT('Ctrl Pts',(1.42071263806928,-3.6674329714434,56.8070128830112));
#22057=CARTESIAN_POINT('Ctrl Pts',(1.31269148692994,-3.7092788663234,56.8011488801076));
#22058=CARTESIAN_POINT('Ctrl Pts',(1.20270702352047,-3.7463919645691,56.7952848772041));
#22059=CARTESIAN_POINT('Ctrl Pts',(1.09121176224109,-3.77859046338005,56.7894208743005));
#22060=CARTESIAN_POINT('Ctrl Pts',(0.976594837299304,-3.81169046134503,
56.7833926900267));
#22061=CARTESIAN_POINT('Ctrl Pts',(0.860381661439289,-3.83959639243075,
56.7773645057528));
#22062=CARTESIAN_POINT('Ctrl Pts',(0.74308401614705,-3.86216456730507,56.771336321479));
#22063=CARTESIAN_POINT('Ctrl Pts',(0.629109489314705,-3.88409337113026,
56.7654789195801));
#22064=CARTESIAN_POINT('Ctrl Pts',(0.514111547251461,-3.90098271963304,
56.7596215176812));
#22065=CARTESIAN_POINT('Ctrl Pts',(0.398572190586897,-3.91275212719778,
56.7537641157823));
#22066=CARTESIAN_POINT('Ctrl Pts',(0.283049523391554,-3.92451983469104,
56.7479075599755));
#22067=CARTESIAN_POINT('Ctrl Pts',(0.166986007382457,-3.93116903010421,
56.7420510041686));
#22068=CARTESIAN_POINT('Ctrl Pts',(0.05086962625867,-3.93267101104635,56.7361944483618));
#22069=CARTESIAN_POINT('Ctrl Pts',(-0.0652579562082603,-3.93417313687936,
56.7303373275933));
#22070=CARTESIAN_POINT('Ctrl Pts',(-0.181438001445452,-3.93052705584168,
56.7244802068249));
#22071=CARTESIAN_POINT('Ctrl Pts',(-0.297182362219594,-3.92175619379706,
56.7186230860565));
#22072=CARTESIAN_POINT('Ctrl Pts',(-0.418843892450566,-3.9125369412075,
56.7124665331958));
#22073=CARTESIAN_POINT('Ctrl Pts',(-0.540023505878393,-3.89765509485266,
56.7063099803351));
#22074=CARTESIAN_POINT('Ctrl Pts',(-0.660161724269143,-3.87719944003529,
56.7001534274744));
#22075=CARTESIAN_POINT('Ctrl Pts',(-0.774627148834287,-3.85770967861889,
56.694287580232));
#22076=CARTESIAN_POINT('Ctrl Pts',(-0.888146879067335,-3.83316060599723,
56.6884217329896));
#22077=CARTESIAN_POINT('Ctrl Pts',(-1.00024979820838,-3.80368102516288,
56.6825558857472));
#22078=CARTESIAN_POINT('Ctrl Pts',(-1.11242979638612,-3.77418117493937,
56.6766860053015));
#22079=CARTESIAN_POINT('Ctrl Pts',(-1.22319065087741,-3.73974418817955,
56.6708161248559));
#22080=CARTESIAN_POINT('Ctrl Pts',(-1.33207874584417,-3.70054796143358,
56.6649462444102));
#22081=CARTESIAN_POINT('Ctrl Pts',(-1.44112124456879,-3.66129615427999,
56.6590680404504));
#22082=CARTESIAN_POINT('Ctrl Pts',(-1.54828530500223,-3.61727179706604,
56.6531898364907));
#22083=CARTESIAN_POINT('Ctrl Pts',(-1.65313952220212,-3.56869986411486,
56.6473116325309));
#22084=CARTESIAN_POINT('Ctrl Pts',(-1.66840380674172,-3.56162894388862,
56.6464559055966));
#22085=CARTESIAN_POINT('Ctrl Pts',(-1.68361918720646,-3.55446172620473,
56.6456001786624));
#22086=CARTESIAN_POINT('Ctrl Pts',(-1.6987843822387,-3.54719898267096,56.6447444517282));
#22087=CARTESIAN_POINT('Ctrl Pts',(-1.80294463275982,-3.49731573459276,
56.6388669980155));
#22088=CARTESIAN_POINT('Ctrl Pts',(-1.90507659828325,-3.44275897953083,
56.6329895443029));
#22089=CARTESIAN_POINT('Ctrl Pts',(-2.00473216674064,-3.38371658677783,
56.6271120905902));
#22090=CARTESIAN_POINT('Ctrl Pts',(-2.10426037385781,-3.32474965110553,
56.6212421483532));
#22091=CARTESIAN_POINT('Ctrl Pts',(-2.20131812632969,-3.26130868710462,
56.6153722061163));
#22092=CARTESIAN_POINT('Ctrl Pts',(-2.29547904868907,-3.19362880388902,
56.6095022638793));
#22093=CARTESIAN_POINT('Ctrl Pts',(-2.38954468605381,-3.12601740850412,
56.6036382616587));
#22094=CARTESIAN_POINT('Ctrl Pts',(-2.48071899135305,-3.05417586585131,
56.597774259438));
#22095=CARTESIAN_POINT('Ctrl Pts',(-2.56860246330661,-2.97838385462574,
56.5919102572174));
#22096=CARTESIAN_POINT('Ctrl Pts',(-2.65894652627984,-2.90046979316662,
56.5858820726894));
#22097=CARTESIAN_POINT('Ctrl Pts',(-2.74581237212719,-2.81838100309495,
56.5798538881614));
#22098=CARTESIAN_POINT('Ctrl Pts',(-2.8288000410369,-2.73246762612655,56.5738257036334));
#22099=CARTESIAN_POINT('Ctrl Pts',(-2.90943660249154,-2.64898824427737,
56.567968302425));
#22100=CARTESIAN_POINT('Ctrl Pts',(-2.98641147531313,-2.5618983896874,56.5621109012166));
#22101=CARTESIAN_POINT('Ctrl Pts',(-3.05939390736504,-2.47155779207724,
56.5562535000082));
#22102=CARTESIAN_POINT('Ctrl Pts',(-3.13236579720378,-2.38123024404369,
56.5503969448935));
#22103=CARTESIAN_POINT('Ctrl Pts',(-3.20134613390724,-2.28765320752724,
56.5445403897788));
#22104=CARTESIAN_POINT('Ctrl Pts',(-3.26604426790166,-2.1912197151602,56.538683834664));
#22105=CARTESIAN_POINT('Ctrl Pts',(-3.3307486430911,-2.09477692020289,56.5328267145886));
#22106=CARTESIAN_POINT('Ctrl Pts',(-3.39116976456058,-1.99547746418522,
56.5269695945132));
#22107=CARTESIAN_POINT('Ctrl Pts',(-3.44706055378369,-1.89374299696357,
56.5211124744378));
#22108=CARTESIAN_POINT('Ctrl Pts',(-3.50580864972638,-1.78680755511183,
56.5149559206134));
#22109=CARTESIAN_POINT('Ctrl Pts',(-3.55955070280624,-1.67718198904026,
56.508799366789));
#22110=CARTESIAN_POINT('Ctrl Pts',(-3.60805540492265,-1.56538340192061,
56.5026428129647));
#22111=CARTESIAN_POINT('Ctrl Pts',(-3.65426975598089,-1.45886384963962,
56.4967769664109));
#22112=CARTESIAN_POINT('Ctrl Pts',(-3.6957299657723,-1.35037221803497,56.4909111198572));
#22113=CARTESIAN_POINT('Ctrl Pts',(-3.73228651975144,-1.24037346572788,
56.4850452733035));
#22114=CARTESIAN_POINT('Ctrl Pts',(-3.76886820907414,-1.13029908111604,
56.479175393545));
#22115=CARTESIAN_POINT('Ctrl Pts',(-3.80053941657034,-1.01871590810039,
56.4733055137865));
#22116=CARTESIAN_POINT('Ctrl Pts',(-3.8272013079809,-0.906101069522241,
56.467435634028));
#22117=CARTESIAN_POINT('Ctrl Pts',(-3.85390100609433,-0.793326542508052,
56.461557430749));
#22118=CARTESIAN_POINT('Ctrl Pts',(-3.8755771375722,-0.679517834267319,
56.45567922747));
#22119=CARTESIAN_POINT('Ctrl Pts',(-3.89218243339884,-0.565159185665073,
56.449801024191));
#22120=CARTESIAN_POINT('Ctrl Pts',(-3.89459978447921,-0.548511183387055,
56.4489452923091));
#22121=CARTESIAN_POINT('Ctrl Pts',(-3.89690976096515,-0.531851528853973,
56.4480895604272));
#22122=CARTESIAN_POINT('Ctrl Pts',(-3.89911230905229,-0.515181716869908,
56.4472338285453));
#22123=CARTESIAN_POINT('Ctrl Pts',(-3.9215347511864,-0.345479226930439,
56.4385222827152));
#22124=CARTESIAN_POINT('Ctrl Pts',(-3.93288130956813,-0.17428194010258,
56.4298107368851));
#22125=CARTESIAN_POINT('Ctrl Pts',(-3.93299907365402,-0.00269937709636038,
56.421099191055));
#22126=CARTESIAN_POINT('',(-3.93299991625273,-0.000811637929910356,55.1710991910932));
#22127=CARTESIAN_POINT('Ctrl Pts',(-3.93299907365457,-0.00269937629318175,
56.4210991910142));
#22128=CARTESIAN_POINT('Ctrl Pts',(-3.93307733299134,0.111324703940528,
56.4153099896917));
#22129=CARTESIAN_POINT('Ctrl Pts',(-3.92819278913474,0.22553690514298,56.4095207883691));
#22130=CARTESIAN_POINT('Ctrl Pts',(-3.91832287188957,0.339462621840942,
56.4037315870465));
#22131=CARTESIAN_POINT('Ctrl Pts',(-3.90846364095589,0.453264989409994,
56.3979486537814));
#22132=CARTESIAN_POINT('Ctrl Pts',(-3.8936298028039,0.566781068380818,56.3921657205164));
#22133=CARTESIAN_POINT('Ctrl Pts',(-3.87385082285357,0.679535725533855,
56.3863827872513));
#22134=CARTESIAN_POINT('Ctrl Pts',(-3.85408757408983,0.792200703413459,
56.3806044534348));
#22135=CARTESIAN_POINT('Ctrl Pts',(-3.82938707706054,0.904105046395576,
56.3748261196184));
#22136=CARTESIAN_POINT('Ctrl Pts',(-3.79983058608534,1.01477904838956,56.3690477858019));
#22137=CARTESIAN_POINT('Ctrl Pts',(-3.77028658968899,1.12540626455076,56.3632718946925));
#22138=CARTESIAN_POINT('Ctrl Pts',(-3.73589078724557,1.23480376284223,56.357496003583));
#22139=CARTESIAN_POINT('Ctrl Pts',(-3.69677531831842,1.34251303378098,56.3517201124736));
#22140=CARTESIAN_POINT('Ctrl Pts',(-3.65766632269399,1.45020447968183,56.3459451772287));
#22141=CARTESIAN_POINT('Ctrl Pts',(-3.61383935817217,1.55620785387354,56.3401702419838));
#22142=CARTESIAN_POINT('Ctrl Pts',(-3.56547584208702,1.6600816303706,56.334395306739));
#22143=CARTESIAN_POINT('Ctrl Pts',(-3.5171078883149,1.76396493800482,56.3286198416039));
#22144=CARTESIAN_POINT('Ctrl Pts',(-3.46420273621944,1.86571787446573,56.3228443764688));
#22145=CARTESIAN_POINT('Ctrl Pts',(-3.40698879950162,1.96492145391886,56.3170689113337));
#22146=CARTESIAN_POINT('Ctrl Pts',(-3.34971954438805,2.06422095026187,56.311287862079));
#22147=CARTESIAN_POINT('Ctrl Pts',(-3.28813339752779,2.16096579784075,56.3055068128243));
#22148=CARTESIAN_POINT('Ctrl Pts',(-3.2225033644604,2.2547640821251,56.2997257635696));
#22149=CARTESIAN_POINT('Ctrl Pts',(-3.15684142882249,2.34860796148597,56.2939419041634));
#22150=CARTESIAN_POINT('Ctrl Pts',(-3.08713195244681,2.43950208873545,56.2881580447573));
#22151=CARTESIAN_POINT('Ctrl Pts',(-3.01368847512405,2.52708740943097,56.2823741853511));
#22152=CARTESIAN_POINT('Ctrl Pts',(-2.94012722295438,2.61481318300418,56.2765810508782));
#22153=CARTESIAN_POINT('Ctrl Pts',(-2.86282029676006,2.69921923792204,56.2707879164053));
#22154=CARTESIAN_POINT('Ctrl Pts',(-2.78211857535195,2.77998295546604,56.2649947819324));
#22155=CARTESIAN_POINT('Ctrl Pts',(-2.71120460390429,2.85095140396986,56.2599042564091));
#22156=CARTESIAN_POINT('Ctrl Pts',(-2.63767004399989,2.91910790852508,56.2548137308858));
#22157=CARTESIAN_POINT('Ctrl Pts',(-2.56177270149997,2.98426031469267,56.2497232053624));
#22158=CARTESIAN_POINT('Ctrl Pts',(-2.4741426282765,3.05948442577611,56.2438457515589));
#22159=CARTESIAN_POINT('Ctrl Pts',(-2.38305277740475,3.1309688112403,56.2379682977553));
#22160=CARTESIAN_POINT('Ctrl Pts',(-2.28885567755934,3.19837907185881,56.2320908439518));
#22161=CARTESIAN_POINT('Ctrl Pts',(-2.19477896305574,3.26570318112787,56.2262209016246));
#22162=CARTESIAN_POINT('Ctrl Pts',(-2.09760322962568,3.32896328266626,56.2203509592973));
#22163=CARTESIAN_POINT('Ctrl Pts',(-1.99771547979881,3.3878639083901,56.2144810169701));
#22164=CARTESIAN_POINT('Ctrl Pts',(-1.89792881017084,3.44670493033897,56.2086170146599));
#22165=CARTESIAN_POINT('Ctrl Pts',(-1.79543593648024,3.50119504340813,56.2027530123498));
#22166=CARTESIAN_POINT('Ctrl Pts',(-1.69065382084452,3.55108133644723,56.1968890100396));
#22167=CARTESIAN_POINT('Ctrl Pts',(-1.58293798252598,3.6023643616344,56.1908608255455));
#22168=CARTESIAN_POINT('Ctrl Pts',(-1.472803176436,3.64878169596722,56.1848326410513));
#22169=CARTESIAN_POINT('Ctrl Pts',(-1.36073103707832,3.69010840555285,56.1788044565571));
#22170=CARTESIAN_POINT('Ctrl Pts',(-1.2518339894023,3.73026429701554,56.1729470552616));
#22171=CARTESIAN_POINT('Ctrl Pts',(-1.14110831956745,3.76561398212311,56.1670896539662));
#22172=CARTESIAN_POINT('Ctrl Pts',(-1.02901654604823,3.79599972971008,56.1612322526707));
#22173=CARTESIAN_POINT('Ctrl Pts',(-0.916940964053141,3.82638108811174,
56.1553756974699));
#22174=CARTESIAN_POINT('Ctrl Pts',(-0.803500068803967,3.85179982693971,
56.1495191422691));
#22175=CARTESIAN_POINT('Ctrl Pts',(-0.689170696037995,3.87214833803181,
56.1436625870683));
#22176=CARTESIAN_POINT('Ctrl Pts',(-0.574830294353475,3.89249881206717,
56.137805466908));
#22177=CARTESIAN_POINT('Ctrl Pts',(-0.459601650906687,3.90777801378501,
56.1319483467476));
#22178=CARTESIAN_POINT('Ctrl Pts',(-0.34397023255161,3.91792974402533,56.1260912265873));
#22179=CARTESIAN_POINT('Ctrl Pts',(-0.222427389465489,3.92860046114706,
56.1199346728867));
#22180=CARTESIAN_POINT('Ctrl Pts',(-0.10044000590948,3.93360552608599,56.113778119186));
#22181=CARTESIAN_POINT('Ctrl Pts',(0.0214254481688518,3.93294164082952,
56.1076215654854));
#22182=CARTESIAN_POINT('Ctrl Pts',(0.137536522395278,3.93230910365255,56.1017557188505));
#22183=CARTESIAN_POINT('Ctrl Pts',(0.253536501168739,3.92653082887976,56.0958898722156));
#22184=CARTESIAN_POINT('Ctrl Pts',(0.368939600224272,3.9156573613362,56.0900240255807));
#22185=CARTESIAN_POINT('Ctrl Pts',(0.484422047447499,3.90477641747932,56.0841541457424));
#22186=CARTESIAN_POINT('Ctrl Pts',(0.59930639031804,3.88879336160765,56.078284265904));
#22187=CARTESIAN_POINT('Ctrl Pts',(0.713116136264978,3.86781002328171,56.0724143860656));
#22188=CARTESIAN_POINT('Ctrl Pts',(0.827087264985156,3.84679693047998,56.0665361827091));
#22189=CARTESIAN_POINT('Ctrl Pts',(0.939980356082507,3.82076949932781,56.0606579793525));
#22190=CARTESIAN_POINT('Ctrl Pts',(1.05133318359121,3.78987962039429,56.054779775996));
#22191=CARTESIAN_POINT('Ctrl Pts',(1.06754359533752,3.78538276416253,56.0539240447239));
#22192=CARTESIAN_POINT('Ctrl Pts',(1.08372139884249,3.78078294314022,56.0530683134517));
#22193=CARTESIAN_POINT('Ctrl Pts',(1.09986520438379,3.77608071049677,56.0522125821796));
#22194=CARTESIAN_POINT('Ctrl Pts',(1.21074635684578,3.74378417587136,56.0463351284772));
#22195=CARTESIAN_POINT('Ctrl Pts',(1.32038552345773,3.70654668199652,56.0404576747747));
#22196=CARTESIAN_POINT('Ctrl Pts',(1.42831002183767,3.66448079289796,56.0345802210723));
#22197=CARTESIAN_POINT('Ctrl Pts',(1.53609659102824,3.62246866466065,56.0287102788472));
#22198=CARTESIAN_POINT('Ctrl Pts',(1.6421724691666,3.5756405618185,56.0228403366221));
#22199=CARTESIAN_POINT('Ctrl Pts',(1.74607874615064,3.52415919223876,56.016970394397));
#22200=CARTESIAN_POINT('Ctrl Pts',(1.84987987641872,3.47272991861609,56.0111063921898));
#22201=CARTESIAN_POINT('Ctrl Pts',(1.9515154052644,3.41665692696112,56.0052423899826));
#22202=CARTESIAN_POINT('Ctrl Pts',(2.05054569804127,3.35615126897528,55.9993783877755));
#22203=CARTESIAN_POINT('Ctrl Pts',(2.15234867458703,3.29395155302879,55.993350203243));
#22204=CARTESIAN_POINT('Ctrl Pts',(2.25139795879813,3.22706744470576,55.9873220187106));
#22205=CARTESIAN_POINT('Ctrl Pts',(2.34724201481534,3.15577944791545,55.9812938341781));
#22206=CARTESIAN_POINT('Ctrl Pts',(2.44037073123758,3.08651109770913,55.9754364329872));
#22207=CARTESIAN_POINT('Ctrl Pts',(2.53047304201592,3.01308530289735,55.9695790317962));
#22208=CARTESIAN_POINT('Ctrl Pts',(2.6171641414872,2.93580327278813,55.9637216306052));
#22209=CARTESIAN_POINT('Ctrl Pts',(2.70384271852548,2.8585324059823,55.9578650755093));
#22210=CARTESIAN_POINT('Ctrl Pts',(2.7871107562618,2.77740668596996,55.9520085204134));
#22211=CARTESIAN_POINT('Ctrl Pts',(2.86661760768431,2.69276669827043,55.9461519653175));
#22212=CARTESIAN_POINT('Ctrl Pts',(2.94613212882622,2.60811854567763,55.9402948452624));
#22213=CARTESIAN_POINT('Ctrl Pts',(3.02188445995336,2.51995575214908,55.9344377252072));
#22214=CARTESIAN_POINT('Ctrl Pts',(3.09356229642685,2.42865421954755,55.928580605152));
#22215=CARTESIAN_POINT('Ctrl Pts',(3.16890452190235,2.33268507491432,55.9224240513057));
#22216=CARTESIAN_POINT('Ctrl Pts',(3.23974431383181,2.23324817505333,55.9162674974595));
#22217=CARTESIAN_POINT('Ctrl Pts',(3.30576941926725,2.13081616913271,55.9101109436132));
#22218=CARTESIAN_POINT('Ctrl Pts',(3.36867687452289,2.03322091674044,55.9042450970832));
#22219=CARTESIAN_POINT('Ctrl Pts',(3.42721378332237,1.93290734142136,55.8983792505531));
#22220=CARTESIAN_POINT('Ctrl Pts',(3.48115707180607,1.83030993042558,55.8925134040231));
#22221=CARTESIAN_POINT('Ctrl Pts',(3.53513745029254,1.72764197611729,55.8866435242895));
#22222=CARTESIAN_POINT('Ctrl Pts',(3.58451774412173,1.62268743150759,55.8807736445559));
#22223=CARTESIAN_POINT('Ctrl Pts',(3.62912290984797,1.51590102091677,55.8749037648223));
#22224=CARTESIAN_POINT('Ctrl Pts',(3.67379132592364,1.40896318665845,55.8690255615697));
#22225=CARTESIAN_POINT('Ctrl Pts',(3.71367096145326,1.30018868876741,55.863147358317));
#22226=CARTESIAN_POINT('Ctrl Pts',(3.74863649650455,1.19004765327864,55.8572691550644));
#22227=CARTESIAN_POINT('Ctrl Pts',(3.75372667912401,1.17401363624696,55.8564134230419));
#22228=CARTESIAN_POINT('Ctrl Pts',(3.75871280715739,1.15795067565749,55.8555576910193));
#22229=CARTESIAN_POINT('Ctrl Pts',(3.7635945846407,1.14186023770998,55.8547019589967));
#22230=CARTESIAN_POINT('Ctrl Pts',(3.7971242648828,1.03134572917699,55.8488245053053));
#22231=CARTESIAN_POINT('Ctrl Pts',(3.825837050582,0.919171963622134,55.8429470516138));
#22232=CARTESIAN_POINT('Ctrl Pts',(3.84956897070611,0.805796338895009,55.8370695979224));
#22233=CARTESIAN_POINT('Ctrl Pts',(3.873270561065,0.692565609990109,55.8311996557087));
#22234=CARTESIAN_POINT('Ctrl Pts',(3.89200386175915,0.578136476797947,55.8253297134951));
#22235=CARTESIAN_POINT('Ctrl Pts',(3.90565442457242,0.462982198165142,55.8194597712814));
#22236=CARTESIAN_POINT('Ctrl Pts',(3.9192911738607,0.347944448537503,55.8135957690861));
#22237=CARTESIAN_POINT('Ctrl Pts',(3.92785536810784,0.232183420396551,55.8077317668907));
#22238=CARTESIAN_POINT('Ctrl Pts',(3.9312835809627,0.116182640927894,55.8018677646954));
#22239=CARTESIAN_POINT('Ctrl Pts',(3.93480777809496,-0.00306596808511381,
55.7958395801587));
#22240=CARTESIAN_POINT('Ctrl Pts',(3.93290404981569,-0.122567518241643,
55.7898113956219));
#22241=CARTESIAN_POINT('Ctrl Pts',(3.92556063774814,-0.241790569217127,
55.7837832110852));
#22242=CARTESIAN_POINT('Ctrl Pts',(3.91842527050216,-0.357635934432931,
55.7779258099071));
#22243=CARTESIAN_POINT('Ctrl Pts',(3.90615432996575,-0.473217930074345,
55.7720684087289));
#22244=CARTESIAN_POINT('Ctrl Pts',(3.88878985773621,-0.588049693791152,
55.7662110075508));
#22245=CARTESIAN_POINT('Ctrl Pts',(3.87142789378636,-0.70286487018093,55.760354452468));
#22246=CARTESIAN_POINT('Ctrl Pts',(3.84897392287386,-0.81692962238403,55.7544978973853));
#22247=CARTESIAN_POINT('Ctrl Pts',(3.82152162899223,-0.929764184696576,
55.7486413423026));
#22248=CARTESIAN_POINT('Ctrl Pts',(3.79406668689527,-1.04260963171762,55.7427842222609));
#22249=CARTESIAN_POINT('Ctrl Pts',(3.76161256084109,-1.15422425211548,55.7369271022192));
#22250=CARTESIAN_POINT('Ctrl Pts',(3.72430346262254,-1.26414109904617,55.7310699821776));
#22251=CARTESIAN_POINT('Ctrl Pts',(3.6850870096299,-1.37967723008603,55.7249134283139));
#22252=CARTESIAN_POINT('Ctrl Pts',(3.64050621031212,-1.49333692218658,55.7187568744503));
#22253=CARTESIAN_POINT('Ctrl Pts',(3.59078633611034,-1.60460041393589,55.7126003205866));
#22254=CARTESIAN_POINT('Ctrl Pts',(3.54341419297414,-1.71061013623707,55.7067344740708));
#22255=CARTESIAN_POINT('Ctrl Pts',(3.49137745245901,-1.81444443054335,55.700868627555));
#22256=CARTESIAN_POINT('Ctrl Pts',(3.43491814617481,-1.91567907778911,55.6950027810391));
#22257=CARTESIAN_POINT('Ctrl Pts',(3.37842001994147,-2.01698333134276,55.6891329013199));
#22258=CARTESIAN_POINT('Ctrl Pts',(3.31749348899304,-2.11568402856839,55.6832630216008));
#22259=CARTESIAN_POINT('Ctrl Pts',(3.25242377604221,-2.21138612210425,55.6773931418816));
#22260=CARTESIAN_POINT('Ctrl Pts',(3.18726179391393,-2.30722392168598,55.6715149386437));
#22261=CARTESIAN_POINT('Ctrl Pts',(3.1179451524688,-2.40005430407117,55.6656367354058));
#22262=CARTESIAN_POINT('Ctrl Pts',(3.04479914065971,-2.48951545346435,55.6597585321679));
#22263=CARTESIAN_POINT('Ctrl Pts',(3.03415075218513,-2.50253895329107,55.6589028000499));
#22264=CARTESIAN_POINT('Ctrl Pts',(3.02342127162262,-2.51549111473446,55.6580470679318));
#22265=CARTESIAN_POINT('Ctrl Pts',(3.0126117652989,-2.5283708888497,55.6571913358138));
#22266=CARTESIAN_POINT('Ctrl Pts',(2.93836846900302,-2.61683347513477,55.6513138820907));
#22267=CARTESIAN_POINT('Ctrl Pts',(2.86010374146197,-2.7021681710333,55.6454364283676));
#22268=CARTESIAN_POINT('Ctrl Pts',(2.77811109404059,-2.78398774228058,55.6395589746444));
#22269=CARTESIAN_POINT('Ctrl Pts',(2.6962232344979,-2.86570274684322,55.6336890323986));
#22270=CARTESIAN_POINT('Ctrl Pts',(2.61061721958203,-2.94391127222344,55.6278190901527));
#22271=CARTESIAN_POINT('Ctrl Pts',(2.52162690192179,-3.01825889669926,55.6219491479068));
#22272=CARTESIAN_POINT('Ctrl Pts',(2.4327266369501,-3.09253128598494,55.6160851456789));
#22273=CARTESIAN_POINT('Ctrl Pts',(2.34044919628267,-3.16295028308159,55.610221143451));
#22274=CARTESIAN_POINT('Ctrl Pts',(2.24516490864606,-3.22919858989568,55.604357141223));
#22275=CARTESIAN_POINT('Ctrl Pts',(2.14721281963813,-3.29730173897339,55.5983289566983));
#22276=CARTESIAN_POINT('Ctrl Pts',(2.04608333297791,-3.36099688426316,55.5923007721737));
#22277=CARTESIAN_POINT('Ctrl Pts',(1.94221513615544,-3.41998382523787,55.586272587649));
#22278=CARTESIAN_POINT('Ctrl Pts',(1.84128960883708,-3.47729961876171,55.5804151864373));
#22279=CARTESIAN_POINT('Ctrl Pts',(1.73777885005964,-3.5301701838976,55.5745577852256));
#22280=CARTESIAN_POINT('Ctrl Pts',(1.63211360431378,-3.5783647358275,55.5687003840139));
#22281=CARTESIAN_POINT('Ctrl Pts',(1.52646362179604,-3.62655232610758,55.5628438288974));
#22282=CARTESIAN_POINT('Ctrl Pts',(1.41866014637608,-3.67006507518796,55.5569872737808));
#22283=CARTESIAN_POINT('Ctrl Pts',(1.3091561935006,-3.70871932896236,55.5511307186643));
#22284=CARTESIAN_POINT('Ctrl Pts',(1.19964167720273,-3.74737731156297,55.5452735985885));
#22285=CARTESIAN_POINT('Ctrl Pts',(1.08842674634867,-3.78117572985175,55.5394164785128));
#22286=CARTESIAN_POINT('Ctrl Pts',(0.975981285700459,-3.80998025322474,
55.533559358437));
#22287=CARTESIAN_POINT('Ctrl Pts',(0.857787272085699,-3.84025735118928,
55.5274028046198));
#22288=CARTESIAN_POINT('Ctrl Pts',(0.738234074887739,-3.86501631056285,
55.5212462508027));
#22289=CARTESIAN_POINT('Ctrl Pts',(0.617880100977389,-3.88416183761904,
55.5150896969855));
#22290=CARTESIAN_POINT('Ctrl Pts',(0.503209139976766,-3.90240332907185,
55.5092238504353));
#22291=CARTESIAN_POINT('Ctrl Pts',(0.387811723368453,-3.91554940901367,
55.5033580038851));
#22292=CARTESIAN_POINT('Ctrl Pts',(0.272175392775181,-3.92357102083901,
55.4974921573349));
#22293=CARTESIAN_POINT('Ctrl Pts',(0.156459553650134,-3.93159814811589,
55.4916222775812));
#22294=CARTESIAN_POINT('Ctrl Pts',(0.0405048846693676,-3.93449378099791,
55.4857523978276));
#22295=CARTESIAN_POINT('Ctrl Pts',(-0.0752019080726868,-3.93228097584878,
55.4798825180739));
#22296=CARTESIAN_POINT('Ctrl Pts',(-0.191072773621905,-3.93006503293095,
55.4740043148016));
#22297=CARTESIAN_POINT('Ctrl Pts',(-0.306694651742633,-3.92272622381837,
55.4681261115293));
#22298=CARTESIAN_POINT('Ctrl Pts',(-0.421586779503249,-3.91033931869705,
55.4622479082569));
#22299=CARTESIAN_POINT('Ctrl Pts',(-0.438312444028915,-3.90853606878246,
55.4613921763816));
#22300=CARTESIAN_POINT('Ctrl Pts',(-0.455022663217249,-3.90662592396641,
55.4605364445063));
#22301=CARTESIAN_POINT('Ctrl Pts',(-0.471715975930993,-3.90460920426763,
55.459680712631));
#22302=CARTESIAN_POINT('Ctrl Pts',(-0.586371250022407,-3.89075769655348,
55.4538032589228));
#22303=CARTESIAN_POINT('Ctrl Pts',(-0.700603844411803,-3.87182908837603,
55.4479258052146));
#22304=CARTESIAN_POINT('Ctrl Pts',(-0.81392906842518,-3.8478576469995,55.4420483515063));
#22305=CARTESIAN_POINT('Ctrl Pts',(-0.927109461036369,-3.82391684149859,
55.4361784092755));
#22306=CARTESIAN_POINT('Ctrl Pts',(-1.03938438951155,-3.79494610458086,
55.4303084670447));
#22307=CARTESIAN_POINT('Ctrl Pts',(-1.15027460512398,-3.76103141874764,
55.4244385248139));
#22308=CARTESIAN_POINT('Ctrl Pts',(-1.26105260670441,-3.72715105247652,
55.4185745226012));
#22309=CARTESIAN_POINT('Ctrl Pts',(-1.37044829054053,-3.68833680898498,
55.4127105203885));
#22310=CARTESIAN_POINT('Ctrl Pts',(-1.47799357236597,-3.64472550407365,
55.4068465181757));
#22311=CARTESIAN_POINT('Ctrl Pts',(-1.58854994337173,-3.59989315509483,
55.4008183336454));
#22312=CARTESIAN_POINT('Ctrl Pts',(-1.69715032901682,-3.54999124256197,
55.3947901491151));
#22313=CARTESIAN_POINT('Ctrl Pts',(-1.80330361743498,-3.49522317790237,
55.3887619645848));
#22314=CARTESIAN_POINT('Ctrl Pts',(-1.90644949749864,-3.44200673672681,
55.3829045633885));
#22315=CARTESIAN_POINT('Ctrl Pts',(-2.0072846847053,-3.38419636745221,55.3770471621923));
#22316=CARTESIAN_POINT('Ctrl Pts',(-2.1053805464764,-3.32202675403417,55.371189760996));
#22317=CARTESIAN_POINT('Ctrl Pts',(-2.20346223840749,-3.25986612094882,
55.365333205895));
#22318=CARTESIAN_POINT('Ctrl Pts',(-2.29880504341771,-3.19334771663263,
55.3594766507939));
#22319=CARTESIAN_POINT('Ctrl Pts',(-2.39100763586765,-3.12275062808778,
55.3536200956929));
#22320=CARTESIAN_POINT('Ctrl Pts',(-2.48321912274417,-3.05214672931554,
55.3477629756327));
#22321=CARTESIAN_POINT('Ctrl Pts',(-2.57228946734184,-2.97746361494556,
55.3419058555725));
#22322=CARTESIAN_POINT('Ctrl Pts',(-2.65784943873237,-2.89902144887375,
55.3360487355123));
#22323=CARTESIAN_POINT('Ctrl Pts',(-2.74778349589481,-2.81656908087041,
55.3298921816736));
#22324=CARTESIAN_POINT('Ctrl Pts',(-2.83383838568118,-2.72996348587167,
55.3237356278349));
#22325=CARTESIAN_POINT('Ctrl Pts',(-2.91562920875397,-2.63962029789528,
55.3175790739962));
#22326=CARTESIAN_POINT('Ctrl Pts',(-2.99355793782203,-2.55354303941493,
55.3117132274616));
#22327=CARTESIAN_POINT('Ctrl Pts',(-3.06761586698334,-2.46407345665159,
55.3058473809269));
#22328=CARTESIAN_POINT('Ctrl Pts',(-3.13751229148755,-2.37160401854201,
55.2999815343923));
#22329=CARTESIAN_POINT('Ctrl Pts',(-3.20745677495527,-2.27907100085189,
55.2941116546541));
#22330=CARTESIAN_POINT('Ctrl Pts',(-3.27323382289168,-2.18353435947397,
55.2882417749159));
#22331=CARTESIAN_POINT('Ctrl Pts',(-3.33459683463049,-2.0854143354433,55.2823718951778));
#22332=CARTESIAN_POINT('Ctrl Pts',(-3.39604685942572,-1.9871551767296,55.2764936919209));
#22333=CARTESIAN_POINT('Ctrl Pts',(-3.45307015651262,-1.88630568322637,
55.270615488664));
#22334=CARTESIAN_POINT('Ctrl Pts',(-3.50546668555464,-1.78330937205708,
55.2647372854072));
#22335=CARTESIAN_POINT('Ctrl Pts',(-3.51309442211228,-1.76831546420914,
55.2638815534208));
#22336=CARTESIAN_POINT('Ctrl Pts',(-3.52062418949426,-1.75327609071389,
55.2630258214344));
#22337=CARTESIAN_POINT('Ctrl Pts',(-3.52805545744261,-1.73819265020005,
55.2621700894481));
#22338=CARTESIAN_POINT('Ctrl Pts',(-3.58270597932811,-1.62726704482021,
55.2558769238707));
#22339=CARTESIAN_POINT('Ctrl Pts',(-3.63218448513408,-1.51363371506473,
55.2495837582933));
#22340=CARTESIAN_POINT('Ctrl Pts',(-3.67623402409242,-1.39778124186345,
55.2432905927159));
#22341=CARTESIAN_POINT('Ctrl Pts',(-3.72014805511793,-1.28228516124943,
55.2370167865661));
#22342=CARTESIAN_POINT('Ctrl Pts',(-3.75866630602752,-1.16458384905882,
55.2307429804162));
#22343=CARTESIAN_POINT('Ctrl Pts',(-3.79157931829358,-1.0451867168542,55.2244691742664));
#22344=CARTESIAN_POINT('Ctrl Pts',(-3.82443080129216,-0.926012791751532,
55.2182070966905));
#22345=CARTESIAN_POINT('Ctrl Pts',(-3.85169783684823,-0.805149670778713,
55.2119450191145));
#22346=CARTESIAN_POINT('Ctrl Pts',(-3.87321950393292,-0.683124933195756,
55.2056829415386));
#22347=CARTESIAN_POINT('Ctrl Pts',(-3.89468073070556,-0.561442883434727,
55.1994384500503));
#22348=CARTESIAN_POINT('Ctrl Pts',(-3.9104287024252,-0.438606036713807,
55.193193958562));
#22349=CARTESIAN_POINT('Ctrl Pts',(-3.9203529112033,-0.315154012539693,
55.1869494670736));
#22350=CARTESIAN_POINT('Ctrl Pts',(-3.92874972239361,-0.21070202435307,
55.1816660417468));
#22351=CARTESIAN_POINT('Ctrl Pts',(-3.93297824814287,-0.105810025913677,
55.17638261642));
#22352=CARTESIAN_POINT('Ctrl Pts',(-3.93299991625273,-0.000811637929901232,
55.1710991910931));
#22353=CARTESIAN_POINT('',(-3.93299849539527,0.00344023525537216,53.9210991911024));
#22354=CARTESIAN_POINT('Ctrl Pts',(-3.93299991625288,-0.000811637171698235,
55.171099191055));
#22355=CARTESIAN_POINT('Ctrl Pts',(-3.93302469910098,0.119280126577695,
55.1650562805083));
#22356=CARTESIAN_POINT('Ctrl Pts',(-3.92754474829664,0.239305970276732,
55.1590133699616));
#22357=CARTESIAN_POINT('Ctrl Pts',(-3.91660425106563,0.358748018161383,
55.1529704594149));
#22358=CARTESIAN_POINT('Ctrl Pts',(-3.90565438845343,0.478292311884077,
55.1469223759625));
#22359=CARTESIAN_POINT('Ctrl Pts',(-3.88923469700456,0.597251441927818,
55.1408742925101));
#22360=CARTESIAN_POINT('Ctrl Pts',(-3.86744093349248,0.715115113773244,
55.1348262090577));
#22361=CARTESIAN_POINT('Ctrl Pts',(-3.84560602894256,0.833201282012232,
55.1287667083743));
#22362=CARTESIAN_POINT('Ctrl Pts',(-3.81837684731064,0.950187491230551,
55.122707207691));
#22363=CARTESIAN_POINT('Ctrl Pts',(-3.78590002041667,1.06557497878337,55.1166477070077));
#22364=CARTESIAN_POINT('Ctrl Pts',(-3.75339153151481,1.18107495883897,55.110582298852));
#22365=CARTESIAN_POINT('Ctrl Pts',(-3.71562531250432,1.29497275462065,55.1045168906962));
#22366=CARTESIAN_POINT('Ctrl Pts',(-3.67279687090257,1.40678788205201,55.0984514825405));
#22367=CARTESIAN_POINT('Ctrl Pts',(-3.62987684703792,1.5188421095303,55.0923731044101));
#22368=CARTESIAN_POINT('Ctrl Pts',(-3.58187311003354,1.62880442247361,55.0862947262797));
#22369=CARTESIAN_POINT('Ctrl Pts',(-3.52902855380103,1.73621613471858,55.0802163481492));
#22370=CARTESIAN_POINT('Ctrl Pts',(-3.48394544654873,1.82785194526426,55.0750307208546));
#22371=CARTESIAN_POINT('Ctrl Pts',(-3.43533991392117,1.91763167699019,55.0698450935599));
#22372=CARTESIAN_POINT('Ctrl Pts',(-3.38338756700251,2.00528740370375,55.0646594662652));
#22373=CARTESIAN_POINT('Ctrl Pts',(-3.32450413844372,2.10463748176254,55.0587820125514));
#22374=CARTESIAN_POINT('Ctrl Pts',(-3.26114449866947,2.20155463144174,55.0529045588376));
#22375=CARTESIAN_POINT('Ctrl Pts',(-3.19353534138345,2.29560907458891,55.0470271051238));
#22376=CARTESIAN_POINT('Ctrl Pts',(-3.12601258965375,2.38954331469244,55.0411571628874));
#22377=CARTESIAN_POINT('Ctrl Pts',(-3.0542513598767,2.48062179232339,55.035287220651));
#22378=CARTESIAN_POINT('Ctrl Pts',(-2.97852348231728,2.56844055124595,55.0294172784146));
#22379=CARTESIAN_POINT('Ctrl Pts',(-2.90287223668011,2.6561704430231,55.0235532761962));
#22380=CARTESIAN_POINT('Ctrl Pts',(-2.82326259561433,2.74064686703493,55.0176892739778));
#22381=CARTESIAN_POINT('Ctrl Pts',(-2.74000841260159,2.82149657077101,55.0118252717594));
#22382=CARTESIAN_POINT('Ctrl Pts',(-2.65442325092256,2.90460993175246,55.0057970872312));
#22383=CARTESIAN_POINT('Ctrl Pts',(-2.56498670439147,2.98389012328394,54.999768902703));
#22384=CARTESIAN_POINT('Ctrl Pts',(-2.47208285490105,3.0589696563556,54.9937407181748));
#22385=CARTESIAN_POINT('Ctrl Pts',(-2.38181104634603,3.13192212574219,54.9878833169729));
#22386=CARTESIAN_POINT('Ctrl Pts',(-2.28826610221537,3.20090848110424,54.982025915771));
#22387=CARTESIAN_POINT('Ctrl Pts',(-2.19183554554886,3.26563101731788,54.9761685145691));
#22388=CARTESIAN_POINT('Ctrl Pts',(-2.09541891817104,3.33034420443178,54.9703119594624));
#22389=CARTESIAN_POINT('Ctrl Pts',(-1.996117849541,3.39079456731503,54.9644554043558));
#22390=CARTESIAN_POINT('Ctrl Pts',(-1.8943494954736,3.44672728671692,54.9585988492491));
#22391=CARTESIAN_POINT('Ctrl Pts',(-1.79257132420814,3.50266540173112,54.9527417291833));
#22392=CARTESIAN_POINT('Ctrl Pts',(-1.68832575587778,3.55408480824334,54.9468846091175));
#22393=CARTESIAN_POINT('Ctrl Pts',(-1.58205460549139,3.60077661418249,54.9410274890516));
#22394=CARTESIAN_POINT('Ctrl Pts',(-1.47035055116756,3.64985544703733,54.9348709352209));
#22395=CARTESIAN_POINT('Ctrl Pts',(-1.35640879189321,3.6937103053147,54.9287143813901));
#22396=CARTESIAN_POINT('Ctrl Pts',(-1.24076483118586,3.73215643210361,54.9225578275593));
#22397=CARTESIAN_POINT('Ctrl Pts',(-1.13058148097809,3.7687871651415,54.9166919810191));
#22398=CARTESIAN_POINT('Ctrl Pts',(-1.01885343043069,3.80050822844357,54.9108261344789));
#22399=CARTESIAN_POINT('Ctrl Pts',(-0.906057021613535,3.82721173618404,
54.9049602879387));
#22400=CARTESIAN_POINT('Ctrl Pts',(-0.793183056920543,3.85393360456162,
54.8990904081951));
#22401=CARTESIAN_POINT('Ctrl Pts',(-0.679239675345709,3.87563097079524,
54.8932205284514));
#22402=CARTESIAN_POINT('Ctrl Pts',(-0.564710861801534,3.89224750530633,
54.8873506487078));
#22403=CARTESIAN_POINT('Ctrl Pts',(-0.450019645830238,3.90888760214599,
54.8814724454454));
#22404=CARTESIAN_POINT('Ctrl Pts',(-0.334741750038798,3.92043245027605,
54.8755942421831));
#22405=CARTESIAN_POINT('Ctrl Pts',(-0.21936369756515,3.92687771240595,54.8697160389208));
#22406=CARTESIAN_POINT('Ctrl Pts',(-0.202567292102037,3.92781599515322,
54.8688603069746));
#22407=CARTESIAN_POINT('Ctrl Pts',(-0.185768758550378,3.92864629385762,
54.8680045750285));
#22408=CARTESIAN_POINT('Ctrl Pts',(-0.168969590628545,3.92936868688124,
54.8671488430823));
#22409=CARTESIAN_POINT('Ctrl Pts',(-0.0535872770041763,3.93433032419565,
54.8612713893744));
#22410=CARTESIAN_POINT('Ctrl Pts',(0.0622028962169044,3.93421364901562,
54.8553939356666));
#22411=CARTESIAN_POINT('Ctrl Pts',(0.177917111223361,3.92897372115594,54.8495164819587));
#22412=CARTESIAN_POINT('Ctrl Pts',(0.293483441659719,3.92374049000572,54.8436465397283));
#22413=CARTESIAN_POINT('Ctrl Pts',(0.40897359852132,3.91339704624324,54.8377765974978));
#22414=CARTESIAN_POINT('Ctrl Pts',(0.523900730986083,3.89795036193026,54.8319066552674));
#22415=CARTESIAN_POINT('Ctrl Pts',(0.638711564309674,3.88251930870526,54.826042653055));
#22416=CARTESIAN_POINT('Ctrl Pts',(0.752960100088524,3.86199534194862,54.8201786508426));
#22417=CARTESIAN_POINT('Ctrl Pts',(0.866162244258594,3.83643740553927,54.8143146486302));
#22418=CARTESIAN_POINT('Ctrl Pts',(0.982533860363644,3.81016388937868,54.8082864640998));
#22419=CARTESIAN_POINT('Ctrl Pts',(1.09779918040499,3.77857036735483,54.8022582795693));
#22420=CARTESIAN_POINT('Ctrl Pts',(1.21144056831204,3.74177775254594,54.7962300950389));
#22421=CARTESIAN_POINT('Ctrl Pts',(1.32186240395243,3.70602750221875,54.7903726938429));
#22422=CARTESIAN_POINT('Ctrl Pts',(1.4307506685698,3.66536892867762,54.784515292647));
#22423=CARTESIAN_POINT('Ctrl Pts',(1.53764429402338,3.61996395355773,54.7786578914511));
#22424=CARTESIAN_POINT('Ctrl Pts',(1.64452247880962,3.57456553713686,54.7728013363504));
#22425=CARTESIAN_POINT('Ctrl Pts',(1.74940621780225,3.52442224372723,54.7669447812497));
#22426=CARTESIAN_POINT('Ctrl Pts',(1.85185417237748,3.46974424478924,54.761088226149));
#22427=CARTESIAN_POINT('Ctrl Pts',(1.95431200970947,3.4150609712768,54.7552311060892));
#22428=CARTESIAN_POINT('Ctrl Pts',(2.05433323159601,3.35584231686793,54.7493739860293));
#22429=CARTESIAN_POINT('Ctrl Pts',(2.15150149351262,3.29234419880621,54.7435168659694));
#22430=CARTESIAN_POINT('Ctrl Pts',(2.25363729230696,3.22559986395605,54.7373603121303));
#22431=CARTESIAN_POINT('Ctrl Pts',(2.3526202827518,3.15412720661996,54.7312037582911));
#22432=CARTESIAN_POINT('Ctrl Pts',(2.44800314821565,3.07827379976606,54.7250472044519));
#22433=CARTESIAN_POINT('Ctrl Pts',(2.53888211483149,3.00600212711658,54.7191813579176));
#22434=CARTESIAN_POINT('Ctrl Pts',(2.62649289859137,2.92975428334712,54.7133155113832));
#22435=CARTESIAN_POINT('Ctrl Pts',(2.71048488963366,2.84987028881449,54.7074496648488));
#22436=CARTESIAN_POINT('Ctrl Pts',(2.79453463138393,2.7699313681254,54.701579785111));
#22437=CARTESIAN_POINT('Ctrl Pts',(2.87496034062874,2.68635161476229,54.6957099053732));
#22438=CARTESIAN_POINT('Ctrl Pts',(2.95145041314914,2.59950561813621,54.6898400256353));
#22439=CARTESIAN_POINT('Ctrl Pts',(3.02804894897422,2.51253647345337,54.6839618223787));
#22440=CARTESIAN_POINT('Ctrl Pts',(3.10070045478603,2.42229216364554,54.6780836191221));
#22441=CARTESIAN_POINT('Ctrl Pts',(3.1691354861231,2.32917780999976,54.6722054158655));
#22442=CARTESIAN_POINT('Ctrl Pts',(3.17909806191479,2.31562248917406,54.6713496838768));
#22443=CARTESIAN_POINT('Ctrl Pts',(3.18897135756376,2.30200638890523,54.6704939518881));
#22444=CARTESIAN_POINT('Ctrl Pts',(3.19875462261016,2.28833080308116,54.6696382198994));
#22445=CARTESIAN_POINT('Ctrl Pts',(3.26594936136754,2.19440230247896,54.663760766191));
#22446=CARTESIAN_POINT('Ctrl Pts',(3.32911355679179,2.09735766200803,54.6578833124826));
#22447=CARTESIAN_POINT('Ctrl Pts',(3.38794523522725,1.99757755371372,54.6520058587742));
#22448=CARTESIAN_POINT('Ctrl Pts',(3.4467017258606,1.89792496595318,54.6461359165433));
#22449=CARTESIAN_POINT('Ctrl Pts',(3.50113650364579,1.79554421518162,54.6402659743123));
#22450=CARTESIAN_POINT('Ctrl Pts',(3.55098941731985,1.69084687600101,54.6343960320814));
#22451=CARTESIAN_POINT('Ctrl Pts',(3.60079188293217,1.58625548404477,54.6285320298685));
#22452=CARTESIAN_POINT('Ctrl Pts',(3.64602153101796,1.47935253706216,54.6226680276557));
#22453=CARTESIAN_POINT('Ctrl Pts',(3.68646324583839,1.37057569549537,54.6168040254428));
#22454=CARTESIAN_POINT('Ctrl Pts',(3.72803726146939,1.25875328312565,54.6107758409126));
#22455=CARTESIAN_POINT('Ctrl Pts',(3.76455104336783,1.1449508738046,54.6047476563823));
#22456=CARTESIAN_POINT('Ctrl Pts',(3.79582305288225,1.02966807817257,54.598719471852));
#22457=CARTESIAN_POINT('Ctrl Pts',(3.82620910112278,0.917651337202903,54.5928620706558));
#22458=CARTESIAN_POINT('Ctrl Pts',(3.8516462818897,0.804237389167053,54.5870046694595));
#22459=CARTESIAN_POINT('Ctrl Pts',(3.87201830941147,0.689900870837413,54.5811472682632));
#22460=CARTESIAN_POINT('Ctrl Pts',(3.892387394216,0.575580868293638,54.5752907131622));
#22461=CARTESIAN_POINT('Ctrl Pts',(3.90769270835451,0.460338966456682,54.5694341580612));
#22462=CARTESIAN_POINT('Ctrl Pts',(3.91786915725888,0.344659638773526,54.5635776029602));
#22463=CARTESIAN_POINT('Ctrl Pts',(3.92804658784575,0.22896915195495,54.5577204829));
#22464=CARTESIAN_POINT('Ctrl Pts',(3.93309413350725,0.112841566336625,54.5518633628399));
#22465=CARTESIAN_POINT('Ctrl Pts',(3.93299866990278,-0.00323458543118984,
54.5460062427797));
#22466=CARTESIAN_POINT('Ctrl Pts',(3.93289832590871,-0.125244902856397,
54.5398496889411));
#22467=CARTESIAN_POINT('Ctrl Pts',(3.92711520564665,-0.247197880111946,
54.5336931351025));
#22468=CARTESIAN_POINT('Ctrl Pts',(3.91569603009031,-0.368528967565535,
54.5275365812639));
#22469=CARTESIAN_POINT('Ctrl Pts',(3.90481605841775,-0.48413090292266,54.5216707347294));
#22470=CARTESIAN_POINT('Ctrl Pts',(3.88882024546085,-0.599167927744024,
54.5158048881948));
#22471=CARTESIAN_POINT('Ctrl Pts',(3.86780182215661,-0.713160616216218,
54.5099390416603));
#22472=CARTESIAN_POINT('Ctrl Pts',(3.84676894713138,-0.827231683095119,
54.5040691619223));
#22473=CARTESIAN_POINT('Ctrl Pts',(3.82070667763449,-0.940256582962956,
54.4981992821843));
#22474=CARTESIAN_POINT('Ctrl Pts',(3.78975850888195,-1.051769672674,54.4923294024463));
#22475=CARTESIAN_POINT('Ctrl Pts',(3.75876645547193,-1.16344088850185,54.4864511991895));
#22476=CARTESIAN_POINT('Ctrl Pts',(3.72287480551736,-1.27359562609761,54.4805729959328));
#22477=CARTESIAN_POINT('Ctrl Pts',(3.68227566039492,-1.38178687244562,54.4746947926761));
#22478=CARTESIAN_POINT('Ctrl Pts',(3.67636535318206,-1.39753704407438,54.4738390606896));
#22479=CARTESIAN_POINT('Ctrl Pts',(3.67035536153618,-1.41324564530154,54.4729833287031));
#22480=CARTESIAN_POINT('Ctrl Pts',(3.66424635914895,-1.42891134065888,54.4721275967165));
#22481=CARTESIAN_POINT('Ctrl Pts',(3.62228768587896,-1.53650858017229,54.4662501429928));
#22482=CARTESIAN_POINT('Ctrl Pts',(3.57551698132201,-1.6424325108648,54.460372689269));
#22483=CARTESIAN_POINT('Ctrl Pts',(3.52408809690542,-1.74622223249203,54.4544952355452));
#22484=CARTESIAN_POINT('Ctrl Pts',(3.47272493940417,-1.84987930923839,54.4486252932988));
#22485=CARTESIAN_POINT('Ctrl Pts',(3.41671562307969,-1.95140723502391,54.4427553510525));
#22486=CARTESIAN_POINT('Ctrl Pts',(3.35626273166703,-2.05036325465096,54.4368854088061));
#22487=CARTESIAN_POINT('Ctrl Pts',(3.29587101483622,-2.14921913691517,54.4310214065777));
#22488=CARTESIAN_POINT('Ctrl Pts',(3.23104488126119,-2.24550794006632,54.4251574043494));
#22489=CARTESIAN_POINT('Ctrl Pts',(3.16203336820224,-2.33881037674616,54.419293402121));
#22490=CARTESIAN_POINT('Ctrl Pts',(3.09108964771404,-2.43472512626092,54.4132652175965));
#22491=CARTESIAN_POINT('Ctrl Pts',(3.01572290971197,-2.52748341109336,54.407237033072));
#22492=CARTESIAN_POINT('Ctrl Pts',(2.93625242311743,-2.61666022015411,54.4012088485476));
#22493=CARTESIAN_POINT('Ctrl Pts',(2.859033399282,-2.70331057853889,54.3953514473358));
#22494=CARTESIAN_POINT('Ctrl Pts',(2.77794032268958,-2.78657934079926,54.389494046124));
#22495=CARTESIAN_POINT('Ctrl Pts',(2.69330719610779,-2.86610979332508,54.3836366449123));
#22496=CARTESIAN_POINT('Ctrl Pts',(2.60868629468924,-2.94562875776339,54.3777800897957));
#22497=CARTESIAN_POINT('Ctrl Pts',(2.52052666065431,-3.02141020385537,54.3719235346792));
#22498=CARTESIAN_POINT('Ctrl Pts',(2.4291985038431,-3.09313491928923,54.3660669795627));
#22499=CARTESIAN_POINT('Ctrl Pts',(2.33786153695993,-3.16486655372732,54.360209859487));
#22500=CARTESIAN_POINT('Ctrl Pts',(2.24335576411272,-3.2325404247759,54.3543527394114));
#22501=CARTESIAN_POINT('Ctrl Pts',(2.14608318887078,-3.29587863041802,54.3484956193358));
#22502=CARTESIAN_POINT('Ctrl Pts',(2.0438377445828,-3.36245487721909,54.342339065519));
#22503=CARTESIAN_POINT('Ctrl Pts',(1.93853554331856,-3.42424014600822,54.3361825117021));
#22504=CARTESIAN_POINT('Ctrl Pts',(1.83067495367516,-3.48096512679837,54.3300259578853));
#22505=CARTESIAN_POINT('Ctrl Pts',(1.72790744989947,-3.5350116019456,54.3241601113355));
#22506=CARTESIAN_POINT('Ctrl Pts',(1.62281805304736,-3.58446462863214,54.3182942647857));
#22507=CARTESIAN_POINT('Ctrl Pts',(1.51585924635706,-3.62914035898775,54.3124284182359));
#22508=CARTESIAN_POINT('Ctrl Pts',(1.40882689757588,-3.67384680721246,54.3065585384828));
#22509=CARTESIAN_POINT('Ctrl Pts',(1.29992296573686,-3.71376927683264,54.3006886587296));
#22510=CARTESIAN_POINT('Ctrl Pts',(1.18961585217552,-3.74877354934286,54.2948187789765));
#22511=CARTESIAN_POINT('Ctrl Pts',(1.07915232258203,-3.78382745808449,54.2889405757048));
#22512=CARTESIAN_POINT('Ctrl Pts',(0.967282037537844,-3.81394914705215,
54.2830623724331));
#22513=CARTESIAN_POINT('Ctrl Pts',(0.854484350536292,-3.8390552867455,54.2771841691615));
#22514=CARTESIAN_POINT('Ctrl Pts',(0.838063588640734,-3.84271016614046,
54.2763284372856));
#22515=CARTESIAN_POINT('Ctrl Pts',(0.82162318178757,-3.84625884217346,54.2754727054096));
#22516=CARTESIAN_POINT('Ctrl Pts',(0.805164616578459,-3.84970114946733,
54.2746169735337));
#22517=CARTESIAN_POINT('Ctrl Pts',(0.692121667573628,-3.87334407112761,
54.2687395198443));
#22518=CARTESIAN_POINT('Ctrl Pts',(0.577851158963191,-3.89204242967716,
54.2628620661548));
#22519=CARTESIAN_POINT('Ctrl Pts',(0.462823177736543,-3.90567327181241,
54.2569846124653));
#22520=CARTESIAN_POINT('Ctrl Pts',(0.347942204061899,-3.91928669351906,
54.2511146702532));
#22521=CARTESIAN_POINT('Ctrl Pts',(0.232306089007898,-3.92784543061053,
54.2452447280411));
#22522=CARTESIAN_POINT('Ctrl Pts',(0.116396346927415,-3.93127725941862,
54.239374785829));
#22523=CARTESIAN_POINT('Ctrl Pts',(0.000603898327194333,-3.9347056154285,
54.2335107836349));
#22524=CARTESIAN_POINT('Ctrl Pts',(-0.115461216568417,-3.93301737104643,
54.2276467814408));
#22525=CARTESIAN_POINT('Ctrl Pts',(-0.231311759198476,-3.92619203173463,
54.2217827792466));
#22526=CARTESIAN_POINT('Ctrl Pts',(-0.350405925026531,-3.91917559423354,
54.2157545947093));
#22527=CARTESIAN_POINT('Ctrl Pts',(-0.469272885050501,-3.90673009317892,
54.209726410172));
#22528=CARTESIAN_POINT('Ctrl Pts',(-0.587382235703046,-3.88889072991007,
54.2036982256347));
#22529=CARTESIAN_POINT('Ctrl Pts',(-0.702145452613,-3.8715567702782,54.1978408244568));
#22530=CARTESIAN_POINT('Ctrl Pts',(-0.816192976570165,-3.84913053608896,
54.1919834232789));
#22531=CARTESIAN_POINT('Ctrl Pts',(-0.929043557234587,-3.82169688342246,
54.186126022101));
#22532=CARTESIAN_POINT('Ctrl Pts',(-1.04187783675824,-3.79426719351655,
54.1802694670182));
#22533=CARTESIAN_POINT('Ctrl Pts',(-1.15351511607574,-3.761831620883,54.1744129119354));
#22534=CARTESIAN_POINT('Ctrl Pts',(-1.26348577260973,-3.72452583591694,
54.1685563568526));
#22535=CARTESIAN_POINT('Ctrl Pts',(-1.37346703758901,-3.68721645220563,
54.1626992368106));
#22536=CARTESIAN_POINT('Ctrl Pts',(-1.48178096953255,-3.64503605474311,
54.1568421167685));
#22537=CARTESIAN_POINT('Ctrl Pts',(-1.58797517510659,-3.59816951285584,
54.1509849967264));
#22538=CARTESIAN_POINT('Ctrl Pts',(-1.69959835203152,-3.54890701055015,
54.1448284428617));
#22539=CARTESIAN_POINT('Ctrl Pts',(-1.80887886874512,-3.4944667502624,54.1386718889971));
#22540=CARTESIAN_POINT('Ctrl Pts',(-1.91531887921463,-3.43511900680662,
54.1325153351325));
#22541=CARTESIAN_POINT('Ctrl Pts',(-2.01673288101222,-3.3785736143836,54.1266494886154));
#22542=CARTESIAN_POINT('Ctrl Pts',(-2.1155681723429,-3.31757387487189,54.1207836420982));
#22543=CARTESIAN_POINT('Ctrl Pts',(-2.21142355605467,-3.25239832365695,
54.1149177955811));
#22544=CARTESIAN_POINT('Ctrl Pts',(-2.30734484743756,-3.18717795942653,
54.1090479158604));
#22545=CARTESIAN_POINT('Ctrl Pts',(-2.40028182175256,-3.11777631243909,
54.1031780361396));
#22546=CARTESIAN_POINT('Ctrl Pts',(-2.48986615243409,-3.04451236538187,
54.0973081564188));
#22547=CARTESIAN_POINT('Ctrl Pts',(-2.57957751414965,-2.97114452967715,
54.0914299531789));
#22548=CARTESIAN_POINT('Ctrl Pts',(-2.66592643995281,-2.89390373942269,
54.085551749939));
#22549=CARTESIAN_POINT('Ctrl Pts',(-2.74858124202434,-2.81314595355307,
54.0796735466991));
#22550=CARTESIAN_POINT('Ctrl Pts',(-2.7606138931248,-2.80138946467812,54.078817814583));
#22551=CARTESIAN_POINT('Ctrl Pts',(-2.77256832580449,-2.78955849781866,
54.0779620824669));
#22552=CARTESIAN_POINT('Ctrl Pts',(-2.7844435893455,-2.77765420773588,54.0771063503508));
#22553=CARTESIAN_POINT('Ctrl Pts',(-2.86487758717835,-2.69702360619902,
54.0713102722314));
#22554=CARTESIAN_POINT('Ctrl Pts',(-2.94195621667249,-2.61274587632333,
54.0655141941119));
#22555=CARTESIAN_POINT('Ctrl Pts',(-3.01532404489709,-2.52513562096484,
54.0597181159925));
#22556=CARTESIAN_POINT('Ctrl Pts',(-3.08857726562201,-2.43766222112678,
54.0539310918962));
#22557=CARTESIAN_POINT('Ctrl Pts',(-3.1581309477068,-2.34686697586053,54.0481440678));
#22558=CARTESIAN_POINT('Ctrl Pts',(-3.2236657095407,-2.25310194912071,54.0423570437038));
#22559=CARTESIAN_POINT('Ctrl Pts',(-3.28914205744857,-2.15942049914507,
54.0365751778288));
#22560=CARTESIAN_POINT('Ctrl Pts',(-3.35060635987211,-2.06277487262656,
54.0307933119538));
#22561=CARTESIAN_POINT('Ctrl Pts',(-3.40777900761285,-1.96355067041145,
54.0250114460788));
#22562=CARTESIAN_POINT('Ctrl Pts',(-3.46491539869334,-1.86438939231005,
54.0192332468372));
#22563=CARTESIAN_POINT('Ctrl Pts',(-3.51776533204567,-1.76265315515072,
54.0134550475958));
#22564=CARTESIAN_POINT('Ctrl Pts',(-3.56609260362719,-1.65875632398357,
54.0076768483543));
#22565=CARTESIAN_POINT('Ctrl Pts',(-3.61440165302202,-1.55489866795281,
54.0019008278293));
#22566=CARTESIAN_POINT('Ctrl Pts',(-3.65819125215211,-1.44888242258307,
53.9961248073043));
#22567=CARTESIAN_POINT('Ctrl Pts',(-3.69727164606475,-1.34114554586955,
53.9903487867793));
#22568=CARTESIAN_POINT('Ctrl Pts',(-3.73636210810007,-1.23338091334337,
53.9845712782017));
#22569=CARTESIAN_POINT('Ctrl Pts',(-3.77074078579598,-1.1238951600797,53.9787937696241));
#22570=CARTESIAN_POINT('Ctrl Pts',(-3.80026663420399,-1.01314486079533,
53.9730162610465));
#22571=CARTESIAN_POINT('Ctrl Pts',(-3.82979492306188,-0.902385407479146,
53.9672382749307));
#22572=CARTESIAN_POINT('Ctrl Pts',(-3.85446948338104,-0.790361613535798,
53.9614602888149));
#22573=CARTESIAN_POINT('Ctrl Pts',(-3.87419996464605,-0.677542348445218,
53.9556823026991));
#22574=CARTESIAN_POINT('Ctrl Pts',(-3.89395032833318,-0.56460939528879,
53.949898494102));
#22575=CARTESIAN_POINT('Ctrl Pts',(-3.90874659429761,-0.450879790525878,
53.9441146855048));
#22576=CARTESIAN_POINT('Ctrl Pts',(-3.91855008018397,-0.336829733085216,
53.9383308769077));
#22577=CARTESIAN_POINT('Ctrl Pts',(-3.92828591345906,-0.223566720609123,
53.9325869816393));
#22578=CARTESIAN_POINT('Ctrl Pts',(-3.93309771233674,-0.109988077799192,
53.9268430863709));
#22579=CARTESIAN_POINT('Ctrl Pts',(-3.93299849539527,0.00344023525537207,
53.9210991911024));
#22580=CARTESIAN_POINT('',(-3.93299921172447,-0.00249009532928107,52.6710991910122));
#22581=CARTESIAN_POINT('Ctrl Pts',(-3.93299849539445,0.003440236192082,
53.921099191055));
#22582=CARTESIAN_POINT('Ctrl Pts',(-3.93285730429221,0.164854848927317,
53.9129253180124));
#22583=CARTESIAN_POINT('Ctrl Pts',(-3.92277566495795,0.325846686158594,
53.9047514449697));
#22584=CARTESIAN_POINT('Ctrl Pts',(-3.90292980314051,0.485415236429215,
53.8965775719271));
#22585=CARTESIAN_POINT('Ctrl Pts',(-3.88918603920976,0.5959205148528,53.8909169570073));
#22586=CARTESIAN_POINT('Ctrl Pts',(-3.87076040826518,0.705743982120764,
53.8852563420876));
#22587=CARTESIAN_POINT('Ctrl Pts',(-3.84772403021341,0.814560487206655,
53.8795957271679));
#22588=CARTESIAN_POINT('Ctrl Pts',(-3.8238052069376,0.927545382175443,53.8737182733602));
#22589=CARTESIAN_POINT('Ctrl Pts',(-3.79486641686709,1.03966105773686,53.8678408195524));
#22590=CARTESIAN_POINT('Ctrl Pts',(-3.76098458040149,1.15042774044366,53.8619633657447));
#22591=CARTESIAN_POINT('Ctrl Pts',(-3.72714604544839,1.26105286161199,53.856093423414));
#22592=CARTESIAN_POINT('Ctrl Pts',(-3.68837714723683,1.37033202765081,53.8502234810834));
#22593=CARTESIAN_POINT('Ctrl Pts',(-3.64480583910922,1.47779545106737,53.8443535387528));
#22594=CARTESIAN_POINT('Ctrl Pts',(-3.60127862244515,1.58515012815939,53.83848953644));
#22595=CARTESIAN_POINT('Ctrl Pts',(-3.55295881680666,1.69069233749325,53.8326255341273));
#22596=CARTESIAN_POINT('Ctrl Pts',(-3.50002402481952,1.79396789984834,53.8267615318145));
#22597=CARTESIAN_POINT('Ctrl Pts',(-3.445607147886,1.90013500386344,53.8207333473216));
#22598=CARTESIAN_POINT('Ctrl Pts',(-3.38631316709253,2.00390623425911,53.8147051628287));
#22599=CARTESIAN_POINT('Ctrl Pts',(-3.32238805348545,2.10481035299079,53.8086769783358));
#22600=CARTESIAN_POINT('Ctrl Pts',(-3.26027398850708,2.20285577886221,53.8028195770397));
#22601=CARTESIAN_POINT('Ctrl Pts',(-3.19378791043858,2.29819399583277,53.7969621757437));
#22602=CARTESIAN_POINT('Ctrl Pts',(-3.12320142531508,2.39041876183023,53.7911047744476));
#22603=CARTESIAN_POINT('Ctrl Pts',(-3.05262513633502,2.48263020605734,53.785248219247));
#22604=CARTESIAN_POINT('Ctrl Pts',(-2.97794986875202,2.57172876613824,53.7793916640464));
#22605=CARTESIAN_POINT('Ctrl Pts',(-2.89948904773072,2.65733932008874,53.7735351088458));
#22606=CARTESIAN_POINT('Ctrl Pts',(-2.82102065790323,2.74295813255197,53.7676779886864));
#22607=CARTESIAN_POINT('Ctrl Pts',(-2.73876626741577,2.82508796588879,53.7618208685269));
#22608=CARTESIAN_POINT('Ctrl Pts',(-2.65307738474624,2.90338929366148,53.7559637483675));
#22609=CARTESIAN_POINT('Ctrl Pts',(-2.56300782954424,2.98569362001629,53.749807194669));
#22610=CARTESIAN_POINT('Ctrl Pts',(-2.4691437019627,3.06376729023432,53.7436506409704));
#22611=CARTESIAN_POINT('Ctrl Pts',(-2.37193299098857,3.13726359846604,53.7374940872719));
#22612=CARTESIAN_POINT('Ctrl Pts',(-2.27931248453441,3.20728947547813,53.7316282406398));
#22613=CARTESIAN_POINT('Ctrl Pts',(-2.18365459889173,3.27316020083352,53.7257623940077));
#22614=CARTESIAN_POINT('Ctrl Pts',(-2.08537593326546,3.33462085055516,53.7198965473756));
#22615=CARTESIAN_POINT('Ctrl Pts',(-1.9870296937972,3.3961237590133,53.7140266675407));
#22616=CARTESIAN_POINT('Ctrl Pts',(-1.88605944427407,3.45321035146174,53.7081567877058));
#22617=CARTESIAN_POINT('Ctrl Pts',(-1.7829055542137,3.50567208745398,53.7022869078708));
#22618=CARTESIAN_POINT('Ctrl Pts',(-1.67960539145098,3.55820821443516,53.6964087045186));
#22619=CARTESIAN_POINT('Ctrl Pts',(-1.57411578352132,3.60610622928743,53.6905305011664));
#22620=CARTESIAN_POINT('Ctrl Pts',(-1.46689617496833,3.64920602485846,53.6846522978142));
#22621=CARTESIAN_POINT('Ctrl Pts',(-1.45128746479236,3.65548036428938,53.6837965665378));
#22622=CARTESIAN_POINT('Ctrl Pts',(-1.43564211492558,3.6616531036275,53.6829408352614));
#22623=CARTESIAN_POINT('Ctrl Pts',(-1.41996156534227,3.66772383815232,53.682085103985));
#22624=CARTESIAN_POINT('Ctrl Pts',(-1.3122622163181,3.70941970811829,53.6762076504611));
#22625=CARTESIAN_POINT('Ctrl Pts',(-1.20254823139564,3.74643617145609,53.6703301969372));
#22626=CARTESIAN_POINT('Ctrl Pts',(-1.09126347367353,3.77857552935309,53.6644527434132));
#22627=CARTESIAN_POINT('Ctrl Pts',(-0.980120939606572,3.8106738126497,53.6585828013665));
#22628=CARTESIAN_POINT('Ctrl Pts',(-0.867412017898489,3.8379072730176,53.6527128593198));
#22629=CARTESIAN_POINT('Ctrl Pts',(-0.75360008967137,3.86012641047509,53.646842917273));
#22630=CARTESIAN_POINT('Ctrl Pts',(-0.639903332063104,3.88232306354231,
53.6409789152439));
#22631=CARTESIAN_POINT('Ctrl Pts',(-0.525106190717566,3.89951540851951,
53.6351149132148));
#22632=CARTESIAN_POINT('Ctrl Pts',(-0.409686099805357,3.91160405711343,
53.6292509111857));
#22633=CARTESIAN_POINT('Ctrl Pts',(-0.291034433070842,3.92403116831133,
53.6232227265864));
#22634=CARTESIAN_POINT('Ctrl Pts',(-0.171724843581924,3.93106444109953,
53.6171945419871));
#22635=CARTESIAN_POINT('Ctrl Pts',(-0.0522864064142289,3.93265242955747,
53.6111663573878));
#22636=CARTESIAN_POINT('Ctrl Pts',(0.0637682384864407,3.93419542895501,
53.605308956373));
#22637=CARTESIAN_POINT('Ctrl Pts',(0.179944088795455,3.93059753512055,53.5994515553583));
#22638=CARTESIAN_POINT('Ctrl Pts',(0.295752501716406,3.92186428344078,53.5935941543435));
#22639=CARTESIAN_POINT('Ctrl Pts',(0.411544186260149,3.91313229326806,53.5877375994228));
#22640=CARTESIAN_POINT('Ctrl Pts',(0.526968127731309,3.89926645134358,53.5818810445021));
#22641=CARTESIAN_POINT('Ctrl Pts',(0.641538900322014,3.88032432141614,53.5760244895814));
#22642=CARTESIAN_POINT('Ctrl Pts',(0.756120725136563,3.86138036421062,53.5701673697003));
#22643=CARTESIAN_POINT('Ctrl Pts',(0.869848810469708,3.83735921282958,53.5643102498191));
#22644=CARTESIAN_POINT('Ctrl Pts',(0.982246737016988,3.80836977558895,53.558453129938));
#22645=CARTESIAN_POINT('Ctrl Pts',(1.10039079569383,3.77789830801322,53.5522965758434));
#22646=CARTESIAN_POINT('Ctrl Pts',(1.21706460083901,3.74193725081163,53.5461400217487));
#22647=CARTESIAN_POINT('Ctrl Pts',(1.33173300771971,3.70067239784202,53.5399834676541));
#22648=CARTESIAN_POINT('Ctrl Pts',(1.44098686090307,3.66135603939059,53.5341176212935));
#22649=CARTESIAN_POINT('Ctrl Pts',(1.5484200079586,3.61722553696908,53.5282517749329));
#22650=CARTESIAN_POINT('Ctrl Pts',(1.65359132669396,3.56849053862869,53.5223859285724));
#22651=CARTESIAN_POINT('Ctrl Pts',(1.7588349585249,3.51972203135606,53.5165160490066));
#22652=CARTESIAN_POINT('Ctrl Pts',(1.86181330011028,3.46634291336468,53.5106461694409));
#22653=CARTESIAN_POINT('Ctrl Pts',(1.96211109121973,3.40860808332558,53.5047762898751));
#22654=CARTESIAN_POINT('Ctrl Pts',(2.06255110516054,3.35079138497308,53.4988980867872));
#22655=CARTESIAN_POINT('Ctrl Pts',(2.16030263759414,3.28860687062497,53.4930198836992));
#22656=CARTESIAN_POINT('Ctrl Pts',(2.25498057231444,3.22235187688812,53.4871416806113));
#22657=CARTESIAN_POINT('Ctrl Pts',(2.26876353582098,3.21270665000924,53.4862859473416));
#22658=CARTESIAN_POINT('Ctrl Pts',(2.28248142121484,3.20297522571995,53.4854302140719));
#22659=CARTESIAN_POINT('Ctrl Pts',(2.29613310278219,3.1931585889692,53.4845744808022));
#22660=CARTESIAN_POINT('Ctrl Pts',(2.3898972809373,3.12573474285618,53.478697027072));
#22661=CARTESIAN_POINT('Ctrl Pts',(2.48084288367599,3.0540669316364,53.4728195733417));
#22662=CARTESIAN_POINT('Ctrl Pts',(2.56856182247688,2.97841890339727,53.4669421196115));
#22663=CARTESIAN_POINT('Ctrl Pts',(2.65616865508283,2.90286755453795,53.4610721773603));
#22664=CARTESIAN_POINT('Ctrl Pts',(2.74055671523021,2.82334637202897,53.4552022351091));
#22665=CARTESIAN_POINT('Ctrl Pts',(2.82134762001191,2.74016178483189,53.449332292858));
#22666=CARTESIAN_POINT('Ctrl Pts',(2.9020567693786,2.65706137530885,53.4434682906265));
#22667=CARTESIAN_POINT('Ctrl Pts',(2.97917571841164,2.57030522942354,53.437604288395));
#22668=CARTESIAN_POINT('Ctrl Pts',(3.05236037773252,2.48023892487166,53.4317402861635));
#22669=CARTESIAN_POINT('Ctrl Pts',(3.12759408556559,2.38765091387129,53.4257121016409));
#22670=CARTESIAN_POINT('Ctrl Pts',(3.19866960110609,2.29156493349301,53.4196839171182));
#22671=CARTESIAN_POINT('Ctrl Pts',(3.26525477551063,2.19239600688493,53.4136557325955));
#22672=CARTESIAN_POINT('Ctrl Pts',(3.32995353841542,2.09603661566131,53.4077983313847));
#22673=CARTESIAN_POINT('Ctrl Pts',(3.39041272939229,1.99676698273288,53.4019409301739));
#22674=CARTESIAN_POINT('Ctrl Pts',(3.44637001481703,1.89499939867272,53.3960835289631));
#22675=CARTESIAN_POINT('Ctrl Pts',(3.50231921725811,1.79324651485602,53.390226973849));
#22676=CARTESIAN_POINT('Ctrl Pts',(3.55376760858011,1.68899675879178,53.384370418735));
#22677=CARTESIAN_POINT('Ctrl Pts',(3.60049818948871,1.58268815231823,53.378513863621));
#22678=CARTESIAN_POINT('Ctrl Pts',(3.64723327830258,1.47636929069443,53.3726567435493));
#22679=CARTESIAN_POINT('Ctrl Pts',(3.68924948598868,1.3679915614872,53.3667996234777));
#22680=CARTESIAN_POINT('Ctrl Pts',(3.72637773796442,1.25801349515936,53.3609425034061));
#22681=CARTESIAN_POINT('Ctrl Pts',(3.76540409879904,1.14241301649401,53.3547859495905));
#22682=CARTESIAN_POINT('Ctrl Pts',(3.79902934229234,1.0250447242216,53.348629395775));
#22683=CARTESIAN_POINT('Ctrl Pts',(3.82711670531169,0.90645834097553,53.3424728419594));
#22684=CARTESIAN_POINT('Ctrl Pts',(3.85387780676215,0.793471506629281,53.3366069954173));
#22685=CARTESIAN_POINT('Ctrl Pts',(3.87561204479805,0.679379411978636,53.3307411488752));
#22686=CARTESIAN_POINT('Ctrl Pts',(3.89225400468771,0.564666063255461,53.3248753023331));
#22687=CARTESIAN_POINT('Ctrl Pts',(3.90890740715212,0.449873840644997,53.3190054225889));
#22688=CARTESIAN_POINT('Ctrl Pts',(3.920461518559,0.334459922704503,53.3131355428447));
#22689=CARTESIAN_POINT('Ctrl Pts',(3.92690295383275,0.218911377455589,53.3072656631005));
#22690=CARTESIAN_POINT('Ctrl Pts',(3.93335352309169,0.103198983832043,53.3013874598396));
#22691=CARTESIAN_POINT('Ctrl Pts',(3.93467694536156,-0.012648007394774,
53.2955092565786));
#22692=CARTESIAN_POINT('Ctrl Pts',(3.93091184894263,-0.128144589594604,
53.2896310533176));
#22693=CARTESIAN_POINT('Ctrl Pts',(3.93036373705076,-0.144958249360539,
53.2887753214182));
#22694=CARTESIAN_POINT('Ctrl Pts',(3.92970787483743,-0.161764496431242,
53.2879195895187));
#22695=CARTESIAN_POINT('Ctrl Pts',(3.92894447221929,-0.178561849837614,
53.2870638576193));
#22696=CARTESIAN_POINT('Ctrl Pts',(3.92370116635798,-0.293931720830033,
53.28118640321));
#22697=CARTESIAN_POINT('Ctrl Pts',(3.91336336805461,-0.409259562022228,
53.2753089488007));
#22698=CARTESIAN_POINT('Ctrl Pts',(3.89792902249375,-0.524059477159622,
53.2694314943914));
#22699=CARTESIAN_POINT('Ctrl Pts',(3.88251440225738,-0.638712676288338,
53.2635615514567));
#22700=CARTESIAN_POINT('Ctrl Pts',(3.86201624293027,-0.752838885977837,
53.2576916085221));
#22701=CARTESIAN_POINT('Ctrl Pts',(3.83648446702211,-0.865953771455513,
53.2518216655874));
#22702=CARTESIAN_POINT('Ctrl Pts',(3.81097852767865,-0.978954191724504,
53.2459576626689));
#22703=CARTESIAN_POINT('Ctrl Pts',(3.78044919428983,-1.09094492343176,53.2400936597504));
#22704=CARTESIAN_POINT('Ctrl Pts',(3.74499791492547,-1.20144896570924,53.2342296568319));
#22705=CARTESIAN_POINT('Ctrl Pts',(3.70855406463075,-1.3150469188982,53.2282014725654));
#22706=CARTESIAN_POINT('Ctrl Pts',(3.6669086386595,-1.4270732622134,53.2221732882989));
#22707=CARTESIAN_POINT('Ctrl Pts',(3.62022777324901,-1.5370230544128,53.2161451040324));
#22708=CARTESIAN_POINT('Ctrl Pts',(3.57486940698688,-1.64385789779391,53.2102877021302));
#22709=CARTESIAN_POINT('Ctrl Pts',(3.52475725730696,-1.74873186593735,53.2044303002279));
#22710=CARTESIAN_POINT('Ctrl Pts',(3.47009331534487,-1.85119998455024,53.1985728983256));
#22711=CARTESIAN_POINT('Ctrl Pts',(3.41543726953916,-1.95365330173717,53.1927163425197));
#22712=CARTESIAN_POINT('Ctrl Pts',(3.35623093302101,-2.05370109659577,53.1868597867138));
#22713=CARTESIAN_POINT('Ctrl Pts',(3.29272261672546,-2.15092230666395,53.1810032309079));
#22714=CARTESIAN_POINT('Ctrl Pts',(3.22920817405052,-2.24815289525218,53.1751461101448));
#22715=CARTESIAN_POINT('Ctrl Pts',(3.16139115222987,-2.34255601164886,53.1692889893816));
#22716=CARTESIAN_POINT('Ctrl Pts',(3.0895632229923,-2.43373952820209,53.1634318686185));
#22717=CARTESIAN_POINT('Ctrl Pts',(3.01406325291621,-2.52958459632918,53.15727531577));
#22718=CARTESIAN_POINT('Ctrl Pts',(2.9341317409814,-2.62187176497204,53.1511187629214));
#22719=CARTESIAN_POINT('Ctrl Pts',(2.85015439061182,-2.71018614668367,53.1449622100729));
#22720=CARTESIAN_POINT('Ctrl Pts',(2.77014235792697,-2.79433042088328,53.1390963628466));
#22721=CARTESIAN_POINT('Ctrl Pts',(2.6864581807883,-2.87486826708975,53.1332305156203));
#22722=CARTESIAN_POINT('Ctrl Pts',(2.59947150285008,-2.95148046001838,53.1273646683939));
#22723=CARTESIAN_POINT('Ctrl Pts',(2.51242501520104,-3.02814532943969,53.1214947879681));
#22724=CARTESIAN_POINT('Ctrl Pts',(2.42207182567495,-3.10087891295247,53.1156249075422));
#22725=CARTESIAN_POINT('Ctrl Pts',(2.32881256873694,-3.1694038902754,53.1097550271164));
#22726=CARTESIAN_POINT('Ctrl Pts',(2.23542106987779,-3.23802603623278,53.1038768231816));
#22727=CARTESIAN_POINT('Ctrl Pts',(2.13911562234646,-3.30242743961088,53.0979986192467));
#22728=CARTESIAN_POINT('Ctrl Pts',(2.04032355156761,-3.36237547054437,53.0921204153119));
#22729=CARTESIAN_POINT('Ctrl Pts',(2.02594177114823,-3.3711024808263,53.0912646883534));
#22730=CARTESIAN_POINT('Ctrl Pts',(2.01150733054545,-3.37973519521384,53.0904089613949));
#22731=CARTESIAN_POINT('Ctrl Pts',(1.99702158481975,-3.38827298040816,53.0895532344364));
#22732=CARTESIAN_POINT('Ctrl Pts',(1.8975280770807,-3.44691367543279,53.0836757823273));
#22733=CARTESIAN_POINT('Ctrl Pts',(1.79528639897419,-3.50126448233823,53.0777983302181));
#22734=CARTESIAN_POINT('Ctrl Pts',(1.69070239339066,-3.55105821086941,53.071920878109));
#22735=CARTESIAN_POINT('Ctrl Pts',(1.58625204782377,-3.60078830222637,53.0660509374768));
#22736=CARTESIAN_POINT('Ctrl Pts',(1.47946569731972,-3.64597272201073,53.0601809968447));
#22737=CARTESIAN_POINT('Ctrl Pts',(1.37077627475081,-3.68638866705347,53.0543110562125));
#22738=CARTESIAN_POINT('Ctrl Pts',(1.26219683913274,-3.72676371366787,53.048447055596));
#22739=CARTESIAN_POINT('Ctrl Pts',(1.15171854657812,-3.76237974113116,53.0425830549794));
#22740=CARTESIAN_POINT('Ctrl Pts',(1.03979633838236,-3.79306110874668,53.0367190543629));
#22741=CARTESIAN_POINT('Ctrl Pts',(0.924740451585198,-3.82460151539216,
53.0306908692334));
#22742=CARTESIAN_POINT('Ctrl Pts',(0.80815899767297,-3.85092665468197,53.0246626841038));
#22743=CARTESIAN_POINT('Ctrl Pts',(0.690565662773502,-3.87189980053696,
53.0186344989742));
#22744=CARTESIAN_POINT('Ctrl Pts',(0.576303884167373,-3.89227875271488,
53.0127770993584));
#22745=CARTESIAN_POINT('Ctrl Pts',(0.461087223141258,-3.90760481946477,
53.0069196997425));
#22746=CARTESIAN_POINT('Ctrl Pts',(0.345398728597537,-3.91780406838872,
53.0010623001266));
#22747=CARTESIAN_POINT('Ctrl Pts',(0.229726944965099,-3.92800184405688,
52.9952057465973));
#22748=CARTESIAN_POINT('Ctrl Pts',(0.113583874145427,-3.93307423829894,
52.989349193068));
#22749=CARTESIAN_POINT('Ctrl Pts',(-0.00254215567874407,-3.932999178419,
52.9834926395388));
#22750=CARTESIAN_POINT('Ctrl Pts',(-0.118679387937313,-3.93292411129818,
52.97763552104));
#22751=CARTESIAN_POINT('Ctrl Pts',(-0.234799163415466,-3.92770060319777,
52.9717784025413));
#22752=CARTESIAN_POINT('Ctrl Pts',(-0.35041369833918,-3.91735870709031,
52.9659212840426));
#22753=CARTESIAN_POINT('Ctrl Pts',(-0.471938876023687,-3.90648809499225,
52.9597647279769));
#22754=CARTESIAN_POINT('Ctrl Pts',(-0.592905280379541,-3.88996194967868,
52.9536081719111));
#22755=CARTESIAN_POINT('Ctrl Pts',(-0.712754689367659,-3.86787664653159,
52.9474516158453));
#22756=CARTESIAN_POINT('Ctrl Pts',(-0.82694483895059,-3.84683420592847,
52.941585770832));
#22757=CARTESIAN_POINT('Ctrl Pts',(-0.940120674119461,-3.82074576729556,
52.9357199258187));
#22758=CARTESIAN_POINT('Ctrl Pts',(-1.05181287110385,-3.78974651977943,
52.9298540808053));
#22759=CARTESIAN_POINT('Ctrl Pts',(-1.16358186502298,-3.75872595790784,
52.9239842025745));
#22760=CARTESIAN_POINT('Ctrl Pts',(-1.27386479835553,-3.72278799109742,
52.9181143243438));
#22761=CARTESIAN_POINT('Ctrl Pts',(-1.38221051337374,-3.6821166598465,52.912244446113));
#22762=CARTESIAN_POINT('Ctrl Pts',(-1.49070986372734,-3.64138765623062,
52.9063662443346));
#22763=CARTESIAN_POINT('Ctrl Pts',(-1.5972661367457,-3.59591205639966,52.9004880425563));
#22764=CARTESIAN_POINT('Ctrl Pts',(-1.7014510229078,-3.54592067263864,52.894609840778));
#22765=CARTESIAN_POINT('Ctrl Pts',(-1.716618162216,-3.53864297325589,52.8937540976032));
#22766=CARTESIAN_POINT('Ctrl Pts',(-1.73173509228498,-3.53126964581346,
52.8928983544283));
#22767=CARTESIAN_POINT('Ctrl Pts',(-1.74680054228167,-3.52380147929541,
52.8920426112535));
#22768=CARTESIAN_POINT('Ctrl Pts',(-1.85027375514464,-3.47250827637161,
52.8861651568326));
#22769=CARTESIAN_POINT('Ctrl Pts',(-1.95165540109902,-3.41656954182265,
52.8802877024118));
#22770=CARTESIAN_POINT('Ctrl Pts',(-2.05049996068643,-3.35617921321627,
52.8744102479909));
#22771=CARTESIAN_POINT('Ctrl Pts',(-2.14921819519744,-3.29586606450635,
52.8685403050597));
#22772=CARTESIAN_POINT('Ctrl Pts',(-2.2454054428876,-3.23111284935119,52.8626703621284));
#22773=CARTESIAN_POINT('Ctrl Pts',(-2.33863856043279,-3.16216044559047,
52.8568004191971));
#22774=CARTESIAN_POINT('Ctrl Pts',(-2.43177733164452,-3.09327781753444,
52.8509364162967));
#22775=CARTESIAN_POINT('Ctrl Pts',(-2.52196758939371,-3.02020469736552,
52.8450724133962));
#22776=CARTESIAN_POINT('Ctrl Pts',(-2.60881366733854,-2.94322616343149,
52.8392084104958));
#22777=CARTESIAN_POINT('Ctrl Pts',(-2.69809127679203,-2.86409237119243,
52.8331802262281));
#22778=CARTESIAN_POINT('Ctrl Pts',(-2.78383429546973,-2.78083147187155,
52.8271520419603));
#22779=CARTESIAN_POINT('Ctrl Pts',(-2.86564755563438,-2.69379900640095,
52.8211238576926));
#22780=CARTESIAN_POINT('Ctrl Pts',(-2.94514299240547,-2.6092322278381,52.8152664558444));
#22781=CARTESIAN_POINT('Ctrl Pts',(-3.0209280456164,-2.52110503640395,52.8094090539962));
#22782=CARTESIAN_POINT('Ctrl Pts',(-3.09267687884802,-2.42978162044224,
52.8035516521479));
#22783=CARTESIAN_POINT('Ctrl Pts',(-3.16441534786508,-2.33847139626965,
52.7976950964092));
#22784=CARTESIAN_POINT('Ctrl Pts',(-3.2321185015145,-2.2439661899538,52.7918385406705));
#22785=CARTESIAN_POINT('Ctrl Pts',(-3.29550105450613,-2.14666294507291,
52.7859819849317));
#22786=CARTESIAN_POINT('Ctrl Pts',(-3.35888972160454,-2.04935031397446,
52.7801248642488));
#22787=CARTESIAN_POINT('Ctrl Pts',(-3.4179567343685,-1.94923945340892,52.7742677435658));
#22788=CARTESIAN_POINT('Ctrl Pts',(-3.47246076316776,-1.84675532983134,
52.7684106228828));
#22789=CARTESIAN_POINT('Ctrl Pts',(-3.52975118875137,-1.73903193424627,
52.7622540699818));
#22790=CARTESIAN_POINT('Ctrl Pts',(-3.58199950153473,-1.62868664782208,
52.7560975170808));
#22791=CARTESIAN_POINT('Ctrl Pts',(-3.62898143730125,-1.51623966697981,
52.7499409641798));
#22792=CARTESIAN_POINT('Ctrl Pts',(-3.67374493674294,-1.40910231126998,
52.7440751170653));
#22793=CARTESIAN_POINT('Ctrl Pts',(-3.71372795068742,-1.30005762113249,
52.7382092699509));
#22794=CARTESIAN_POINT('Ctrl Pts',(-3.74878729262083,-1.18957254284247,
52.7323434228364));
#22795=CARTESIAN_POINT('Ctrl Pts',(-3.78387074035469,-1.07901149817362,
52.7264735425333));
#22796=CARTESIAN_POINT('Ctrl Pts',(-3.81402366807081,-0.967008490512607,
52.7206036622302));
#22797=CARTESIAN_POINT('Ctrl Pts',(-3.83915373006062,-0.854041940985162,
52.7147337819271));
#22798=CARTESIAN_POINT('Ctrl Pts',(-3.8643194264966,-0.740915204808353,
52.7088555781295));
#22799=CARTESIAN_POINT('Ctrl Pts',(-3.88444797384919,-0.626822604870012,
52.7029773743318));
#22800=CARTESIAN_POINT('Ctrl Pts',(-3.8994986835627,-0.51224897939661,52.6970991705342));
#22801=CARTESIAN_POINT('Ctrl Pts',(-3.90168971103587,-0.49556976852276,
52.6962434430463));
#22802=CARTESIAN_POINT('Ctrl Pts',(-3.90377321667196,-0.478880364767715,
52.6953877155585));
#22803=CARTESIAN_POINT('Ctrl Pts',(-3.90574916697184,-0.462182263505258,
52.6945319880707));
#22804=CARTESIAN_POINT('Ctrl Pts',(-3.9237852991702,-0.309764886484231,
52.6867210557321));
#22805=CARTESIAN_POINT('Ctrl Pts',(-3.93290184813808,-0.156271669277873,
52.6789101233936));
#22806=CARTESIAN_POINT('Ctrl Pts',(-3.93299921172394,-0.00249009617154345,
52.671099191055));
#22807=CARTESIAN_POINT('',(-3.93076159747888,-0.00108900750095069,51.4210992232121));
#22808=CARTESIAN_POINT('Ctrl Pts',(-3.93299921172447,-0.00249009532928107,
52.6710991910122));
#22809=CARTESIAN_POINT('Ctrl Pts',(-3.93307142957185,0.111574909923686,
52.6653055577425));
#22810=CARTESIAN_POINT('Ctrl Pts',(-3.92817727933913,0.22583195648946,52.6595119244728));
#22811=CARTESIAN_POINT('Ctrl Pts',(-3.91829309654896,0.339806135225414,
52.6537182912031));
#22812=CARTESIAN_POINT('Ctrl Pts',(-3.90841996795221,0.453652848429453,
52.6479311373707));
#22813=CARTESIAN_POINT('Ctrl Pts',(-3.89356793662517,0.567216902680455,
52.6421439835383));
#22814=CARTESIAN_POINT('Ctrl Pts',(-3.87376536650919,0.680022709351676,
52.6363568297059));
#22815=CARTESIAN_POINT('Ctrl Pts',(-3.85389952520209,0.793188941852033,
52.6305511853385));
#22816=CARTESIAN_POINT('Ctrl Pts',(-3.82905145330541,0.90559164150953,52.624745540971));
#22817=CARTESIAN_POINT('Ctrl Pts',(-3.79930239470142,1.01675479522654,52.6189398966036));
#22818=CARTESIAN_POINT('Ctrl Pts',(-3.76968670854771,1.12741957679704,52.6131602803881));
#22819=CARTESIAN_POINT('Ctrl Pts',(-3.73521399798968,1.23685548968949,52.6073806641725));
#22820=CARTESIAN_POINT('Ctrl Pts',(-3.69601554610006,1.34460331807814,52.6016010479569));
#22821=CARTESIAN_POINT('Ctrl Pts',(-3.65682487407717,1.45232976134301,52.5958225788439));
#22822=CARTESIAN_POINT('Ctrl Pts',(-3.61291046997645,1.55836838693821,52.5900441097309));
#22823=CARTESIAN_POINT('Ctrl Pts',(-3.56445294361742,1.66227681591761,52.5842656406178));
#22824=CARTESIAN_POINT('Ctrl Pts',(-3.51599259796712,1.76619129035884,52.5784868353096));
#22825=CARTESIAN_POINT('Ctrl Pts',(-3.46298878515761,1.86797493726591,52.5727080300014));
#22826=CARTESIAN_POINT('Ctrl Pts',(-3.40566918253362,1.96720777223476,52.5669292246932));
#22827=CARTESIAN_POINT('Ctrl Pts',(-3.34788488095486,2.0672451032674,52.5611035697094));
#22828=CARTESIAN_POINT('Ctrl Pts',(-3.28571470762259,2.16468969157742,52.5552779147256));
#22829=CARTESIAN_POINT('Ctrl Pts',(-3.21943707636124,2.25914008227702,52.5494522597418));
#22830=CARTESIAN_POINT('Ctrl Pts',(-3.15359986645065,2.35296284088024,52.5436653168059));
#22831=CARTESIAN_POINT('Ctrl Pts',(-3.08370993337709,2.44383077506574,52.5378783738701));
#22832=CARTESIAN_POINT('Ctrl Pts',(-3.01008058582062,2.53138378498122,52.5320914309342));
#22833=CARTESIAN_POINT('Ctrl Pts',(-2.93571241738874,2.61981533033913,52.5262464199265));
#22834=CARTESIAN_POINT('Ctrl Pts',(-2.85752968143504,2.70486473577434,52.5204014089187));
#22835=CARTESIAN_POINT('Ctrl Pts',(-2.77589224681784,2.78620014249814,52.514556397911));
#22836=CARTESIAN_POINT('Ctrl Pts',(-2.69425481220065,2.86753554922193,52.5087113869032));
#22837=CARTESIAN_POINT('Ctrl Pts',(-2.60916304801192,2.9451567104361,52.5028663758955));
#22838=CARTESIAN_POINT('Ctrl Pts',(-2.52100877130662,3.01877521107404,52.4970213648877));
#22839=CARTESIAN_POINT('Ctrl Pts',(-2.43236539580103,3.09280216291465,52.4911439245076));
#22840=CARTESIAN_POINT('Ctrl Pts',(-2.3403133601219,3.16304276857767,52.4852664841274));
#22841=CARTESIAN_POINT('Ctrl Pts',(-2.24520969962729,3.2291674476093,52.4793890437472));
#22842=CARTESIAN_POINT('Ctrl Pts',(-2.15022758345157,3.29520761802126,52.4735191148496));
#22843=CARTESIAN_POINT('Ctrl Pts',(-2.05220193435526,3.35714208973021,52.467649185952));
#22844=CARTESIAN_POINT('Ctrl Pts',(-1.95152372976844,3.41468067791861,52.4617792570543));
#22845=CARTESIAN_POINT('Ctrl Pts',(-1.85094740533806,3.47216104059148,52.4559152681641));
#22846=CARTESIAN_POINT('Ctrl Pts',(-1.74772422086267,3.52525416478485,52.4500512792738));
#22847=CARTESIAN_POINT('Ctrl Pts',(-1.64227453274059,3.57371282549559,52.4441872903835));
#22848=CARTESIAN_POINT('Ctrl Pts',(-1.53387209242361,3.62352840265933,52.4381591008552));
#22849=CARTESIAN_POINT('Ctrl Pts',(-1.42311697650877,3.66844587849009,52.432130911327));
#22850=CARTESIAN_POINT('Ctrl Pts',(-1.3104938323533,3.70824687896639,52.4261027217987));
#22851=CARTESIAN_POINT('Ctrl Pts',(-1.2010617303594,3.74692016567174,52.4202453338147));
#22852=CARTESIAN_POINT('Ctrl Pts',(-1.08986645002449,3.78076287615063,52.4143879458307));
#22853=CARTESIAN_POINT('Ctrl Pts',(-0.977372607493188,3.80962357538405,
52.4085305578467));
#22854=CARTESIAN_POINT('Ctrl Pts',(-0.864895013389615,3.83848010602501,
52.4026740158943));
#22855=CARTESIAN_POINT('Ctrl Pts',(-0.751119629522808,3.86235595386983,
52.3968174739419));
#22856=CARTESIAN_POINT('Ctrl Pts',(-0.636524707289445,3.88114999671619,
52.3909609319895));
#22857=CARTESIAN_POINT('Ctrl Pts',(-0.521918728982694,3.89994585280448,
52.3851038250002));
#22858=CARTESIAN_POINT('Ctrl Pts',(-0.406493462208433,3.91365886247838,
52.3792467180109));
#22859=CARTESIAN_POINT('Ctrl Pts',(-0.290735090501276,3.92223942501618,
52.3733896110216));
#22860=CARTESIAN_POINT('Ctrl Pts',(-0.169058159789764,3.93125869937171,
52.3672330385786));
#22861=CARTESIAN_POINT('Ctrl Pts',(-0.0470136672297076,3.93460677047019,
52.3610764661355));
#22862=CARTESIAN_POINT('Ctrl Pts',(0.0748319178295033,3.93228803422053,
52.3549198936924));
#22863=CARTESIAN_POINT('Ctrl Pts',(0.190923453384458,3.93007879823025,52.3490540599134));
#22864=CARTESIAN_POINT('Ctrl Pts',(0.306834022036394,3.922725829333,52.3431882261343));
#22865=CARTESIAN_POINT('Ctrl Pts',(0.422078572658463,3.91028626554407,52.3373223923553));
#22866=CARTESIAN_POINT('Ctrl Pts',(0.537402364764424,3.8978381483833,52.3314525252629));
#22867=CARTESIAN_POINT('Ctrl Pts',(0.652058820325884,3.88029653418258,52.3255826581706));
#22868=CARTESIAN_POINT('Ctrl Pts',(0.765572875668805,3.85776971474973,52.3197127910783));
#22869=CARTESIAN_POINT('Ctrl Pts',(0.879247899326109,3.83521095121848,52.3138346002361));
#22870=CARTESIAN_POINT('Ctrl Pts',(0.991776891409228,3.80765297422279,52.3079564093938));
#22871=CARTESIAN_POINT('Ctrl Pts',(1.10269973352898,3.77525393817093,52.3020782185516));
#22872=CARTESIAN_POINT('Ctrl Pts',(1.1188493639481,3.7705368533201,52.301222392936));
#22873=CARTESIAN_POINT('Ctrl Pts',(1.13496498330523,3.76571723345069,52.3003665673205));
#22874=CARTESIAN_POINT('Ctrl Pts',(1.15104520906026,3.7607956507499,52.2995107417049));
#22875=CARTESIAN_POINT('Ctrl Pts',(1.26147768457721,3.72699621476005,52.2936332781186));
#22876=CARTESIAN_POINT('Ctrl Pts',(1.37060118244447,3.68827312874922,52.2877558145322));
#22877=CARTESIAN_POINT('Ctrl Pts',(1.47794459146711,3.64474536621601,52.2818783509458));
#22878=CARTESIAN_POINT('Ctrl Pts',(1.58515081259428,3.60127323338742,52.2760083989232));
#22879=CARTESIAN_POINT('Ctrl Pts',(1.69058109043122,3.55300878965019,52.2701384469006));
#22880=CARTESIAN_POINT('Ctrl Pts',(1.79377876580033,3.50012096067605,52.264268494878));
#22881=CARTESIAN_POINT('Ctrl Pts',(1.89687200998751,3.44728665169128,52.2584044829701));
#22882=CARTESIAN_POINT('Ctrl Pts',(1.99773678082893,3.38983845113601,52.2525404710621));
#22883=CARTESIAN_POINT('Ctrl Pts',(2.09593634936964,3.3279933622817,52.2466764591542));
#22884=CARTESIAN_POINT('Ctrl Pts',(2.19688511427671,3.26441685753541,52.2406482782945));
#22885=CARTESIAN_POINT('Ctrl Pts',(2.29501682801645,3.19619379818832,52.2346200974348));
#22886=CARTESIAN_POINT('Ctrl Pts',(2.38988380759784,3.12361079300569,52.2285919165752));
#22887=CARTESIAN_POINT('Ctrl Pts',(2.48206333307946,3.05308396686144,52.2227345059818));
#22888=CARTESIAN_POINT('Ctrl Pts',(2.57116026332614,2.97844116882488,52.2168770953884));
#22889=CARTESIAN_POINT('Ctrl Pts',(2.6567939176076,2.89998880676516,52.211019684795));
#22890=CARTESIAN_POINT('Ctrl Pts',(2.74241520037575,2.82154777873584,52.2051631204231));
#22891=CARTESIAN_POINT('Ctrl Pts',(2.82457389804232,2.73929855968457,52.1993065560511));
#22892=CARTESIAN_POINT('Ctrl Pts',(2.90292402008163,2.65358646620626,52.1934499916792));
#22893=CARTESIAN_POINT('Ctrl Pts',(2.98128169842472,2.56786610641517,52.1875928624838));
#22894=CARTESIAN_POINT('Ctrl Pts',(3.05582979263931,2.47868251277184,52.1817357332885));
#22895=CARTESIAN_POINT('Ctrl Pts',(3.12626113059767,2.3864157943062,52.1758786040932));
#22896=CARTESIAN_POINT('Ctrl Pts',(3.2002928563174,2.289432482722,52.1697220636289));
#22897=CARTESIAN_POINT('Ctrl Pts',(3.26977549092988,2.18904289665158,52.1635655231647));
#22898=CARTESIAN_POINT('Ctrl Pts',(3.33440323090798,2.08572387762866,52.1574089827004));
#22899=CARTESIAN_POINT('Ctrl Pts',(3.39597952847646,1.98728313589773,52.1515431274539));
#22900=CARTESIAN_POINT('Ctrl Pts',(3.45314875494368,1.88618366667587,52.1456772722074));
#22901=CARTESIAN_POINT('Ctrl Pts',(3.50569375606319,1.78286294725632,52.1398114169609));
#22902=CARTESIAN_POINT('Ctrl Pts',(3.55827488439563,1.67947118987785,52.1339415286571));
#22903=CARTESIAN_POINT('Ctrl Pts',(3.60622528644685,1.57385551582131,52.1280716403532));
#22904=CARTESIAN_POINT('Ctrl Pts',(3.64937610872275,1.46647298545984,52.1222017520494));
#22905=CARTESIAN_POINT('Ctrl Pts',(3.69258811709727,1.35893819106849,52.1163235404844));
#22906=CARTESIAN_POINT('Ctrl Pts',(3.73098682975768,1.24963192870861,52.1104453289194));
#22907=CARTESIAN_POINT('Ctrl Pts',(3.76445332125774,1.13902598393165,52.1045671173544));
#22908=CARTESIAN_POINT('Ctrl Pts',(3.76932489620612,1.12292554658178,52.1037114510769));
#22909=CARTESIAN_POINT('Ctrl Pts',(3.77409204910857,1.10679758562085,52.1028557847995));
#22910=CARTESIAN_POINT('Ctrl Pts',(3.77875450399893,1.09064357079098,52.102000118522));
#22911=CARTESIAN_POINT('Ctrl Pts',(3.8107804355628,0.979683275069462,52.0961226333157));
#22912=CARTESIAN_POINT('Ctrl Pts',(3.83796732377089,0.867129288955818,52.0902451481093));
#22913=CARTESIAN_POINT('Ctrl Pts',(3.86015742648859,0.753441200575642,52.084367662903));
#22914=CARTESIAN_POINT('Ctrl Pts',(3.88231917084835,0.639898402532647,52.0784976889656));
#22915=CARTESIAN_POINT('Ctrl Pts',(3.89949675111667,0.525224785894342,52.0726277150282));
#22916=CARTESIAN_POINT('Ctrl Pts',(3.91158215895138,0.409895125334751,52.0667577410908));
#22917=CARTESIAN_POINT('Ctrl Pts',(3.92365533751389,0.294682167316825,52.0608937070034));
#22918=CARTESIAN_POINT('Ctrl Pts',(3.93064655066653,0.178814893778597,52.0550296729159));
#22919=CARTESIAN_POINT('Ctrl Pts',(3.93249894675403,0.0627776534951526,
52.0491656388285));
#22920=CARTESIAN_POINT('Ctrl Pts',(3.9344031927486,-0.0565075531206359,
52.0431374661831));
#22921=CARTESIAN_POINT('Ctrl Pts',(3.93087660300224,-0.175971946927321,
52.0371092935377));
#22922=CARTESIAN_POINT('Ctrl Pts',(3.92191463987212,-0.295083983903956,
52.0310811208923));
#22923=CARTESIAN_POINT('Ctrl Pts',(3.91320651152266,-0.410822342888443,
52.0252236876105));
#22924=CARTESIAN_POINT('Ctrl Pts',(3.89936680872289,-0.526227598819512,
52.0193662543286));
#22925=CARTESIAN_POINT('Ctrl Pts',(3.88044418295405,-0.640813500933015,
52.0135088210468));
#22926=CARTESIAN_POINT('Ctrl Pts',(3.86152429045182,-0.755382851758902,
52.0076522338382));
#22927=CARTESIAN_POINT('Ctrl Pts',(3.83752300214969,-0.86913267723255,52.0017956466296));
#22928=CARTESIAN_POINT('Ctrl Pts',(3.80854051076383,-0.981584524058269,
51.995939059421));
#22929=CARTESIAN_POINT('Ctrl Pts',(3.77955522363123,-1.09404721836014,51.9900819072667));
#22930=CARTESIAN_POINT('Ctrl Pts',(3.74558788117118,-1.20521128565554,51.9842247551123));
#22931=CARTESIAN_POINT('Ctrl Pts',(3.70678902513152,-1.31461177659582,51.978367602958));
#22932=CARTESIAN_POINT('Ctrl Pts',(3.66600717434945,-1.42960368492558,51.9722110939898));
#22933=CARTESIAN_POINT('Ctrl Pts',(3.61988704088369,-1.54264649743468,51.9660545850215));
#22934=CARTESIAN_POINT('Ctrl Pts',(3.56866092694071,-1.65322357487626,51.9598980760533));
#22935=CARTESIAN_POINT('Ctrl Pts',(3.51985304709199,-1.75858063389108,51.9540321977565));
#22936=CARTESIAN_POINT('Ctrl Pts',(3.46641049709761,-1.86169909325234,51.9481663194596));
#22937=CARTESIAN_POINT('Ctrl Pts',(3.408581048649,-1.96215805550695,51.9423004411628));
#22938=CARTESIAN_POINT('Ctrl Pts',(3.35071183955772,-2.06268608833042,51.9364305297808));
#22939=CARTESIAN_POINT('Ctrl Pts',(3.28844994683734,-2.16055063593432,51.9305606183988));
#22940=CARTESIAN_POINT('Ctrl Pts',(3.22208593325395,-2.25536055625857,51.9246907070167));
#22941=CARTESIAN_POINT('Ctrl Pts',(3.15562781972929,-2.35030491100672,51.9188124724745));
#22942=CARTESIAN_POINT('Ctrl Pts',(3.08505622921332,-2.44218567024063,51.9129342379323));
#22943=CARTESIAN_POINT('Ctrl Pts',(3.01070133586929,-2.53064546434202,51.9070560033901));
#22944=CARTESIAN_POINT('Ctrl Pts',(2.99987992166008,-2.5435196684432,51.9062005007065));
#22945=CARTESIAN_POINT('Ctrl Pts',(2.98897843458229,-2.55632147826902,51.9053449980228));
#22946=CARTESIAN_POINT('Ctrl Pts',(2.97799795422667,-2.56904986028331,51.9044894953391));
#22947=CARTESIAN_POINT('Ctrl Pts',(2.90256151038189,-2.65649447508698,51.898612149534));
#22948=CARTESIAN_POINT('Ctrl Pts',(2.82314659863413,-2.74075702202623,51.8927348037289));
#22949=CARTESIAN_POINT('Ctrl Pts',(2.74005194549637,-2.82145429450514,51.8868574579238));
#22950=CARTESIAN_POINT('Ctrl Pts',(2.65706349213867,-2.90204843119534,51.8809876237071));
#22951=CARTESIAN_POINT('Ctrl Pts',(2.57040494365269,-2.97908607059595,51.8751177894904));
#22952=CARTESIAN_POINT('Ctrl Pts',(2.48041491919786,-3.05221736261044,51.8692479552737));
#22953=CARTESIAN_POINT('Ctrl Pts',(2.39051596047105,-3.12527464915166,51.8633840610568));
#22954=CARTESIAN_POINT('Ctrl Pts',(2.29729255013922,-3.19443319290352,51.8575201668399));
#22955=CARTESIAN_POINT('Ctrl Pts',(2.20111927658947,-3.25938075870651,51.8516562726229));
#22956=CARTESIAN_POINT('Ctrl Pts',(2.10225082631248,-3.3261484265127,51.8456280476035));
#22957=CARTESIAN_POINT('Ctrl Pts',(2.00026504762229,-3.38846529382579,51.839599822584));
#22958=CARTESIAN_POINT('Ctrl Pts',(1.89560468220114,-3.4460371281832,51.8335715975646));
#22959=CARTESIAN_POINT('Ctrl Pts',(1.79391197486553,-3.50197650579307,51.8277143036388));
#22960=CARTESIAN_POINT('Ctrl Pts',(1.68969470443012,-3.55343611481209,51.821857009713));
#22961=CARTESIAN_POINT('Ctrl Pts',(1.58338669623113,-3.60019104634716,51.8159997157871));
#22962=CARTESIAN_POINT('Ctrl Pts',(1.4770940361507,-3.64693922768301,51.8101432675026));
#22963=CARTESIAN_POINT('Ctrl Pts',(1.36871161605367,-3.68898391617528,51.8042868192181));
#22964=CARTESIAN_POINT('Ctrl Pts',(1.25869489020222,-3.72614763172084,51.7984303709335));
#22965=CARTESIAN_POINT('Ctrl Pts',(1.14866754058109,-3.76331493598211,51.7925733571208));
#22966=CARTESIAN_POINT('Ctrl Pts',(1.0370059623169,-3.79560019830782,51.7867163433081));
#22967=CARTESIAN_POINT('Ctrl Pts',(0.924181807461963,-3.82287548669275,
51.7808593294954));
#22968=CARTESIAN_POINT('Ctrl Pts',(0.805584680066861,-3.85154639369386,
51.7747026247172));
#22969=CARTESIAN_POINT('Ctrl Pts',(0.685703346159854,-3.87468092942088,
51.7685459199389));
#22970=CARTESIAN_POINT('Ctrl Pts',(0.565097510560029,-3.89219138835166,
51.7623892151606));
#22971=CARTESIAN_POINT('Ctrl Pts',(0.450191432651099,-3.9088743137517,51.7565234724675));
#22972=CARTESIAN_POINT('Ctrl Pts',(0.334628190883094,-3.92045260275053,
51.7506577297744));
#22973=CARTESIAN_POINT('Ctrl Pts',(0.218895662112313,-3.92690382987773,
51.7447919870813));
#22974=CARTESIAN_POINT('Ctrl Pts',(0.103083540709917,-3.93335949370177,
51.7389222103461));
#22975=CARTESIAN_POINT('Ctrl Pts',(-0.0128976881731574,-3.93468106983234,
51.7330524336109));
#22976=CARTESIAN_POINT('Ctrl Pts',(-0.128561691980987,-3.93089822958506,
51.7271826568757));
#22977=CARTESIAN_POINT('Ctrl Pts',(-0.244389746367142,-3.92711002399412,
51.7213045548168));
#22978=CARTESIAN_POINT('Ctrl Pts',(-0.359899268433259,-3.91820298742322,
51.7154264527579));
#22979=CARTESIAN_POINT('Ctrl Pts',(-0.47461057168177,-3.90425841937338,
51.709548350699));
#22980=CARTESIAN_POINT('Ctrl Pts',(-0.491325050230513,-3.90222656918129,
51.7086918578514));
#22981=CARTESIAN_POINT('Ctrl Pts',(-0.508022602959161,-3.90008785421182,
51.7078353650038));
#22982=CARTESIAN_POINT('Ctrl Pts',(-0.524701769303992,-3.89784261525389,
51.7069788721562));
#22983=CARTESIAN_POINT('Ctrl Pts',(-0.63916023950688,-3.88243497370565,
51.7011013085509));
#22984=CARTESIAN_POINT('Ctrl Pts',(-0.753127073525721,-3.8619562765558,
51.6952237449456));
#22985=CARTESIAN_POINT('Ctrl Pts',(-0.866118077357017,-3.83644737694594,
51.6893461813402));
#22986=CARTESIAN_POINT('Ctrl Pts',(-0.978964668335136,-3.81097108004647,
51.6834761297996));
#22987=CARTESIAN_POINT('Ctrl Pts',(-1.09083751071811,-3.78047745655816,
51.677606078259));
#22988=CARTESIAN_POINT('Ctrl Pts',(-1.20125855487867,-3.74505899610818,
51.6717360267183));
#22989=CARTESIAN_POINT('Ctrl Pts',(-1.31156784853888,-3.70967638055269,
51.665871915904));
#22990=CARTESIAN_POINT('Ctrl Pts',(-1.4204278761091,-3.66937896757605,51.6600078050896));
#22991=CARTESIAN_POINT('Ctrl Pts',(-1.52737244212953,-3.62430992369904,
51.6541436942752));
#22992=CARTESIAN_POINT('Ctrl Pts',(-1.63730849496429,-3.57798019444538,
51.648115550721));
#22993=CARTESIAN_POINT('Ctrl Pts',(-1.74521990979877,-3.52660803868946,
51.6420874071667));
#22994=CARTESIAN_POINT('Ctrl Pts',(-1.85061840581349,-3.47040350911308,
51.6360592636125));
#22995=CARTESIAN_POINT('Ctrl Pts',(-1.95303343001351,-3.41578993800566,
51.6302017562349));
#22996=CARTESIAN_POINT('Ctrl Pts',(-2.05307550368128,-3.35661410648841,
51.6243442488574));
#22997=CARTESIAN_POINT('Ctrl Pts',(-2.15031920814855,-3.29311650311182,
51.6184867414798));
#22998=CARTESIAN_POINT('Ctrl Pts',(-2.2475488482417,-3.2296280834048,51.6126300812746));
#22999=CARTESIAN_POINT('Ctrl Pts',(-2.3419805786639,-3.1618193602502,51.6067734210694));
#23000=CARTESIAN_POINT('Ctrl Pts',(-2.43321688783559,-3.08997485050473,
51.6009167608641));
#23001=CARTESIAN_POINT('Ctrl Pts',(-2.52446197956638,-3.01812342488707,
51.595059536887));
#23002=CARTESIAN_POINT('Ctrl Pts',(-2.61251071449089,-2.94223569559399,
51.5892023129099));
#23003=CARTESIAN_POINT('Ctrl Pts',(-2.69699823013746,-2.86263681710333,
51.5833450889329));
#23004=CARTESIAN_POINT('Ctrl Pts',(-2.78580125776636,-2.77897213183307,
51.5771886856029));
#23005=CARTESIAN_POINT('Ctrl Pts',(-2.87066927267329,-2.69120750080115,
51.5710322822729));
#23006=CARTESIAN_POINT('Ctrl Pts',(-2.95122308578683,-2.59976370040027,
51.564875878943));
#23007=CARTESIAN_POINT('Ctrl Pts',(-3.02797640016931,-2.51263418425181,
51.5590099324162));
#23008=CARTESIAN_POINT('Ctrl Pts',(-3.10081308566887,-2.42216510162187,
51.5531439858895));
#23009=CARTESIAN_POINT('Ctrl Pts',(-3.16944777765645,-2.32875283890512,
51.5472780393627));
#23010=CARTESIAN_POINT('Ctrl Pts',(-3.23812964437753,-2.2352763710689,51.5414080609906));
#23011=CARTESIAN_POINT('Ctrl Pts',(-3.30260353793884,-2.13885303694543,
51.5355380826185));
#23012=CARTESIAN_POINT('Ctrl Pts',(-3.36262857005296,-2.03990639487788,
51.5296681042464));
#23013=CARTESIAN_POINT('Ctrl Pts',(-3.42273869087957,-1.94081949062167,
51.5237898048642));
#23014=CARTESIAN_POINT('Ctrl Pts',(-3.4783871690931,-1.83920250123322,51.5179115054819));
#23015=CARTESIAN_POINT('Ctrl Pts',(-3.52937998787692,-1.73550162811044,
51.5120332060996));
#23016=CARTESIAN_POINT('Ctrl Pts',(-3.53679678114902,-1.72041856432947,
51.5111782203909));
#23017=CARTESIAN_POINT('Ctrl Pts',(-3.54411516846418,-1.70529144587849,
51.5103232346821));
#23018=CARTESIAN_POINT('Ctrl Pts',(-3.55133463990173,-1.69012167474241,
51.5094682489733));
#23019=CARTESIAN_POINT('Ctrl Pts',(-3.60486774011933,-1.57763630991621,
51.5031284447331));
#23020=CARTESIAN_POINT('Ctrl Pts',(-3.65311231872581,-1.46248026746492,
51.4967886404929));
#23021=CARTESIAN_POINT('Ctrl Pts',(-3.69581538181708,-1.3451533977671,51.4904488362527));
#23022=CARTESIAN_POINT('Ctrl Pts',(-3.73837808187887,-1.22821217616282,
51.4841298706612));
#23023=CARTESIAN_POINT('Ctrl Pts',(-3.77543548111521,-1.10911464538009,
51.4778109050697));
#23024=CARTESIAN_POINT('Ctrl Pts',(-3.8067824973443,-0.988380502596623,
51.4714919394781));
#23025=CARTESIAN_POINT('Ctrl Pts',(-3.83806546245479,-0.867893054964066,
51.4651858853807));
#23026=CARTESIAN_POINT('Ctrl Pts',(-3.86366121578873,-0.745775955930149,
51.4588798312833));
#23027=CARTESIAN_POINT('Ctrl Pts',(-3.88341347034862,-0.622566316399284,
51.4525737771858));
#23028=CARTESIAN_POINT('Ctrl Pts',(-3.90310460269884,-0.499737941973974,
51.4462872368082));
#23029=CARTESIAN_POINT('Ctrl Pts',(-3.91698823758152,-0.375824071597219,
51.4400006964305));
#23030=CARTESIAN_POINT('Ctrl Pts',(-3.92495867402245,-0.251373043932732,
51.4337141560528));
#23031=CARTESIAN_POINT('Ctrl Pts',(-3.93028997762093,-0.168129646091341,
51.4295091848965));
#23032=CARTESIAN_POINT('Ctrl Pts',(-3.93297669174091,-0.0846462499726585,
51.4253042137402));
#23033=CARTESIAN_POINT('Ctrl Pts',(-3.93299984895417,-0.00109001217197362,
51.4210992425839));
#23034=CARTESIAN_POINT('',(-3.93427805355045,0.00340288565414877,50.1711036262703));
#23035=CARTESIAN_POINT('Ctrl Pts',(-3.92704610517626,-0.00108733974936265,
51.421099191055));
#23036=CARTESIAN_POINT('Ctrl Pts',(-3.92524730607414,0.72072979241773,51.3847186693002));
#23037=CARTESIAN_POINT('Ctrl Pts',(-3.3898856313511,2.75129080723824,51.2825012731509));
#23038=CARTESIAN_POINT('Ctrl Pts',(-0.136318537846259,4.63920340706317,
51.1144470026077));
#23039=CARTESIAN_POINT('Ctrl Pts',(3.81089992892979,2.6488745889284,50.9169363794247));
#23040=CARTESIAN_POINT('Ctrl Pts',(4.30110806150455,-1.74478063138574,50.719425756242));
#23041=CARTESIAN_POINT('Ctrl Pts',(0.887676967041259,-4.55539414744317,
50.5219151330588));
#23042=CARTESIAN_POINT('Ctrl Pts',(-3.01408004080397,-3.33156985104081,
50.3391410897352));
#23043=CARTESIAN_POINT('Ctrl Pts',(-3.92504487197984,-1.00631924839508,
50.2222039208056));
#23044=CARTESIAN_POINT('Ctrl Pts',(-3.93427805355045,0.00340288565414877,
50.1711036262703));
#23045=CARTESIAN_POINT('',(-3.89317704633887,0.578984810677012,50.1436634243168));
#23046=CARTESIAN_POINT('Ctrl Pts',(-3.93299849268476,0.00344333260814783,
50.1718402566183));
#23047=CARTESIAN_POINT('Ctrl Pts',(-3.93291481497374,0.099020597068333,
50.167553787606));
#23048=CARTESIAN_POINT('Ctrl Pts',(-3.92934717672993,0.194561546255428,
50.1632628550717));
#23049=CARTESIAN_POINT('Ctrl Pts',(-3.91516728110938,0.386429387633131,
50.1544929579965));
#23050=CARTESIAN_POINT('Ctrl Pts',(-3.90446908640162,0.482681821527946,
50.1500151960044));
#23051=CARTESIAN_POINT('Ctrl Pts',(-3.89023144643595,0.578436075258949,
50.1454016210458));
#23052=CARTESIAN_POINT('',(-2.81006454498411,-2.75173150089599,50.1419356690201));
#23053=CARTESIAN_POINT('Origin',(-1.041818884589E-14,0.,50.1419356690201));
#23054=CARTESIAN_POINT('',(-3.9296784706345,-0.000991769389231509,51.2377721674176));
#23055=CARTESIAN_POINT('Ctrl Pts',(-2.8100645449841,-2.751731500896,50.1419356690201));
#23056=CARTESIAN_POINT('Ctrl Pts',(-1.89942791543654,-3.68167241454335,
50.2077725434144));
#23057=CARTESIAN_POINT('Ctrl Pts',(0.902301753494953,-4.550726992117,50.3394462922028));
#23058=CARTESIAN_POINT('Ctrl Pts',(4.31098005768057,-1.72664187782764,50.5369569153859));
#23059=CARTESIAN_POINT('Ctrl Pts',(3.79825323790283,2.66550893609982,50.7344675385685));
#23060=CARTESIAN_POINT('Ctrl Pts',(-0.155736620608226,4.63846238854458,
50.9319781617517));
#23061=CARTESIAN_POINT('Ctrl Pts',(-3.39636166881464,2.73991008102441,51.0997463645569));
#23062=CARTESIAN_POINT('Ctrl Pts',(-3.92545006867067,0.715178458449969,
51.2016776929682));
#23063=CARTESIAN_POINT('Ctrl Pts',(-3.92705168969078,-0.00099070069027788,
51.2377721469851));
#23064=CARTESIAN_POINT('',(-3.93299916752078,-0.0025589609114662,52.4877721469424));
#23065=CARTESIAN_POINT('Ctrl Pts',(-3.9329998746137,-0.000993120693749547,
51.2377721932532));
#23066=CARTESIAN_POINT('Ctrl Pts',(-3.93296843644496,-0.125495927339958,
51.2440375667306));
#23067=CARTESIAN_POINT('Ctrl Pts',(-3.9270208887338,-0.249841356608365,
51.250302940208));
#23068=CARTESIAN_POINT('Ctrl Pts',(-3.91522722570074,-0.373476600514333,
51.2565683136855));
#23069=CARTESIAN_POINT('Ctrl Pts',(-3.90339148758525,-0.497552925623416,
51.2628560395147));
#23070=CARTESIAN_POINT('Ctrl Pts',(-3.88566793179864,-0.62091367922872,
51.269143765344));
#23071=CARTESIAN_POINT('Ctrl Pts',(-3.86217818230335,-0.74301324896671,
51.2754314911733));
#23072=CARTESIAN_POINT('Ctrl Pts',(-3.83864586316443,-0.865334095443862,
51.2817306120261));
#23073=CARTESIAN_POINT('Ctrl Pts',(-3.80932655851785,-0.986388887489586,
51.2880297328789));
#23074=CARTESIAN_POINT('Ctrl Pts',(-3.7743919075506,-1.10564674657713,51.2943288537316));
#23075=CARTESIAN_POINT('Ctrl Pts',(-3.73935297989382,-1.22526057930121,
51.3006467768753));
#23076=CARTESIAN_POINT('Ctrl Pts',(-3.698665276834,-1.34306644872994,51.306964700019));
#23077=CARTESIAN_POINT('Ctrl Pts',(-3.65254956116948,-1.45855089153609,
51.3132826231626));
#23078=CARTESIAN_POINT('Ctrl Pts',(-3.6191757588183,-1.54212662950981,51.3178548848142));
#23079=CARTESIAN_POINT('Ctrl Pts',(-3.58296010671762,-1.62448700139721,
51.3224271464657));
#23080=CARTESIAN_POINT('Ctrl Pts',(-3.54400104932148,-1.70544585443465,
51.3269994081173));
#23081=CARTESIAN_POINT('Ctrl Pts',(-3.49391243270941,-1.80953248337725,
51.3328778424589));
#23082=CARTESIAN_POINT('Ctrl Pts',(-3.43915265248908,-1.9115805427375,51.3387562768005));
#23083=CARTESIAN_POINT('Ctrl Pts',(-3.37991065530951,-2.01114220335742,
51.3446347111421));
#23084=CARTESIAN_POINT('Ctrl Pts',(-3.32074416718912,-2.11057696401308,
51.3505056529098));
#23085=CARTESIAN_POINT('Ctrl Pts',(-3.25710703292163,-2.20753127739272,
51.3563765946774));
#23086=CARTESIAN_POINT('Ctrl Pts',(-3.18923538862743,-2.30157916134261,
51.3622475364451));
#23087=CARTESIAN_POINT('Ctrl Pts',(-3.12143221147759,-2.39553217224034,
51.3681125557598));
#23088=CARTESIAN_POINT('Ctrl Pts',(-3.04940326135557,-2.48658425342008,
51.3739775750745));
#23089=CARTESIAN_POINT('Ctrl Pts',(-2.97342918260808,-2.57433639915508,
51.3798425943892));
#23090=CARTESIAN_POINT('Ctrl Pts',(-2.8953463533348,-2.66452420961294,51.3858704042605));
#23091=CARTESIAN_POINT('Ctrl Pts',(-2.81309640538219,-2.75122582878452,
51.3918982141318));
#23092=CARTESIAN_POINT('Ctrl Pts',(-2.72703019679274,-2.83404222018314,
51.3979260240031));
#23093=CARTESIAN_POINT('Ctrl Pts',(-2.64338206200348,-2.9145318430445,51.4037844794975));
#23094=CARTESIAN_POINT('Ctrl Pts',(-2.55612956890415,-2.99135134332138,
51.409642934992));
#23095=CARTESIAN_POINT('Ctrl Pts',(-2.46563325223476,-3.06417063256508,
51.4155013904864));
#23096=CARTESIAN_POINT('Ctrl Pts',(-2.37514981975917,-3.13697955433893,
51.4213590118975));
#23097=CARTESIAN_POINT('Ctrl Pts',(-2.28142380325412,-3.205789139162,51.4272166333085));
#23098=CARTESIAN_POINT('Ctrl Pts',(-2.18484895451548,-3.2703094725045,51.4330742547196));
#23099=CARTESIAN_POINT('Ctrl Pts',(-2.08826461186527,-3.33483614859925,
51.4389324519714));
#23100=CARTESIAN_POINT('Ctrl Pts',(-1.9888312231127,-3.39507250590266,51.4447906492233));
#23101=CARTESIAN_POINT('Ctrl Pts',(-1.88697106577822,-3.45077226094622,
51.4506488464751));
#23102=CARTESIAN_POINT('Ctrl Pts',(-1.77994849575477,-3.50929495608463,
51.4568039452106));
#23103=CARTESIAN_POINT('Ctrl Pts',(-1.6702471638846,-3.56280889739079,51.462959043946));
#23104=CARTESIAN_POINT('Ctrl Pts',(-1.55838412777636,-3.61108403534101,
51.4691141426814));
#23105=CARTESIAN_POINT('Ctrl Pts',(-1.45175807705138,-3.65709912206596,
51.4749810840126));
#23106=CARTESIAN_POINT('Ctrl Pts',(-1.34316855712051,-3.69835472153699,
51.4808480253438));
#23107=CARTESIAN_POINT('Ctrl Pts',(-1.2330809491863,-3.73470217992731,51.486714966675));
#23108=CARTESIAN_POINT('Ctrl Pts',(-1.12291755025563,-3.77107466211589,
51.492585947165));
#23109=CARTESIAN_POINT('Ctrl Pts',(-1.01125440538746,-3.80253216316647,
51.4984569276551));
#23110=CARTESIAN_POINT('Ctrl Pts',(-0.898568962357412,-3.82897673274309,
51.5043279081451));
#23111=CARTESIAN_POINT('Ctrl Pts',(-0.785723724867012,-3.85545880224527,
51.5102072140242));
#23112=CARTESIAN_POINT('Ctrl Pts',(-0.671853699931724,-3.87691367975029,
51.5160865199033));
#23113=CARTESIAN_POINT('Ctrl Pts',(-0.557443355508977,-3.89329499336987,
51.5219658257824));
#23114=CARTESIAN_POINT('Ctrl Pts',(-0.540940079127791,-3.89565793832485,
51.5228138942883));
#23115=CARTESIAN_POINT('Ctrl Pts',(-0.524425562563187,-3.89791540605198,
51.5236619627942));
#23116=CARTESIAN_POINT('Ctrl Pts',(-0.507901260517054,-3.90006734679867,
51.5245100313001));
#23117=CARTESIAN_POINT('Ctrl Pts',(-0.393396833325279,-3.91497912593838,
51.5303866848625));
#23118=CARTESIAN_POINT('Ctrl Pts',(-0.27804693711552,-3.9248684390782,51.5362633384249));
#23119=CARTESIAN_POINT('Ctrl Pts',(-0.162329551315805,-3.92964859965489,
51.5421399919873));
#23120=CARTESIAN_POINT('Ctrl Pts',(-0.0467602864631677,-3.93442264151478,
51.5480091232964));
#23121=CARTESIAN_POINT('Ctrl Pts',(0.0691751238794702,-3.93410051996893,
51.5538782546055));
#23122=CARTESIAN_POINT('Ctrl Pts',(0.184991176837534,-3.92864700176693,
51.5597473859146));
#23123=CARTESIAN_POINT('Ctrl Pts',(0.300689823238378,-3.9231990119764,51.5656105674915));
#23124=CARTESIAN_POINT('Ctrl Pts',(0.416268943145369,-3.91262999213387,
51.5714737490684));
#23125=CARTESIAN_POINT('Ctrl Pts',(0.531241274755709,-3.89695672390597,
51.5773369306452));
#23126=CARTESIAN_POINT('Ctrl Pts',(0.649455143636631,-3.88084156255125,
51.5833654191385));
#23127=CARTESIAN_POINT('Ctrl Pts',(0.767027055499234,-3.85933002829415,
51.5893939076317));
#23128=CARTESIAN_POINT('Ctrl Pts',(0.883430671087542,-3.83249778204525,
51.595422396125));
#23129=CARTESIAN_POINT('Ctrl Pts',(0.99651456511733,-3.8064307662051,51.6012789578003));
#23130=CARTESIAN_POINT('Ctrl Pts',(1.10849547073079,-3.77534251790644,51.6071355194757));
#23131=CARTESIAN_POINT('Ctrl Pts',(1.21890014683637,-3.73935441380491,51.6129920811511));
#23132=CARTESIAN_POINT('Ctrl Pts',(1.32928876797764,-3.7033715430662,51.6188477911697));
#23133=CARTESIAN_POINT('Ctrl Pts',(1.43810122319181,-3.66249036125565,51.6247035011883));
#23134=CARTESIAN_POINT('Ctrl Pts',(1.5448797500048,-3.61688202157951,51.6305592112069));
#23135=CARTESIAN_POINT('Ctrl Pts',(1.65166849401177,-3.57126931783067,51.6364154815341));
#23136=CARTESIAN_POINT('Ctrl Pts',(1.75642254325717,-3.52092871914075,51.6422717518613));
#23137=CARTESIAN_POINT('Ctrl Pts',(1.85870507712417,-3.46607911569727,51.6481280221885));
#23138=CARTESIAN_POINT('Ctrl Pts',(1.96625256103048,-3.40840615218548,51.6542857415464));
#23139=CARTESIAN_POINT('Ctrl Pts',(2.07106686250261,-3.34574786066241,51.6604434609043));
#23140=CARTESIAN_POINT('Ctrl Pts',(2.17267192079167,-3.27841207364227,51.6666011802621));
#23141=CARTESIAN_POINT('Ctrl Pts',(2.26944686453354,-3.21427730407056,51.672466173152));
#23142=CARTESIAN_POINT('Ctrl Pts',(2.36331036165917,-3.14589982114848,51.6783311660418));
#23143=CARTESIAN_POINT('Ctrl Pts',(2.45388381829003,-3.07358800204814,51.6841961589316));
#23144=CARTESIAN_POINT('Ctrl Pts',(2.54451954056608,-3.00122647145132,51.6900651837706));
#23145=CARTESIAN_POINT('Ctrl Pts',(2.63186040877973,-2.92492548975659,51.6959342086095));
#23146=CARTESIAN_POINT('Ctrl Pts',(2.71556370249527,-2.84503124371071,51.7018032334484));
#23147=CARTESIAN_POINT('Ctrl Pts',(2.7993857529864,-2.76502364509976,51.7076805851576));
#23148=CARTESIAN_POINT('Ctrl Pts',(2.87955964664603,-2.6814129060543,51.7135579368667));
#23149=CARTESIAN_POINT('Ctrl Pts',(2.95578202819155,-2.59457927260274,51.7194352885759));
#23150=CARTESIAN_POINT('Ctrl Pts',(2.9669584194391,-2.58184696693054,51.7202970772116));
#23151=CARTESIAN_POINT('Ctrl Pts',(2.97804992849274,-2.56904542094171,51.7211588658473));
#23152=CARTESIAN_POINT('Ctrl Pts',(2.98905567748977,-2.55617588535415,51.722020654483));
#23153=CARTESIAN_POINT('Ctrl Pts',(3.06411804358784,-2.46840195992251,51.727898300256));
#23154=CARTESIAN_POINT('Ctrl Pts',(3.13543388295215,-2.37717510774856,51.733775946029));
#23155=CARTESIAN_POINT('Ctrl Pts',(3.20266945456006,-2.282848519904,51.739653591802));
#23156=CARTESIAN_POINT('Ctrl Pts',(3.26981911428937,-2.1886424601396,51.7455237272709));
#23157=CARTESIAN_POINT('Ctrl Pts',(3.33289863769181,-2.09134487460477,51.7513938627398));
#23158=CARTESIAN_POINT('Ctrl Pts',(3.39161328128917,-1.9913433531621,51.7572639982087));
#23159=CARTESIAN_POINT('Ctrl Pts',(3.45026852051612,-1.89144300796878,51.7631281945851));
#23160=CARTESIAN_POINT('Ctrl Pts',(3.5045674567879,-1.78884452228466,51.7689923909614));
#23161=CARTESIAN_POINT('Ctrl Pts',(3.55425796100606,-1.68396536384363,51.7748565873378));
#23162=CARTESIAN_POINT('Ctrl Pts',(3.60533741168598,-1.57615462846809,51.7808846994348));
#23163=CARTESIAN_POINT('Ctrl Pts',(3.65154673786758,-1.46593419950273,51.7869128115318));
#23164=CARTESIAN_POINT('Ctrl Pts',(3.69266193913359,-1.35378609952757,51.7929409236288));
#23165=CARTESIAN_POINT('Ctrl Pts',(3.73261412492424,-1.24481030497198,51.7987985200177));
#23166=CARTESIAN_POINT('Ctrl Pts',(3.76775636436242,-1.13401484549651,51.8046561164067));
#23167=CARTESIAN_POINT('Ctrl Pts',(3.79793179280356,-1.02186256278029,51.8105137127956));
#23168=CARTESIAN_POINT('Ctrl Pts',(3.82810286277188,-0.909726479094201,
51.8163704631261));
#23169=CARTESIAN_POINT('Ctrl Pts',(3.85330844116812,-0.796234360075338,
51.8222272134567));
#23170=CARTESIAN_POINT('Ctrl Pts',(3.87344181331822,-0.681863269899464,
51.8280839637872));
#23171=CARTESIAN_POINT('Ctrl Pts',(3.89357712697097,-0.567481150683174,
51.8339412788963));
#23172=CARTESIAN_POINT('Ctrl Pts',(3.90863919053139,-0.452220298051512,
51.8397985940054));
#23173=CARTESIAN_POINT('Ctrl Pts',(3.91857271447358,-0.336566310529017,
51.8456559091144));
#23174=CARTESIAN_POINT('Ctrl Pts',(3.92901325945277,-0.215009180775335,
51.851812189827));
#23175=CARTESIAN_POINT('Ctrl Pts',(3.9337878535178,-0.0930182296759476,
51.8579684705397));
#23176=CARTESIAN_POINT('Ctrl Pts',(3.93289425801458,0.0288401677507168,
51.8641247512523));
#23177=CARTESIAN_POINT('Ctrl Pts',(3.93204279158699,0.144953480713162,51.8699907905582));
#23178=CARTESIAN_POINT('Ctrl Pts',(3.9260454836577,0.260946036023648,51.8758568298642));
#23179=CARTESIAN_POINT('Ctrl Pts',(3.91495378487565,0.376332117002756,51.8817228691702));
#23180=CARTESIAN_POINT('Ctrl Pts',(3.90385446151273,0.491797515904352,51.8875929408694));
#23181=CARTESIAN_POINT('Ctrl Pts',(3.88765383153072,0.606655203033215,51.8934630125686));
#23182=CARTESIAN_POINT('Ctrl Pts',(3.86645461305077,0.720428848130284,51.8993330842678));
#23183=CARTESIAN_POINT('Ctrl Pts',(3.84522534329854,0.834363774776051,51.9052114771758));
#23184=CARTESIAN_POINT('Ctrl Pts',(3.81898343906944,0.947211193118578,51.9110898700838));
#23185=CARTESIAN_POINT('Ctrl Pts',(3.78788165308817,1.05850913184438,51.9169682629918));
#23186=CARTESIAN_POINT('Ctrl Pts',(3.78336146448637,1.07468465547299,51.9178226012165));
#23187=CARTESIAN_POINT('Ctrl Pts',(3.77873870681719,1.09082748452661,51.9186769394411));
#23188=CARTESIAN_POINT('Ctrl Pts',(3.77401393306265,1.10693623711978,51.9195312776658));
#23189=CARTESIAN_POINT('Ctrl Pts',(3.74150913385129,1.21775884911978,51.9254088273422));
#23190=CARTESIAN_POINT('Ctrl Pts',(3.70406554225549,1.32733009494124,51.9312863770185));
#23191=CARTESIAN_POINT('Ctrl Pts',(3.66179663040747,1.43517749339113,51.9371639266948));
#23192=CARTESIAN_POINT('Ctrl Pts',(3.61958172310896,1.54288710144343,51.9430339669651));
#23193=CARTESIAN_POINT('Ctrl Pts',(3.57255390550052,1.64887686165038,51.9489040072354));
#23194=CARTESIAN_POINT('Ctrl Pts',(3.5208767670674,1.75268816140378,51.9547740475057));
#23195=CARTESIAN_POINT('Ctrl Pts',(3.46925190475028,1.85639444660502,51.9606381496975));
#23196=CARTESIAN_POINT('Ctrl Pts',(3.41298725985111,1.95792628777203,51.9665022518893));
#23197=CARTESIAN_POINT('Ctrl Pts',(3.35229472869644,2.05684444038775,51.972366354081));
#23198=CARTESIAN_POINT('Ctrl Pts',(3.28990435160217,2.15852978330803,51.978394501863));
#23199=CARTESIAN_POINT('Ctrl Pts',(3.22283485144771,2.25745262942961,51.984422649645));
#23200=CARTESIAN_POINT('Ctrl Pts',(3.15136757940517,2.35316199601174,51.990450797427));
#23201=CARTESIAN_POINT('Ctrl Pts',(3.08192337454572,2.44616205981633,51.9963083027932));
#23202=CARTESIAN_POINT('Ctrl Pts',(3.00832730189277,2.53612778339065,52.0021658081594));
#23203=CARTESIAN_POINT('Ctrl Pts',(2.93088130962389,2.62267492245938,52.0080233135255));
#23204=CARTESIAN_POINT('Ctrl Pts',(2.85344648590253,2.70920958049703,52.0138799741763));
#23205=CARTESIAN_POINT('Ctrl Pts',(2.77216312158727,2.79232632706189,52.019736634827));
#23206=CARTESIAN_POINT('Ctrl Pts',(2.68737247604201,2.87167515137276,52.0255932954777));
#23207=CARTESIAN_POINT('Ctrl Pts',(2.6025736328453,2.95103164721391,52.0314505223567));
#23208=CARTESIAN_POINT('Ctrl Pts',(2.51426713552821,3.02661921477329,52.0373077492357));
#23209=CARTESIAN_POINT('Ctrl Pts',(2.42282948697284,3.0981262526009,52.0431649761148));
#23210=CARTESIAN_POINT('Ctrl Pts',(2.326721260052,3.17328582556181,52.0493213865093));
#23211=CARTESIAN_POINT('Ctrl Pts',(2.22715395030478,3.24393667225648,52.0554777969038));
#23212=CARTESIAN_POINT('Ctrl Pts',(2.12460074935781,3.30976746250068,52.0616342072983));
#23213=CARTESIAN_POINT('Ctrl Pts',(2.02688593127163,3.37249240559151,52.0675001628824));
#23214=CARTESIAN_POINT('Ctrl Pts',(1.92646092773579,3.43084156162493,52.0733661184665));
#23215=CARTESIAN_POINT('Ctrl Pts',(1.8237606571654,3.48459266850167,52.0792320740506));
#23216=CARTESIAN_POINT('Ctrl Pts',(1.72098976059647,3.53838073950298,52.0851020635965));
#23217=CARTESIAN_POINT('Ctrl Pts',(1.61594085388379,3.58756429057839,52.0909720531424));
#23218=CARTESIAN_POINT('Ctrl Pts',(1.50906900213238,3.631969128008,52.0968420426884));
#23219=CARTESIAN_POINT('Ctrl Pts',(1.40204560072971,3.67643693372641,52.1027203561742));
#23220=CARTESIAN_POINT('Ctrl Pts',(1.29319448196287,3.71611236350754,52.10859866966));
#23221=CARTESIAN_POINT('Ctrl Pts',(1.18298601924968,3.75087097595475,52.1144769831458));
#23222=CARTESIAN_POINT('Ctrl Pts',(1.16695672571622,3.75592644980872,52.1153319557134));
#23223=CARTESIAN_POINT('Ctrl Pts',(1.15089873538002,3.76087800014745,52.1161869282811));
#23224=CARTESIAN_POINT('Ctrl Pts',(1.13481351104836,3.76572533453279,52.1170419008488));
#23225=CARTESIAN_POINT('Ctrl Pts',(1.02423857216309,3.79904745005716,52.1229192537206));
#23226=CARTESIAN_POINT('Ctrl Pts',(0.912013391930761,3.82754978012318,52.1287966065924));
#23227=CARTESIAN_POINT('Ctrl Pts',(0.798595653982026,3.8510691997731,52.1346739594642));
#23228=CARTESIAN_POINT('Ctrl Pts',(0.685322895731775,3.87455855500425,52.1405437994297));
#23229=CARTESIAN_POINT('Ctrl Pts',(0.570861011804716,3.89307758428636,52.1464136393951));
#23230=CARTESIAN_POINT('Ctrl Pts',(0.455683456048091,3.90651271441474,52.1522834793605));
#23231=CARTESIAN_POINT('Ctrl Pts',(0.340622480277015,3.91993424582361,52.1581473780134));
#23232=CARTESIAN_POINT('Ctrl Pts',(0.22484768097639,3.92828206641365,52.1640112766663));
#23233=CARTESIAN_POINT('Ctrl Pts',(0.108842686602906,3.93149364358803,52.1698751753191));
#23234=CARTESIAN_POINT('Ctrl Pts',(-0.010413119253216,3.93479521888716,
52.1759033981821));
#23235=CARTESIAN_POINT('Ctrl Pts',(-0.129911778455284,3.93266833168623,
52.1819316210452));
#23236=CARTESIAN_POINT('Ctrl Pts',(-0.249121807255898,3.92510220569472,
52.1879598439082));
#23237=CARTESIAN_POINT('Ctrl Pts',(-0.364951684713297,3.91775061409424,
52.1938171389909));
#23238=CARTESIAN_POINT('Ctrl Pts',(-0.48050864107356,3.905264121684,52.1996744340737));
#23239=CARTESIAN_POINT('Ctrl Pts',(-0.595305907292519,3.88768567103137,
52.2055317291565));
#23240=CARTESIAN_POINT('Ctrl Pts',(-0.710086575880422,3.87010976190824,
52.2113881773791));
#23241=CARTESIAN_POINT('Ctrl Pts',(-0.824107365082178,3.84744342093164,
52.2172446256018));
#23242=CARTESIAN_POINT('Ctrl Pts',(-0.936888698124418,3.81978121982487,
52.2231010738245));
#23243=CARTESIAN_POINT('Ctrl Pts',(-1.04968089843017,3.79211635327319,52.2289580863565));
#23244=CARTESIAN_POINT('Ctrl Pts',(-1.1612330045025,3.7594547679124,52.2348150988886));
#23245=CARTESIAN_POINT('Ctrl Pts',(-1.27107835219798,3.72194153938152,52.2406721114207));
#23246=CARTESIAN_POINT('Ctrl Pts',(-1.38654420853534,3.68250885381795,52.2468288124716));
#23247=CARTESIAN_POINT('Ctrl Pts',(-1.50012353867866,3.63771504765641,52.2529855135225));
#23248=CARTESIAN_POINT('Ctrl Pts',(-1.61129695160193,3.58778638351817,52.2591422145734));
#23249=CARTESIAN_POINT('Ctrl Pts',(-1.71721636315969,3.54021732373732,52.2650079529303));
#23250=CARTESIAN_POINT('Ctrl Pts',(-1.82095171208986,3.4879878901259,52.2708736912872));
#23251=CARTESIAN_POINT('Ctrl Pts',(-1.9220792453382,3.43134090038285,52.276739429644));
#23252=CARTESIAN_POINT('Ctrl Pts',(-2.02327630887592,3.37465496297181,52.2826092009924));
#23253=CARTESIAN_POINT('Ctrl Pts',(-2.12186163679519,3.3135456382147,52.2884789723409));
#23254=CARTESIAN_POINT('Ctrl Pts',(-2.21744072864956,3.24829888017192,52.2943487436893));
#23255=CARTESIAN_POINT('Ctrl Pts',(-2.31315536032801,3.18295959630644,52.300226838906));
#23256=CARTESIAN_POINT('Ctrl Pts',(-2.40585492077329,3.11347141802519,52.3061049341228));
#23257=CARTESIAN_POINT('Ctrl Pts',(-2.49517821624012,3.04016030320784,52.3119830293395));
#23258=CARTESIAN_POINT('Ctrl Pts',(-2.50819352846376,3.02947812848709,52.3128395275702));
#23259=CARTESIAN_POINT('Ctrl Pts',(-2.52113722270169,3.01871484990376,52.3136960258009));
#23260=CARTESIAN_POINT('Ctrl Pts',(-2.53400824918214,3.00787153865935,52.3145525240316));
#23261=CARTESIAN_POINT('Ctrl Pts',(-2.62112209425453,2.93448170162867,52.3203494862463));
#23262=CARTESIAN_POINT('Ctrl Pts',(-2.70520695291592,2.85716757218173,52.3261464484611));
#23263=CARTESIAN_POINT('Ctrl Pts',(-2.78588153773734,2.77621199797391,52.3319434106759));
#23264=CARTESIAN_POINT('Ctrl Pts',(-2.86645237806399,2.69536052960268,52.3377329182144));
#23265=CARTESIAN_POINT('Ctrl Pts',(-2.94362136416235,2.61087722211626,52.3435224257529));
#23266=CARTESIAN_POINT('Ctrl Pts',(-3.0170396055435,2.52308561459615,52.3493119332913));
#23267=CARTESIAN_POINT('Ctrl Pts',(-3.09037685056803,2.435390860395,52.3550950537384));
#23268=CARTESIAN_POINT('Ctrl Pts',(-3.15997131095199,2.34439539023446,52.3608781741855));
#23269=CARTESIAN_POINT('Ctrl Pts',(-3.22551105566922,2.25045938193865,52.3666612946326));
#23270=CARTESIAN_POINT('Ctrl Pts',(-3.29101068199178,2.15658087404768,52.3724408750978));
#23271=CARTESIAN_POINT('Ctrl Pts',(-3.35246028148819,2.05976575145766,52.378220455563));
#23272=CARTESIAN_POINT('Ctrl Pts',(-3.40958866854164,1.96040661888102,52.3840000360282));
#23273=CARTESIAN_POINT('Ctrl Pts',(-3.46669676108072,1.86108278303597,52.3897775633324));
#23274=CARTESIAN_POINT('Ctrl Pts',(-3.51948648055126,1.75921710129378,52.3955550906365));
#23275=CARTESIAN_POINT('Ctrl Pts',(-3.56773087095463,1.65522972195325,52.4013326179407));
#23276=CARTESIAN_POINT('Ctrl Pts',(-3.61597051469422,1.55125257371154,52.4071095768062));
#23277=CARTESIAN_POINT('Ctrl Pts',(-3.65966554066308,1.44515452875821,52.4128865356716));
#23278=CARTESIAN_POINT('Ctrl Pts',(-3.69863610549226,1.33737801654922,52.4186634945371));
#23279=CARTESIAN_POINT('Ctrl Pts',(-3.73763365884993,1.22952686519958,52.4244444541559));
#23280=CARTESIAN_POINT('Ctrl Pts',(-3.77190006757119,1.11999532388408,52.4302254137747));
#23281=CARTESIAN_POINT('Ctrl Pts',(-3.80130464568568,1.0092432762662,52.4360063733935));
#23282=CARTESIAN_POINT('Ctrl Pts',(-3.83071867342992,0.898455636712971,
52.4417891908159));
#23283=CARTESIAN_POINT('Ctrl Pts',(-3.85526766537381,0.786447124592048,
52.4475720082382));
#23284=CARTESIAN_POINT('Ctrl Pts',(-3.87487198407122,0.673688434708522,
52.4533548256605));
#23285=CARTESIAN_POINT('Ctrl Pts',(-3.89450369890896,0.56077216970399,52.4591457243062));
#23286=CARTESIAN_POINT('Ctrl Pts',(-3.90917687778931,0.447104054202614,
52.4649366229518));
#23287=CARTESIAN_POINT('Ctrl Pts',(-3.91886372212132,0.333160813184191,
52.4707275215975));
#23288=CARTESIAN_POINT('Ctrl Pts',(-3.92836763751898,0.221369306511939,
52.4764090633791));
#23289=CARTESIAN_POINT('Ctrl Pts',(-3.9330719559648,0.109313357446281,52.4820906051608));
#23290=CARTESIAN_POINT('Ctrl Pts',(-3.93299916752078,-0.00255896091143951,
52.4877721469424));
#23291=CARTESIAN_POINT('',(-3.93299851282984,0.00342024536944883,53.7377721470129));
#23292=CARTESIAN_POINT('Ctrl Pts',(-3.93299916752023,-0.00255896175136066,
52.4877721469851));
#23293=CARTESIAN_POINT('Ctrl Pts',(-3.93289543366542,-0.161992827610475,
52.4958691470615));
#23294=CARTESIAN_POINT('Ctrl Pts',(-3.9230971514168,-0.321109276650609,
52.503966147138));
#23295=CARTESIAN_POINT('Ctrl Pts',(-3.90371904854297,-0.479026711199759,
52.5120631472145));
#23296=CARTESIAN_POINT('Ctrl Pts',(-3.88965284348736,-0.593656044663781,
52.5179406092216));
#23297=CARTESIAN_POINT('Ctrl Pts',(-3.8705103217993,-0.707853182698984,
52.5238180712288));
#23298=CARTESIAN_POINT('Ctrl Pts',(-3.84632666030604,-0.821133498414874,
52.5296955332359));
#23299=CARTESIAN_POINT('Ctrl Pts',(-3.82217390497882,-0.934269044479273,
52.535565483981));
#23300=CARTESIAN_POINT('Ctrl Pts',(-3.79299290768883,-1.04648969857835,
52.5414354347262));
#23301=CARTESIAN_POINT('Ctrl Pts',(-3.75887055019978,-1.15731637283887,
52.5473053854714));
#23302=CARTESIAN_POINT('Ctrl Pts',(-3.72478272118824,-1.26803090137994,
52.5531693964024));
#23303=CARTESIAN_POINT('Ctrl Pts',(-3.68576359884078,-1.37735386398089,
52.5590334073333));
#23304=CARTESIAN_POINT('Ctrl Pts',(-3.64195087718146,-1.48481743261495,
52.5648974182643));
#23305=CARTESIAN_POINT('Ctrl Pts',(-3.59691156292701,-1.59528957986593,
52.5709255996032));
#23306=CARTESIAN_POINT('Ctrl Pts',(-3.54680636522229,-1.70379624693751,
52.5769537809421));
#23307=CARTESIAN_POINT('Ctrl Pts',(-3.49183961551256,-1.80984670608788,
52.582981962281));
#23308=CARTESIAN_POINT('Ctrl Pts',(-3.43843000629795,-1.9128928860087,52.5888393726479));
#23309=CARTESIAN_POINT('Ctrl Pts',(-3.38043079343676,-2.01361976233204,
52.5946967830148));
#23310=CARTESIAN_POINT('Ctrl Pts',(-3.31807746483069,-2.11159914221019,
52.6005541933816));
#23311=CARTESIAN_POINT('Ctrl Pts',(-3.25573314145588,-2.20956437164931,
52.606410757806));
#23312=CARTESIAN_POINT('Ctrl Pts',(-3.18903617419951,-2.30478254577666,
52.6122673222303));
#23313=CARTESIAN_POINT('Ctrl Pts',(-3.11826640271812,-2.39685286191695,
52.6181238866546));
#23314=CARTESIAN_POINT('Ctrl Pts',(-3.04748980263395,-2.48893206195786,
52.6239810161811));
#23315=CARTESIAN_POINT('Ctrl Pts',(-2.9726398684988,-2.57786247314646,52.6298381457076));
#23316=CARTESIAN_POINT('Ctrl Pts',(-2.89403745660768,-2.66327546448951,
52.6356952752341));
#23317=CARTESIAN_POINT('Ctrl Pts',(-2.81141695282054,-2.75305469905683,
52.6418518164977));
#23318=CARTESIAN_POINT('Ctrl Pts',(-2.72465051699632,-2.83894700917189,
52.6480083577613));
#23319=CARTESIAN_POINT('Ctrl Pts',(-2.63415450019974,-2.92056827844814,
52.6541648990249));
#23320=CARTESIAN_POINT('Ctrl Pts',(-2.54793131003757,-2.99833574790375,
52.6600307553012));
#23321=CARTESIAN_POINT('Ctrl Pts',(-2.45832304356354,-3.07222605884105,
52.6658966115776));
#23322=CARTESIAN_POINT('Ctrl Pts',(-2.36572271466626,-3.14194924168297,
52.6717624678539));
#23323=CARTESIAN_POINT('Ctrl Pts',(-2.27305871481266,-3.21172036540999,
52.6776323574278));
#23324=CARTESIAN_POINT('Ctrl Pts',(-2.17739889520996,-3.27731842298028,
52.6835022470017));
#23325=CARTESIAN_POINT('Ctrl Pts',(-2.07916395915626,-3.33849760085966,
52.6893721365756));
#23326=CARTESIAN_POINT('Ctrl Pts',(-1.98078972445159,-3.3997635317547,52.6952503497433));
#23327=CARTESIAN_POINT('Ctrl Pts',(-1.87983344487127,-3.4565978783223,52.7011285629109));
#23328=CARTESIAN_POINT('Ctrl Pts',(-1.7767390125329,-3.50880143087973,52.7070067760786));
#23329=CARTESIAN_POINT('Ctrl Pts',(-1.76173202460721,-3.5164004647474,52.7078624408515));
#23330=CARTESIAN_POINT('Ctrl Pts',(-1.74667976177442,-3.52390145991034,
52.7087181056243));
#23331=CARTESIAN_POINT('Ctrl Pts',(-1.7315836233202,-3.53130388885598,52.7095737703972));
#23332=CARTESIAN_POINT('Ctrl Pts',(-1.62789036507499,-3.58215013530697,
52.7154512117399));
#23333=CARTESIAN_POINT('Ctrl Pts',(-1.5217856557316,-3.62850859087834,52.7213286530825));
#23334=CARTESIAN_POINT('Ctrl Pts',(-1.4136946120197,-3.67014394049423,52.7272060944252));
#23335=CARTESIAN_POINT('Ctrl Pts',(-1.30574171402068,-3.71172607806908,
52.7330760241064));
#23336=CARTESIAN_POINT('Ctrl Pts',(-1.19580791189216,-3.74859696758625,
52.7389459537876));
#23337=CARTESIAN_POINT('Ctrl Pts',(-1.0843419325385,-3.78056762581212,52.7448158834688));
#23338=CARTESIAN_POINT('Ctrl Pts',(-0.972988753274336,-3.81250593073046,
52.7506798729645));
#23339=CARTESIAN_POINT('Ctrl Pts',(-0.860106875249662,-3.83955375533025,
52.7565438624603));
#23340=CARTESIAN_POINT('Ctrl Pts',(-0.746163356290465,-3.86157082619617,
52.762407851956));
#23341=CARTESIAN_POINT('Ctrl Pts',(-0.629029262716038,-3.8842044052062,
52.7684360411904));
#23342=CARTESIAN_POINT('Ctrl Pts',(-0.510773607508695,-3.90152116614789,
52.7744642304247));
#23343=CARTESIAN_POINT('Ctrl Pts',(-0.391919043644409,-3.91342413536137,
52.780492419659));
#23344=CARTESIAN_POINT('Ctrl Pts',(-0.27643207297672,-3.92498984905145,
52.7863498078034));
#23345=CARTESIAN_POINT('Ctrl Pts',(-0.160380114023787,-3.93144439402871,
52.7922071959478));
#23346=CARTESIAN_POINT('Ctrl Pts',(-0.0442504582975385,-3.93275105961977,
52.7980645840922));
#23347=CARTESIAN_POINT('Ctrl Pts',(0.0718624205706841,-3.93405753644128,
52.8039211260396));
#23348=CARTESIAN_POINT('Ctrl Pts',(0.188052561520881,-3.93021760809878,
52.8097776679869));
#23349=CARTESIAN_POINT('Ctrl Pts',(0.303831382016254,-3.92124667565075,
52.8156342099343));
#23350=CARTESIAN_POINT('Ctrl Pts',(0.419621369536783,-3.91227487794405,
52.8214913167531));
#23351=CARTESIAN_POINT('Ctrl Pts',(0.534999546451255,-3.89817112419895,
52.827348423572));
#23352=CARTESIAN_POINT('Ctrl Pts',(0.649481866172758,-3.87900274626259,
52.8332055303908));
#23353=CARTESIAN_POINT('Ctrl Pts',(0.769817495718348,-3.85885431782447,
52.8393621023232));
#23354=CARTESIAN_POINT('Ctrl Pts',(0.889162734770879,-3.83310975009962,
52.8455186742557));
#23355=CARTESIAN_POINT('Ctrl Pts',(1.00696837892769,-3.80190790049414,52.8516752461882));
#23356=CARTESIAN_POINT('Ctrl Pts',(1.11921075431069,-3.77217953101635,52.857541079382));
#23357=CARTESIAN_POINT('Ctrl Pts',(1.23005523955511,-3.737497713706,52.8634069125758));
#23358=CARTESIAN_POINT('Ctrl Pts',(1.33904424806304,-3.69803319370301,52.8692727457696));
#23359=CARTESIAN_POINT('Ctrl Pts',(1.44810819413825,-3.65854153908191,52.8751426121341));
#23360=CARTESIAN_POINT('Ctrl Pts',(1.55531374291774,-3.61426079075785,52.8810124784986));
#23361=CARTESIAN_POINT('Ctrl Pts',(1.66022516286428,-3.56540901000043,52.886882344863));
#23362=CARTESIAN_POINT('Ctrl Pts',(1.76528534866728,-3.51648795673666,52.8927605347799));
#23363=CARTESIAN_POINT('Ctrl Pts',(1.86804455018492,-3.46298312700869,52.8986387246967));
#23364=CARTESIAN_POINT('Ctrl Pts',(1.96809340004735,-3.40515746606379,52.9045169146135));
#23365=CARTESIAN_POINT('Ctrl Pts',(1.98265986360733,-3.39673842492396,52.9053727409357));
#23366=CARTESIAN_POINT('Ctrl Pts',(1.99716892846468,-3.38822786534177,52.906228567258));
#23367=CARTESIAN_POINT('Ctrl Pts',(2.0116193876095,-3.37962667160051,52.9070843935802));
#23368=CARTESIAN_POINT('Ctrl Pts',(2.11085911684612,-3.32055725868841,52.9129618519808));
#23369=CARTESIAN_POINT('Ctrl Pts',(2.20765753343926,-3.257016191809,52.9188393103813));
#23370=CARTESIAN_POINT('Ctrl Pts',(2.30158528416095,-3.18923096995714,52.9247167687819));
#23371=CARTESIAN_POINT('Ctrl Pts',(2.39539299459476,-3.12153237806801,52.9305867157516));
#23372=CARTESIAN_POINT('Ctrl Pts',(2.48633700384373,-3.04960065758682,52.9364566627214));
#23373=CARTESIAN_POINT('Ctrl Pts',(2.57401386514186,-2.97370839559924,52.9423266096912));
#23374=CARTESIAN_POINT('Ctrl Pts',(2.6616020035624,-2.89789293129545,52.9481906166834));
#23375=CARTESIAN_POINT('Ctrl Pts',(2.7459292603824,-2.81812516606789,52.9540546236756));
#23376=CARTESIAN_POINT('Ctrl Pts',(2.82662297125485,-2.73471965261055,52.9599186306678));
#23377=CARTESIAN_POINT('Ctrl Pts',(2.90957587988532,-2.64897901852271,52.9659468134218));
#23378=CARTESIAN_POINT('Ctrl Pts',(2.98868841453171,-2.55939418855801,52.9719749961758));
#23379=CARTESIAN_POINT('Ctrl Pts',(3.06359380707849,-2.46634993162573,52.9780031789297));
#23380=CARTESIAN_POINT('Ctrl Pts',(3.13637715108831,-2.37594159211652,52.9838605849751));
#23381=CARTESIAN_POINT('Ctrl Pts',(3.2051882516026,-2.28226754593297,52.9897179910205));
#23382=CARTESIAN_POINT('Ctrl Pts',(3.26973012950807,-2.18571587361831,52.9955753970659));
#23383=CARTESIAN_POINT('Ctrl Pts',(3.33426268460913,-2.08917814778903,53.0014319570335));
#23384=CARTESIAN_POINT('Ctrl Pts',(3.39452701418716,-1.9897639652298,53.0072885170011));
#23385=CARTESIAN_POINT('Ctrl Pts',(3.45026908043435,-1.88789095887411,53.0131450769686));
#23386=CARTESIAN_POINT('Ctrl Pts',(3.50601652401266,-1.78600812502327,53.0190022019074));
#23387=CARTESIAN_POINT('Ctrl Pts',(3.55724063901352,-1.68166635773221,53.0248593268462));
#23388=CARTESIAN_POINT('Ctrl Pts',(3.60373336091434,-1.57530786306453,53.030716451785));
#23389=CARTESIAN_POINT('Ctrl Pts',(3.65260283771765,-1.46351221472446,53.0368729988665));
#23390=CARTESIAN_POINT('Ctrl Pts',(3.69624417043921,-1.349488654406,53.043029545948));
#23391=CARTESIAN_POINT('Ctrl Pts',(3.73447360609827,-1.23377302829787,53.0491860930295));
#23392=CARTESIAN_POINT('Ctrl Pts',(3.77089795007778,-1.12352118448947,53.0550519444279));
#23393=CARTESIAN_POINT('Ctrl Pts',(3.80240973273049,-1.01173383485323,53.0609177958264));
#23394=CARTESIAN_POINT('Ctrl Pts',(3.8289019601574,-0.898887523276836,53.0667836472248));
#23395=CARTESIAN_POINT('Ctrl Pts',(3.85541240290985,-0.785963621686248,
53.072653531821));
#23396=CARTESIAN_POINT('Ctrl Pts',(3.87689634188851,-0.671979712553978,
53.0785234164173));
#23397=CARTESIAN_POINT('Ctrl Pts',(3.89329835365933,-0.557419886076462,
53.0843933010135));
#23398=CARTESIAN_POINT('Ctrl Pts',(3.90972362344108,-0.442697614056647,
53.0902715090911));
#23399=CARTESIAN_POINT('Ctrl Pts',(3.92105254676972,-0.327398203845943,
53.0961497171688));
#23400=CARTESIAN_POINT('Ctrl Pts',(3.92728169715956,-0.212008186529219,
53.1020279252464));
#23401=CARTESIAN_POINT('Ctrl Pts',(3.92818848138756,-0.195210735637382,
53.1028836224186));
#23402=CARTESIAN_POINT('Ctrl Pts',(3.92898728655392,-0.178411359029593,
53.1037393195908));
#23403=CARTESIAN_POINT('Ctrl Pts',(3.92967819380633,-0.16161155009135,53.104595016763));
#23404=CARTESIAN_POINT('Ctrl Pts',(3.93442376957651,-0.0462201340038854,
53.1104724710128));
#23405=CARTESIAN_POINT('Ctrl Pts',(3.93409027677237,0.0695696312581488,
53.1163499252626));
#23406=CARTESIAN_POINT('Ctrl Pts',(3.92863368139037,0.185273844471055,53.1222273795125));
#23407=CARTESIAN_POINT('Ctrl Pts',(3.92318405960244,0.30083018631742,53.1280973223056));
#23408=CARTESIAN_POINT('Ctrl Pts',(3.91262437565026,0.416300785173605,53.1339672650987));
#23409=CARTESIAN_POINT('Ctrl Pts',(3.89696251336728,0.531198804036748,53.1398372078918));
#23410=CARTESIAN_POINT('Ctrl Pts',(3.88131649986442,0.645980553620793,53.1457012106867));
#23411=CARTESIAN_POINT('Ctrl Pts',(3.86057863363714,0.760190469397612,53.1515652134817));
#23412=CARTESIAN_POINT('Ctrl Pts',(3.83480876508224,0.873344568454129,53.1574292162767));
#23413=CARTESIAN_POINT('Ctrl Pts',(3.80831738658687,0.989666778636287,53.1634574005962));
#23414=CARTESIAN_POINT('Ctrl Pts',(3.77650808360688,1.10487273239808,53.1694855849158));
#23415=CARTESIAN_POINT('Ctrl Pts',(3.73950273839359,1.21844502114242,53.1755137692353));
#23416=CARTESIAN_POINT('Ctrl Pts',(3.70354577936992,1.3287997309571,53.1813711710597));
#23417=CARTESIAN_POINT('Ctrl Pts',(3.66268337654109,1.43761168075823,53.1872285728841));
#23418=CARTESIAN_POINT('Ctrl Pts',(3.61707831474994,1.54442010637185,53.1930859747086));
#23419=CARTESIAN_POINT('Ctrl Pts',(3.57147984043455,1.65121310391924,53.1989425304538));
#23420=CARTESIAN_POINT('Ctrl Pts',(3.52114023135627,1.7560027734931,53.204799086199));
#23421=CARTESIAN_POINT('Ctrl Pts',(3.46627048514959,1.85834817076369,53.2106556419443));
#23422=CARTESIAN_POINT('Ctrl Pts',(3.41139544572767,1.96070344116572,53.2165127626641));
#23423=CARTESIAN_POINT('Ctrl Pts',(3.3519895953428,2.06061360696042,53.2223698833839));
#23424=CARTESIAN_POINT('Ctrl Pts',(3.28830963052443,2.15766280354466,53.2282270041037));
#23425=CARTESIAN_POINT('Ctrl Pts',(3.22137416916708,2.25967342440876,53.2343835570905));
#23426=CARTESIAN_POINT('Ctrl Pts',(3.14971629912284,2.35852238921075,53.2405401100774));
#23427=CARTESIAN_POINT('Ctrl Pts',(3.07368443022098,2.45376303326484,53.2466966630642));
#23428=CARTESIAN_POINT('Ctrl Pts',(3.00124270376511,2.54450651732878,53.2525625102915));
#23429=CARTESIAN_POINT('Ctrl Pts',(2.92483093237803,2.63197437799811,53.2584283575188));
#23430=CARTESIAN_POINT('Ctrl Pts',(2.84478979244263,2.71581664270881,53.2642942047462));
#23431=CARTESIAN_POINT('Ctrl Pts',(2.76469361815354,2.79971655533474,53.2701640851883));
#23432=CARTESIAN_POINT('Ctrl Pts',(2.68096340321106,2.87998562344194,53.2760339656304));
#23433=CARTESIAN_POINT('Ctrl Pts',(2.59397431994681,2.95631294477707,53.2819038460725));
#23434=CARTESIAN_POINT('Ctrl Pts',(2.50686188556649,3.03274849877679,53.2877820500453));
#23435=CARTESIAN_POINT('Ctrl Pts',(2.41648168233906,3.10523089601225,53.2936602540181));
#23436=CARTESIAN_POINT('Ctrl Pts',(2.32323933546826,3.17349145108868,53.2995384579909));
#23437=CARTESIAN_POINT('Ctrl Pts',(2.30966545749243,3.18342857168104,53.3003941853092));
#23438=CARTESIAN_POINT('Ctrl Pts',(2.29603096802954,3.19327629945579,53.3012499126276));
#23439=CARTESIAN_POINT('Ctrl Pts',(2.282337162349,3.20303388638969,53.3021056399459));
#23440=CARTESIAN_POINT('Ctrl Pts',(2.18828303191081,3.2700526082595,53.3079830921821));
#23441=CARTESIAN_POINT('Ctrl Pts',(2.09112031510791,3.3330349618521,53.3138605444183));
#23442=CARTESIAN_POINT('Ctrl Pts',(1.99123024842126,3.39167968678827,53.3197379966545));
#23443=CARTESIAN_POINT('Ctrl Pts',(1.89146784322042,3.45024946260318,53.3256079373901));
#23444=CARTESIAN_POINT('Ctrl Pts',(1.78898537272642,3.50449242759051,53.3314778781258));
#23445=CARTESIAN_POINT('Ctrl Pts',(1.68419489763579,3.55414920153579,53.3373478188615));
#23446=CARTESIAN_POINT('Ctrl Pts',(1.5795104644201,3.60375572570973,53.3432118195581));
#23447=CARTESIAN_POINT('Ctrl Pts',(1.47252304305926,3.64878511486443,53.3490758202546));
#23448=CARTESIAN_POINT('Ctrl Pts',(1.36367069574011,3.68902307306144,53.3549398209512));
#23449=CARTESIAN_POINT('Ctrl Pts',(1.25177062424374,3.73038764176396,53.3609680060419));
#23450=CARTESIAN_POINT('Ctrl Pts',(1.13790003310018,3.76668827743619,53.3669961911327));
#23451=CARTESIAN_POINT('Ctrl Pts',(1.02255887224883,3.79774437696709,53.3730243762234));
#23452=CARTESIAN_POINT('Ctrl Pts',(0.910485459841775,3.82792062129125,53.3788817758607));
#23453=CARTESIAN_POINT('Ctrl Pts',(0.797024109427844,3.85314539323487,53.3847391754981));
#23454=CARTESIAN_POINT('Ctrl Pts',(0.682649674448849,3.87330329589291,53.3905965751354));
#23455=CARTESIAN_POINT('Ctrl Pts',(0.56829176099391,3.89345828671778,53.3964531286643));
#23456=CARTESIAN_POINT('Ctrl Pts',(0.453021431388943,3.9085477921124,53.4023096821933));
#23457=CARTESIAN_POINT('Ctrl Pts',(0.33732327989459,3.91850762470116,53.4081662357222));
#23458=CARTESIAN_POINT('Ctrl Pts',(0.221613967672717,3.92846841805703,53.4140233541988));
#23459=CARTESIAN_POINT('Ctrl Pts',(0.10547716251848,3.93329851955016,53.4198804726754));
#23460=CARTESIAN_POINT('Ctrl Pts',(-0.0105985794115888,3.93298571954113,
53.425737591152));
#23461=CARTESIAN_POINT('Ctrl Pts',(-0.132608541830317,3.93265692804075,
53.43189414715));
#23462=CARTESIAN_POINT('Ctrl Pts',(-0.254550524003057,3.92664547323169,
53.4380507031481));
#23463=CARTESIAN_POINT('Ctrl Pts',(-0.375860063953985,3.91499913311925,
53.4442072591462));
#23464=CARTESIAN_POINT('Ctrl Pts',(-0.491441397236081,3.90390273032524,
53.4500731040828));
#23465=CARTESIAN_POINT('Ctrl Pts',(-0.606448242278903,3.88769155541726,
53.4559389490194));
#23466=CARTESIAN_POINT('Ctrl Pts',(-0.720401348885594,3.86645973682952,
53.461804793956));
#23467=CARTESIAN_POINT('Ctrl Pts',(-0.834432806611564,3.84521331980915,
53.4676746720912));
#23468=CARTESIAN_POINT('Ctrl Pts',(-0.947408682541798,3.81893947843412,
53.4735445502265));
#23469=CARTESIAN_POINT('Ctrl Pts',(-1.05886360324246,3.78778257952175,53.4794144283617));
#23470=CARTESIAN_POINT('Ctrl Pts',(-1.17047656767251,3.7565814999445,53.4852926300185));
#23471=CARTESIAN_POINT('Ctrl Pts',(-1.28056388315803,3.72048367430413,53.4911708316753));
#23472=CARTESIAN_POINT('Ctrl Pts',(-1.38867889737911,3.67968204060812,53.4970490333321));
#23473=CARTESIAN_POINT('Ctrl Pts',(-1.40441818308723,3.67374217578244,53.4979047765977));
#23474=CARTESIAN_POINT('Ctrl Pts',(-1.42011571071211,3.66770270190615,53.4987605198632));
#23475=CARTESIAN_POINT('Ctrl Pts',(-1.43577014599622,3.66156429519762,53.4996162631288));
#23476=CARTESIAN_POINT('Ctrl Pts',(-1.5432886424542,3.61940421417453,53.5054937175114));
#23477=CARTESIAN_POINT('Ctrl Pts',(-1.64912482168042,3.57243524253913,53.511371171894));
#23478=CARTESIAN_POINT('Ctrl Pts',(-1.75281807226117,3.52081209461037,53.5172486262766));
#23479=CARTESIAN_POINT('Ctrl Pts',(-1.85637880139806,3.4692549217963,53.5231185691892));
#23480=CARTESIAN_POINT('Ctrl Pts',(-1.95780168249082,3.41305558422226,53.5289885121017));
#23481=CARTESIAN_POINT('Ctrl Pts',(-2.05664434040339,3.35241749444886,53.5348584550143));
#23482=CARTESIAN_POINT('Ctrl Pts',(-2.15538697578883,3.29184076659254,53.5407224579154));
#23483=CARTESIAN_POINT('Ctrl Pts',(-2.25155423217577,3.22683443581695,53.5465864608165));
#23484=CARTESIAN_POINT('Ctrl Pts',(-2.34472728922019,3.15764832417832,53.5524504637176));
#23485=CARTESIAN_POINT('Ctrl Pts',(-2.44050902172943,3.08652512774648,53.5584786479924));
#23486=CARTESIAN_POINT('Ctrl Pts',(-2.53312601293964,3.0109848326888,53.5645068322671));
#23487=CARTESIAN_POINT('Ctrl Pts',(-2.62215385049671,2.93134750316733,53.5705350165419));
#23488=CARTESIAN_POINT('Ctrl Pts',(-2.70865947155471,2.85396635094919,53.5763924184383));
#23489=CARTESIAN_POINT('Ctrl Pts',(-2.79177624728224,2.77271748416481,53.5822498203347));
#23490=CARTESIAN_POINT('Ctrl Pts',(-2.87114809007967,2.68793557304335,53.5881072222311));
#23491=CARTESIAN_POINT('Ctrl Pts',(-2.95050846774535,2.6031659085291,53.5939637780354));
#23492=CARTESIAN_POINT('Ctrl Pts',(-3.02612470633072,2.51486451556273,53.5998203338398));
#23493=CARTESIAN_POINT('Ctrl Pts',(-3.09767828727034,2.42340220115729,53.6056768896442));
#23494=CARTESIAN_POINT('Ctrl Pts',(-3.16923877073477,2.33193106370083,53.6115340104101));
#23495=CARTESIAN_POINT('Ctrl Pts',(-3.23673556329017,2.2372987235491,53.617391131176));
#23496=CARTESIAN_POINT('Ctrl Pts',(-3.29989151612973,2.1399077040319,53.6232482519419));
#23497=CARTESIAN_POINT('Ctrl Pts',(-3.36627617471581,2.03753778814412,53.6294048048061));
#23498=CARTESIAN_POINT('Ctrl Pts',(-3.42786414134415,1.9321200930162,53.6355613576702));
#23499=CARTESIAN_POINT('Ctrl Pts',(-3.48438703987511,1.82415349034845,53.6417179105343));
#23500=CARTESIAN_POINT('Ctrl Pts',(-3.53824098958627,1.7212849513727,53.6475837577743));
#23501=CARTESIAN_POINT('Ctrl Pts',(-3.58749715010143,1.61610312423735,53.6534496050142));
#23502=CARTESIAN_POINT('Ctrl Pts',(-3.63197252110668,1.50906083572732,53.6593154522541));
#23503=CARTESIAN_POINT('Ctrl Pts',(-3.67647847221435,1.40194494773806,53.6651853326972));
#23504=CARTESIAN_POINT('Ctrl Pts',(-3.71619694748043,1.29296643767073,53.6710552131403));
#23505=CARTESIAN_POINT('Ctrl Pts',(-3.75099460567478,1.18259395745063,53.6769250935835));
#23506=CARTESIAN_POINT('Ctrl Pts',(-3.78584160708895,1.07206496860795,53.6828032975408));
#23507=CARTESIAN_POINT('Ctrl Pts',(-3.81575376210587,0.960138462149633,
53.6886815014981));
#23508=CARTESIAN_POINT('Ctrl Pts',(-3.84064863891855,0.847293946852686,
53.6945597054554));
#23509=CARTESIAN_POINT('Ctrl Pts',(-3.84427274199704,0.83086646426835,53.6954154324075));
#23510=CARTESIAN_POINT('Ctrl Pts',(-3.84779060633735,0.814419535852366,
53.6962711593596));
#23511=CARTESIAN_POINT('Ctrl Pts',(-3.85120206934889,0.797954648487541,
53.6971268863117));
#23512=CARTESIAN_POINT('Ctrl Pts',(-3.88411142825167,0.639122825967867,
53.7053818271666));
#23513=CARTESIAN_POINT('Ctrl Pts',(-3.90720373726939,0.478193253192053,
53.7136367680216));
#23514=CARTESIAN_POINT('Ctrl Pts',(-3.92027074357112,0.316174472562933,
53.7218917088766));
#23515=CARTESIAN_POINT('Ctrl Pts',(-3.9286499590609,0.212279958017212,53.7271851882461));
#23516=CARTESIAN_POINT('Ctrl Pts',(-3.93290762134356,0.107937899618637,
53.7324786676156));
#23517=CARTESIAN_POINT('Ctrl Pts',(-3.93299851282936,0.00342024591839455,
53.7377721469851));
#23518=CARTESIAN_POINT('',(-3.93299993366718,-0.000722339297042056,54.9877721470192));
#23519=CARTESIAN_POINT('Ctrl Pts',(-3.93299851282984,0.00342024536945145,
53.7377721470129));
#23520=CARTESIAN_POINT('Ctrl Pts',(-3.93309782495112,-0.110780457536849,
53.7435560413447));
#23521=CARTESIAN_POINT('Ctrl Pts',(-3.92821894975723,-0.225136164102259,
53.7493399356766));
#23522=CARTESIAN_POINT('Ctrl Pts',(-3.91834811321992,-0.339171142088976,
53.7551238300084));
#23523=CARTESIAN_POINT('Ctrl Pts',(-3.90842748530965,-0.453781345701163,
53.760936899987));
#23524=CARTESIAN_POINT('Ctrl Pts',(-3.89346434589926,-0.568067143825446,
53.7667499699656));
#23525=CARTESIAN_POINT('Ctrl Pts',(-3.87349782141296,-0.681545029700275,
53.7725630399442));
#23526=CARTESIAN_POINT('Ctrl Pts',(-3.85365782255742,-0.794303818914209,
53.778339273149));
#23527=CARTESIAN_POINT('Ctrl Pts',(-3.82887774495513,-0.906264481991354,
53.7841155063538));
#23528=CARTESIAN_POINT('Ctrl Pts',(-3.79924787160019,-1.01695850954772,
53.7898917395586));
#23529=CARTESIAN_POINT('Ctrl Pts',(-3.76962409111945,-1.12762977477982,
53.7956667849803));
#23530=CARTESIAN_POINT('Ctrl Pts',(-3.73515260675471,-1.23703451145412,
53.801441830402));
#23531=CARTESIAN_POINT('Ctrl Pts',(-3.69597431911322,-1.34471663649098,
53.8072168758238));
#23532=CARTESIAN_POINT('Ctrl Pts',(-3.65679400999867,-1.45240431757759,
53.8129922192192));
#23533=CARTESIAN_POINT('Ctrl Pts',(-3.6129065613013,-1.55836881101843,53.8187675626146));
#23534=CARTESIAN_POINT('Ctrl Pts',(-3.56450172826051,-1.66217220203803,
53.82454290601));
#23535=CARTESIAN_POINT('Ctrl Pts',(-3.51554478973708,-1.76715957444332,
53.830384122967));
#23536=CARTESIAN_POINT('Ctrl Pts',(-3.46196694765328,-1.86993582771499,
53.8362253399241));
#23537=CARTESIAN_POINT('Ctrl Pts',(-3.40401258402014,-1.9700729244961,53.8420665568811));
#23538=CARTESIAN_POINT('Ctrl Pts',(-3.34663156875354,-2.06921935487574,
53.8478499860895));
#23539=CARTESIAN_POINT('Ctrl Pts',(-3.2849605244318,-2.16577828798427,53.8536334152978));
#23540=CARTESIAN_POINT('Ctrl Pts',(-3.21927990030367,-2.25936405289206,
53.8594168445062));
#23541=CARTESIAN_POINT('Ctrl Pts',(-3.15261485968217,-2.35435247454594,
53.8652869553376));
#23542=CARTESIAN_POINT('Ctrl Pts',(-3.08181935582498,-2.44627752267562,
53.871157066169));
#23543=CARTESIAN_POINT('Ctrl Pts',(-3.00722764157043,-2.53477235896536,
53.8770271770004));
#23544=CARTESIAN_POINT('Ctrl Pts',(-2.93263592731587,-2.62326719525511,
53.8828972878317));
#23545=CARTESIAN_POINT('Ctrl Pts',(-2.85424835797467,-2.70833153463351,
53.8887673986631));
#23546=CARTESIAN_POINT('Ctrl Pts',(-2.77243547735778,-2.78963985558853,
53.8946375094945));
#23547=CARTESIAN_POINT('Ctrl Pts',(-2.69052025997408,-2.87104988217497,
53.9005149630348));
#23548=CARTESIAN_POINT('Ctrl Pts',(-2.6048819364985,-2.94898225367245,53.906392416575));
#23549=CARTESIAN_POINT('Ctrl Pts',(-2.51584772932693,-3.0230777698962,53.9122698701153));
#23550=CARTESIAN_POINT('Ctrl Pts',(-2.42692730930555,-3.09707859085731,
53.9181398121753));
#23551=CARTESIAN_POINT('Ctrl Pts',(-2.33461995102914,-3.16725204701039,
53.9240097542353));
#23552=CARTESIAN_POINT('Ctrl Pts',(-2.23929009614874,-3.23327525356104,
53.9298796962953));
#23553=CARTESIAN_POINT('Ctrl Pts',(-2.14405670922281,-3.29923164868424,
53.9357436983346));
#23554=CARTESIAN_POINT('Ctrl Pts',(-2.04580724688095,-3.36104591479999,
53.941607700374));
#23555=CARTESIAN_POINT('Ctrl Pts',(-1.94493913198957,-3.41843542762704,
53.9474717024134));
#23556=CARTESIAN_POINT('Ctrl Pts',(-1.84124687333006,-3.47743175381808,
53.9534998870077));
#23557=CARTESIAN_POINT('Ctrl Pts',(-1.73478749737503,-3.53175160520393,
53.9595280716021));
#23558=CARTESIAN_POINT('Ctrl Pts',(-1.62602496631928,-3.58113554740761,
53.9655562561964));
#23559=CARTESIAN_POINT('Ctrl Pts',(-1.52034376991476,-3.62912040068931,
53.971413657214));
#23560=CARTESIAN_POINT('Ctrl Pts',(-1.41248856738544,-3.67244508538788,
53.9772710582315));
#23561=CARTESIAN_POINT('Ctrl Pts',(-1.30290915295375,-3.71091858427929,
53.983128459249));
#23562=CARTESIAN_POINT('Ctrl Pts',(-1.19334556718039,-3.7493865257047,53.9889850141697));
#23563=CARTESIAN_POINT('Ctrl Pts',(-1.08205865387832,-3.7830045381676,53.9948415690904));
#23564=CARTESIAN_POINT('Ctrl Pts',(-0.969516139116825,-3.81163055082625,
54.0006981240111));
#23565=CARTESIAN_POINT('Ctrl Pts',(-0.856962767843835,-3.84025932491809,
54.0065552438894));
#23566=CARTESIAN_POINT('Ctrl Pts',(-0.743153954117419,-3.86389504022431,
54.0124123637677));
#23567=CARTESIAN_POINT('Ctrl Pts',(-0.628569778541057,-3.88244626923604,
54.0182694836461));
#23568=CARTESIAN_POINT('Ctrl Pts',(-0.508127703087051,-3.90194589484452,
54.024426037732));
#23569=CARTESIAN_POINT('Ctrl Pts',(-0.386829391856616,-3.91582732679284,
54.0305825918179));
#23570=CARTESIAN_POINT('Ctrl Pts',(-0.265239568459779,-3.92404599505705,
54.0367391459039));
#23571=CARTESIAN_POINT('Ctrl Pts',(-0.149391122737724,-3.93187658414514,
54.0426049922546));
#23572=CARTESIAN_POINT('Ctrl Pts',(-0.0332784881345224,-3.93456702174815,
54.0484708386054));
#23573=CARTESIAN_POINT('Ctrl Pts',(0.0826101593482019,-3.93213231740394,
54.0543366849561));
#23574=CARTESIAN_POINT('Ctrl Pts',(0.19857848883911,-3.92969593902059,54.0602065645097));
#23575=CARTESIAN_POINT('Ctrl Pts',(0.314322114061851,-3.92212742860087,
54.0660764440632));
#23576=CARTESIAN_POINT('Ctrl Pts',(0.429358388695931,-3.90949362118119,
54.0719463236167));
#23577=CARTESIAN_POINT('Ctrl Pts',(0.544557785348789,-3.89684189895874,
54.0778245266892));
#23578=CARTESIAN_POINT('Ctrl Pts',(0.659047424167076,-3.87911061047516,
54.0837027297616));
#23579=CARTESIAN_POINT('Ctrl Pts',(0.772355239372889,-3.85641755833224,
54.089580932834));
#23580=CARTESIAN_POINT('Ctrl Pts',(0.788850291906667,-3.85311396372521,
54.0904366661151));
#23581=CARTESIAN_POINT('Ctrl Pts',(0.805320326206703,-3.84970530131541,
54.0912923993963));
#23582=CARTESIAN_POINT('Ctrl Pts',(0.82176391592408,-3.84619202153053,54.0921481326774));
#23583=CARTESIAN_POINT('Ctrl Pts',(0.93470382495127,-3.822061676143,54.0980255864806));
#23584=CARTESIAN_POINT('Ctrl Pts',(1.0467651161977,-3.79291300036868,54.1039030402837));
#23585=CARTESIAN_POINT('Ctrl Pts',(1.15746816109081,-3.7588238128517,54.1097804940869));
#23586=CARTESIAN_POINT('Ctrl Pts',(1.26802972579053,-3.72477819184048,54.1156504364138));
#23587=CARTESIAN_POINT('Ctrl Pts',(1.37723610560554,-3.68580473651154,54.1215203787406));
#23588=CARTESIAN_POINT('Ctrl Pts',(1.48461775345995,-3.64203227966358,54.1273903210675));
#23589=CARTESIAN_POINT('Ctrl Pts',(1.59189073775631,-3.5983041178232,54.1332543233773));
#23590=CARTESIAN_POINT('Ctrl Pts',(1.69734228333967,-3.54978676925473,54.1391183256871));
#23591=CARTESIAN_POINT('Ctrl Pts',(1.80051854434761,-3.49665868672656,54.1449823279969));
#23592=CARTESIAN_POINT('Ctrl Pts',(1.90658356682353,-3.44204310740237,54.1510105124912));
#23593=CARTESIAN_POINT('Ctrl Pts',(2.01024358749085,-3.3825549190365,54.1570386969855));
#23594=CARTESIAN_POINT('Ctrl Pts',(2.11102782971279,-3.31844097464127,54.1630668814798));
#23595=CARTESIAN_POINT('Ctrl Pts',(2.20895677523108,-3.25614342862393,54.1689242827749));
#23596=CARTESIAN_POINT('Ctrl Pts',(2.30417032999127,-3.18947894643206,54.17478168407));
#23597=CARTESIAN_POINT('Ctrl Pts',(2.3962627612175,-3.11871989431597,54.1806390853651));
#23598=CARTESIAN_POINT('Ctrl Pts',(2.48834188980075,-3.04797106326143,54.1864956405655));
#23599=CARTESIAN_POINT('Ctrl Pts',(2.57730046434993,-2.97312908966979,54.1923521957659));
#23600=CARTESIAN_POINT('Ctrl Pts',(2.66276395042939,-2.89450810057489,54.1982087509663));
#23601=CARTESIAN_POINT('Ctrl Pts',(2.7482356808452,-2.8158795272132,54.2040658711262));
#23602=CARTESIAN_POINT('Ctrl Pts',(2.8302113489587,-2.73347149294836,54.2099229912862));
#23603=CARTESIAN_POINT('Ctrl Pts',(2.9083520871297,-2.6476361414077,54.2157801114461));
#23604=CARTESIAN_POINT('Ctrl Pts',(2.99048761408882,-2.55741262937631,54.2219366651473));
#23605=CARTESIAN_POINT('Ctrl Pts',(3.06838538698437,-2.4634024735282,54.2280932188485));
#23606=CARTESIAN_POINT('Ctrl Pts',(3.14169953943729,-2.36605431127425,54.2342497725496));
#23607=CARTESIAN_POINT('Ctrl Pts',(3.21155186190543,-2.27330284387086,54.2401156191841));
#23608=CARTESIAN_POINT('Ctrl Pts',(3.27724335250574,-2.17752178313405,54.2459814658186));
#23609=CARTESIAN_POINT('Ctrl Pts',(3.33851986779332,-2.0791282048852,54.2518473124531));
#23610=CARTESIAN_POINT('Ctrl Pts',(3.39983851521797,-1.98066697377286,54.2577171922911));
#23611=CARTESIAN_POINT('Ctrl Pts',(3.45673594091564,-1.87959000676744,54.2635870721291));
#23612=CARTESIAN_POINT('Ctrl Pts',(3.50900442940083,-1.77633806310771,54.269456951967));
#23613=CARTESIAN_POINT('Ctrl Pts',(3.56134703485703,-1.67293970768946,54.2753351553232));
#23614=CARTESIAN_POINT('Ctrl Pts',(3.60904743658074,-1.56736059581798,54.2812133586793));
#23615=CARTESIAN_POINT('Ctrl Pts',(3.65194638801383,-1.46006047103285,54.2870915620355));
#23616=CARTESIAN_POINT('Ctrl Pts',(3.65819148914052,-1.44444003958164,54.2879472933104));
#23617=CARTESIAN_POINT('Ctrl Pts',(3.66433492174529,-1.42878315875044,54.2888030245853));
#23618=CARTESIAN_POINT('Ctrl Pts',(3.67037628380472,-1.41309126926883,54.2896587558602));
#23619=CARTESIAN_POINT('Ctrl Pts',(3.71187041501763,-1.30531403050651,54.2955362095627));
#23620=CARTESIAN_POINT('Ctrl Pts',(3.74868137511156,-1.19553092150226,54.3014136632652));
#23621=CARTESIAN_POINT('Ctrl Pts',(3.78061229675617,-1.0841861747947,54.3072911169677));
#23622=CARTESIAN_POINT('Ctrl Pts',(3.81250241018582,-0.972983728406827,
54.3131610591929));
#23623=CARTESIAN_POINT('Ctrl Pts',(3.83952477586845,-0.860224006467499,
54.319031001418));
#23624=CARTESIAN_POINT('Ctrl Pts',(3.86153076176818,-0.746370669250853,
54.3249009436432));
#23625=CARTESIAN_POINT('Ctrl Pts',(3.88351447897329,-0.632632544559086,
54.3307649458505));
#23626=CARTESIAN_POINT('Ctrl Pts',(3.90049183611031,-0.51780340861447,54.3366289480577));
#23627=CARTESIAN_POINT('Ctrl Pts',(3.91236433905862,-0.402360880879767,
54.3424929502649));
#23628=CARTESIAN_POINT('Ctrl Pts',(3.92456925237632,-0.283686154049728,
54.3485211347974));
#23629=CARTESIAN_POINT('Ctrl Pts',(3.93137910493229,-0.164363605648615,
54.3545493193298));
#23630=CARTESIAN_POINT('Ctrl Pts',(3.93274344159755,-0.0449224061170324,
54.3605775038622));
#23631=CARTESIAN_POINT('Ctrl Pts',(3.93406912550207,0.0711349276675845,
54.3664349050533));
#23632=CARTESIAN_POINT('Ctrl Pts',(3.93025369795782,0.187303840308811,54.3722923062443));
#23633=CARTESIAN_POINT('Ctrl Pts',(3.92130360932623,0.303095700208723,54.3781497074353));
#23634=CARTESIAN_POINT('Ctrl Pts',(3.91235481352498,0.418870834103377,54.3840062625313));
#23635=CARTESIAN_POINT('Ctrl Pts',(3.89827286330148,0.53426861239305,54.3898628176272));
#23636=CARTESIAN_POINT('Ctrl Pts',(3.87911623126424,0.648803717885653,54.3957193727232));
#23637=CARTESIAN_POINT('Ctrl Pts',(3.85995775126064,0.763349872137798,54.4015764927784));
#23638=CARTESIAN_POINT('Ctrl Pts',(3.83572368434281,0.877032781296482,54.4074336128336));
#23639=CARTESIAN_POINT('Ctrl Pts',(3.8065238307318,0.989376230799395,54.4132907328889));
#23640=CARTESIAN_POINT('Ctrl Pts',(3.77583119179622,1.10746301912048,54.4194472867351));
#23641=CARTESIAN_POINT('Ctrl Pts',(3.7396517263843,1.22406927734305,54.4256038405813));
#23642=CARTESIAN_POINT('Ctrl Pts',(3.6981722300468,1.33866020965388,54.4317603944275));
#23643=CARTESIAN_POINT('Ctrl Pts',(3.65865136078463,1.44784025411824,54.4376262409575));
#23644=CARTESIAN_POINT('Ctrl Pts',(3.61431976499308,1.55519058108515,54.4434920874876));
#23645=CARTESIAN_POINT('Ctrl Pts',(3.56538791635528,1.66027046167415,54.4493579340177));
#23646=CARTESIAN_POINT('Ctrl Pts',(3.51642242345009,1.765422592458,54.4552278137514));
#23647=CARTESIAN_POINT('Ctrl Pts',(3.46285056939417,1.86830080349583,54.4610976934851));
#23648=CARTESIAN_POINT('Ctrl Pts',(3.40492802998567,1.96849031255372,54.4669675732188));
#23649=CARTESIAN_POINT('Ctrl Pts',(3.34692335612531,2.06882189083876,54.4728457764715));
#23650=CARTESIAN_POINT('Ctrl Pts',(3.28455590784092,2.16645681346466,54.4787239797241));
#23651=CARTESIAN_POINT('Ctrl Pts',(3.2181237423487,2.2610105216322,54.4846021829768));
#23652=CARTESIAN_POINT('Ctrl Pts',(3.208452737644,2.27477538011242,54.4854579149989));
#23653=CARTESIAN_POINT('Ctrl Pts',(3.19869565778891,2.28847499937988,54.4863136470211));
#23654=CARTESIAN_POINT('Ctrl Pts',(3.18885348983417,2.30210825557191,54.4871693790432));
#23655=CARTESIAN_POINT('Ctrl Pts',(3.12125418902311,2.39574601816625,54.4930468327347));
#23656=CARTESIAN_POINT('Ctrl Pts',(3.04941620835264,2.48655726347727,54.4989242864262));
#23657=CARTESIAN_POINT('Ctrl Pts',(2.97360405959491,2.57413439757147,54.5048017401177));
#23658=CARTESIAN_POINT('Ctrl Pts',(2.89788879994943,2.66159960671807,54.5106716823315));
#23659=CARTESIAN_POINT('Ctrl Pts',(2.81820974078964,2.74583861555468,54.5165416245452));
#23660=CARTESIAN_POINT('Ctrl Pts',(2.73487401906295,2.82647361563033,54.5224115667589));
#23661=CARTESIAN_POINT('Ctrl Pts',(2.65162262793072,2.90702701807475,54.5282755689543));
#23662=CARTESIAN_POINT('Ctrl Pts',(2.56472222951902,2.98398338113534,54.5341395711497));
#23663=CARTESIAN_POINT('Ctrl Pts',(2.47451904522582,3.0569992631361,54.5400035733451));
#23664=CARTESIAN_POINT('Ctrl Pts',(2.38179032129292,3.13205946880198,54.5460317578818));
#23665=CARTESIAN_POINT('Ctrl Pts',(2.28557142029616,3.2029549394754,54.5520599424185));
#23666=CARTESIAN_POINT('Ctrl Pts',(2.18627798661554,3.269354304024,54.5580881269552));
#23667=CARTESIAN_POINT('Ctrl Pts',(2.0897976164662,3.33387252070624,54.5639455281334));
#23668=CARTESIAN_POINT('Ctrl Pts',(1.990414948337,3.39414572349081,54.5698029293116));
#23669=CARTESIAN_POINT('Ctrl Pts',(1.88854276329811,3.44991235123362,54.5756603304899));
#23670=CARTESIAN_POINT('Ctrl Pts',(1.78668529358891,3.50567092354586,54.5815168855726));
#23671=CARTESIAN_POINT('Ctrl Pts',(1.68233938380184,3.55692401726563,54.5873734406554));
#23672=CARTESIAN_POINT('Ctrl Pts',(1.57594346133791,3.6034554536814,54.5932299957382));
#23673=CARTESIAN_POINT('Ctrl Pts',(1.46953727527553,3.64999137880283,54.59908711578));
#23674=CARTESIAN_POINT('Ctrl Pts',(1.36108106136615,3.6918045758734,54.6049442358217));
#23675=CARTESIAN_POINT('Ctrl Pts',(1.25103366585959,3.72872682921207,54.6108013558635));
#23676=CARTESIAN_POINT('Ctrl Pts',(1.13536031220635,3.76753666063479,54.616957909727));
#23677=CARTESIAN_POINT('Ctrl Pts',(1.01792926161511,3.80094207385933,54.6231144635905));
#23678=CARTESIAN_POINT('Ctrl Pts',(0.899290491862966,3.82880733535194,54.6292710174541));
#23679=CARTESIAN_POINT('Ctrl Pts',(0.786253746042588,3.85535682239686,54.63513686397));
#23680=CARTESIAN_POINT('Ctrl Pts',(0.672121154680575,3.87687738528061,54.6410027104859));
#23681=CARTESIAN_POINT('Ctrl Pts',(0.5573768456465,3.89330451569578,54.6468685570018));
#23682=CARTESIAN_POINT('Ctrl Pts',(0.44255364141266,3.90974294097818,54.6527384367211));
#23683=CARTESIAN_POINT('Ctrl Pts',(0.327118291381488,3.9210809200646,54.6586083164404));
#23684=CARTESIAN_POINT('Ctrl Pts',(0.211557887780263,3.92730597994579,54.6644781961596));
#23685=CARTESIAN_POINT('Ctrl Pts',(0.0958336189511281,3.9335398669929,54.6703563993976));
#23686=CARTESIAN_POINT('Ctrl Pts',(-0.0200156466463229,3.9346463640566,
54.6762346026355));
#23687=CARTESIAN_POINT('Ctrl Pts',(-0.135504975568601,3.9306650075523,54.6821128058735));
#23688=CARTESIAN_POINT('Ctrl Pts',(-0.152317583773183,3.93008541299016,
54.682968537991));
#23689=CARTESIAN_POINT('Ctrl Pts',(-0.169122577528871,3.92939808212121,
54.6838242701085));
#23690=CARTESIAN_POINT('Ctrl Pts',(-0.18591847626111,3.92860322763508,54.684680002226));
#23691=CARTESIAN_POINT('Ctrl Pts',(-0.30127831319858,3.92314390179777,54.6905574559491));
#23692=CARTESIAN_POINT('Ctrl Pts',(-0.416586581313027,3.91259017234618,
54.6964349096721));
#23693=CARTESIAN_POINT('Ctrl Pts',(-0.531357381452448,3.89694089423692,
54.7023123633952));
#23694=CARTESIAN_POINT('Ctrl Pts',(-0.645981502723869,3.88131161614852,
54.708182305641));
#23695=CARTESIAN_POINT('Ctrl Pts',(-0.760069116991416,3.86059979579573,
54.7140522478868));
#23696=CARTESIAN_POINT('Ctrl Pts',(-0.873135983901122,3.83485626244544,
54.7199221901326));
#23697=CARTESIAN_POINT('Ctrl Pts',(-0.986088434146258,3.80913877995604,
54.7257861923605));
#23698=CARTESIAN_POINT('Ctrl Pts',(-1.09802179182215,3.7783998039262,54.7316501945884));
#23699=CARTESIAN_POINT('Ctrl Pts',(-1.20845924694091,3.74274167536086,54.7375141968163));
#23700=CARTESIAN_POINT('Ctrl Pts',(-1.3219887668866,3.70608517857875,54.743542381341));
#23701=CARTESIAN_POINT('Ctrl Pts',(-1.43393693989953,3.66423005744842,54.7495705658657));
#23702=CARTESIAN_POINT('Ctrl Pts',(-1.54379913655438,3.61734339342756,54.7555987503903));
#23703=CARTESIAN_POINT('Ctrl Pts',(-1.65054884887056,3.57178506628599,54.761456151602));
#23704=CARTESIAN_POINT('Ctrl Pts',(-1.75532878853956,3.5214766367418,54.7673135528136));
#23705=CARTESIAN_POINT('Ctrl Pts',(-1.85769436035273,3.4666209287307,54.7731709540253));
#23706=CARTESIAN_POINT('Ctrl Pts',(-1.96004514557197,3.41177314456612,54.7790275091418));
#23707=CARTESIAN_POINT('Ctrl Pts',(-2.0599818929475,3.35237958288713,54.7848840642583));
#23708=CARTESIAN_POINT('Ctrl Pts',(-2.15708400579163,3.28868934257372,54.7907406193748));
#23709=CARTESIAN_POINT('Ctrl Pts',(-2.25419548570091,3.22499295830925,54.7965977394505));
#23710=CARTESIAN_POINT('Ctrl Pts',(-2.34847144255498,3.15699929770198,54.8024548595262));
#23711=CARTESIAN_POINT('Ctrl Pts',(-2.43952029561827,3.08500076616954,54.8083119796019));
#23712=CARTESIAN_POINT('Ctrl Pts',(-2.53522384217987,3.00932145135058,54.8144685334192));
#23713=CARTESIAN_POINT('Ctrl Pts',(-2.62736119639072,2.92921726301465,54.8206250872364));
#23714=CARTESIAN_POINT('Ctrl Pts',(-2.71551819351257,2.8450746810413,54.8267816410537));
#23715=CARTESIAN_POINT('Ctrl Pts',(-2.7995124917498,2.76490524066267,54.8326474876038));
#23716=CARTESIAN_POINT('Ctrl Pts',(-2.87989349302675,2.68107041608969,54.838513334154));
#23717=CARTESIAN_POINT('Ctrl Pts',(-2.95634266486319,2.59394044802684,54.8443791807041));
#23718=CARTESIAN_POINT('Ctrl Pts',(-3.03284440116098,2.50675057166507,54.8502490604578));
#23719=CARTESIAN_POINT('Ctrl Pts',(-3.10540866752619,2.41626136128656,54.8561189402114));
#23720=CARTESIAN_POINT('Ctrl Pts',(-3.17375889444228,2.32287396988054,54.861988819965));
#23721=CARTESIAN_POINT('Ctrl Pts',(-3.24220604231983,2.22935415468938,54.8678670232373));
#23722=CARTESIAN_POINT('Ctrl Pts',(-3.30642699960994,2.13292829994122,54.8737452265095));
#23723=CARTESIAN_POINT('Ctrl Pts',(-3.36618993711564,2.03402416584992,54.8796234297818));
#23724=CARTESIAN_POINT('Ctrl Pts',(-3.37489005316125,2.0196259873149,54.8804791616575));
#23725=CARTESIAN_POINT('Ctrl Pts',(-3.38349577378783,2.00517532465565,54.8813348935332));
#23726=CARTESIAN_POINT('Ctrl Pts',(-3.39200646822428,1.99067353413982,54.8821906254089));
#23727=CARTESIAN_POINT('Ctrl Pts',(-3.45257231638009,1.88747240890521,54.8882803901434));
#23728=CARTESIAN_POINT('Ctrl Pts',(-3.50850811753915,1.78136280708782,54.8943701548779));
#23729=CARTESIAN_POINT('Ctrl Pts',(-3.55953522084632,1.67278151937264,54.9004599196124));
#23730=CARTESIAN_POINT('Ctrl Pts',(-3.61048076066794,1.56437379174058,54.9065399502564));
#23731=CARTESIAN_POINT('Ctrl Pts',(-3.65653306873914,1.45350257799546,54.9126199809005));
#23732=CARTESIAN_POINT('Ctrl Pts',(-3.69745819945993,1.34063114362101,54.9187000115446));
#23733=CARTESIAN_POINT('Ctrl Pts',(-3.73830444202521,1.22797728263267,54.9247683221918));
#23734=CARTESIAN_POINT('Ctrl Pts',(-3.77404307991574,1.11333123252545,54.930836632839));
#23735=CARTESIAN_POINT('Ctrl Pts',(-3.80448766304021,0.997177327146436,
54.9369049434862));
#23736=CARTESIAN_POINT('Ctrl Pts',(-3.83489764772554,0.881155423700603,
54.9429663578631));
#23737=CARTESIAN_POINT('Ctrl Pts',(-3.86002546094088,0.763629433070065,
54.9490277722399));
#23738=CARTESIAN_POINT('Ctrl Pts',(-3.8797337597261,0.645100731391357,54.9550891866167));
#23739=CARTESIAN_POINT('Ctrl Pts',(-3.89941659063284,0.526725197401228,
54.9611427681833));
#23740=CARTESIAN_POINT('Ctrl Pts',(-3.91369380347358,0.407349899215915,
54.9671963497499));
#23741=CARTESIAN_POINT('Ctrl Pts',(-3.92247878698497,0.28748767913248,54.9732499313165));
#23742=CARTESIAN_POINT('Ctrl Pts',(-3.92950368752218,0.191640012126227,
54.9780906698727));
#23743=CARTESIAN_POINT('Ctrl Pts',(-3.93301760252523,0.0954813188314772,
54.9829314084289));
#23744=CARTESIAN_POINT('Ctrl Pts',(-3.9329999336673,-0.000722338618901584,
54.9877721469851));
#23745=CARTESIAN_POINT('',(-3.93299903070378,-0.00276124668366289,56.2377721469449));
#23746=CARTESIAN_POINT('Ctrl Pts',(-3.93299993366718,-0.000722339297067472,
54.9877721470192));
#23747=CARTESIAN_POINT('Ctrl Pts',(-3.93297720821431,-0.124458103037193,
54.9939982354881));
#23748=CARTESIAN_POINT('Ctrl Pts',(-3.927110968723,-0.248049901650573,55.0002243239571));
#23749=CARTESIAN_POINT('Ctrl Pts',(-3.91546729987528,-0.370951241549993,
55.006450412426));
#23750=CARTESIAN_POINT('Ctrl Pts',(-3.90378573984742,-0.494252530715322,
55.0126967620208));
#23751=CARTESIAN_POINT('Ctrl Pts',(-3.88628916959009,-0.616858538656386,
55.0189431116155));
#23752=CARTESIAN_POINT('Ctrl Pts',(-3.86309533707472,-0.738229921279,55.0251894612103));
#23753=CARTESIAN_POINT('Ctrl Pts',(-3.83986373499779,-0.859798948853376,
55.0314459825559));
#23754=CARTESIAN_POINT('Ctrl Pts',(-3.81091642630633,-0.980129019685123,
55.0377025039015));
#23755=CARTESIAN_POINT('Ctrl Pts',(-3.77642124542311,-1.09869539778642,
55.0439590252471));
#23756=CARTESIAN_POINT('Ctrl Pts',(-3.74182559238293,-1.21760711745272,
55.0502337696075));
#23757=CARTESIAN_POINT('Ctrl Pts',(-3.70164984674111,-1.33474455662902,
55.056508513968));
#23758=CARTESIAN_POINT('Ctrl Pts',(-3.65611105196853,-1.44960028134435,
55.0627832583285));
#23759=CARTESIAN_POINT('Ctrl Pts',(-3.61518375983273,-1.5528250992687,55.0684225884162));
#23760=CARTESIAN_POINT('Ctrl Pts',(-3.56992532214057,-1.65420707183091,
55.0740619185039));
#23761=CARTESIAN_POINT('Ctrl Pts',(-3.52052443902146,-1.7533957551713,55.0797012485916));
#23762=CARTESIAN_POINT('Ctrl Pts',(-3.46903757814324,-1.85677273180402,
55.0855787022998));
#23763=CARTESIAN_POINT('Ctrl Pts',(-3.41290911103248,-1.95804944682947,
55.0914561560079));
#23764=CARTESIAN_POINT('Ctrl Pts',(-3.35233380913251,-2.05678074479201,
55.097333609716));
#23765=CARTESIAN_POINT('Ctrl Pts',(-3.29183592341283,-2.15538586261638,
55.1032035519466));
#23766=CARTESIAN_POINT('Ctrl Pts',(-3.22690271905573,-2.25145168448782,
55.1090734941773));
#23767=CARTESIAN_POINT('Ctrl Pts',(-3.15777586579413,-2.34455551894345,
55.1149434364079));
#23768=CARTESIAN_POINT('Ctrl Pts',(-3.08871896462757,-2.43756513808378,
55.1208074386205));
#23769=CARTESIAN_POINT('Ctrl Pts',(-3.01547710049811,-2.52761840275179,
55.1266714408331));
#23770=CARTESIAN_POINT('Ctrl Pts',(-2.93833609211701,-2.61432018118719,
55.1325354430456));
#23771=CARTESIAN_POINT('Ctrl Pts',(-2.8590352636858,-2.70344946534716,55.138563627576));
#23772=CARTESIAN_POINT('Ctrl Pts',(-2.77561395333189,-2.78903643640921,
55.1445918121064));
#23773=CARTESIAN_POINT('Ctrl Pts',(-2.68842844146174,-2.87068659298427,
55.1506199966367));
#23774=CARTESIAN_POINT('Ctrl Pts',(-2.60371296552938,-2.95002353470586,
55.1564773978327));
#23775=CARTESIAN_POINT('Ctrl Pts',(-2.51544403133708,-3.0256434330798,55.1623347990287));
#23776=CARTESIAN_POINT('Ctrl Pts',(-2.42398643669716,-3.09722113429253,
55.1681922002246));
#23777=CARTESIAN_POINT('Ctrl Pts',(-2.3325420530075,-3.16878849618401,55.1740487553254));
#23778=CARTESIAN_POINT('Ctrl Pts',(-2.23791024954299,-3.23631456783101,
55.1799053104261));
#23779=CARTESIAN_POINT('Ctrl Pts',(-2.1404885033547,-3.29951480781741,55.1857618655268));
#23780=CARTESIAN_POINT('Ctrl Pts',(-2.04305735926919,-3.36272114448535,
55.1916189855866));
#23781=CARTESIAN_POINT('Ctrl Pts',(-1.94283608351721,-3.42160059543853,
55.1974761056465));
#23782=CARTESIAN_POINT('Ctrl Pts',(-1.84025009366266,-3.47591262732173,
55.2033332257063));
#23783=CARTESIAN_POINT('Ctrl Pts',(-1.7324195962137,-3.53300125534718,55.2094897795453));
#23784=CARTESIAN_POINT('Ctrl Pts',(-1.62197665314596,-3.58504286822423,
55.2156463333843));
#23785=CARTESIAN_POINT('Ctrl Pts',(-1.50944188025276,-3.63181417615757,
55.2218028872234));
#23786=CARTESIAN_POINT('Ctrl Pts',(-1.40222090488008,-3.67637698218755,
55.2276687337576));
#23787=CARTESIAN_POINT('Ctrl Pts',(-1.29310155049033,-3.71615574044766,
55.2335345802918));
#23788=CARTESIAN_POINT('Ctrl Pts',(-1.18255103060521,-3.751008139156,55.239400426826));
#23789=CARTESIAN_POINT('Ctrl Pts',(-1.07192449905926,-3.7858845014668,55.2452703065637));
#23790=CARTESIAN_POINT('Ctrl Pts',(-0.959865239997425,-3.8158276532582,
55.2511401863014));
#23791=CARTESIAN_POINT('Ctrl Pts',(-0.846851846557203,-3.84074614495448,
55.257010066039));
#23792=CARTESIAN_POINT('Ctrl Pts',(-0.733678199562052,-3.86569997119612,
55.2628882692954));
#23793=CARTESIAN_POINT('Ctrl Pts',(-0.619548123036424,-3.8856148496232,
55.2687664725518));
#23794=CARTESIAN_POINT('Ctrl Pts',(-0.504946530464559,-3.90045099973988,
55.2746446758081));
#23795=CARTESIAN_POINT('Ctrl Pts',(-0.488263158955069,-3.90261080396783,
55.275500407797));
#23796=CARTESIAN_POINT('Ctrl Pts',(-0.471569795818275,-3.90466306633423,
55.2763561397858));
#23797=CARTESIAN_POINT('Ctrl Pts',(-0.454867936511775,-3.90660775614004,
55.2772118717746));
#23798=CARTESIAN_POINT('Ctrl Pts',(-0.340153976662304,-3.91996453661635,
55.2830893254884));
#23799=CARTESIAN_POINT('Ctrl Pts',(-0.224663166259439,-3.92828622915271,
55.2889667792022));
#23800=CARTESIAN_POINT('Ctrl Pts',(-0.108874761772659,-3.93149275546184,
55.294844232916));
#23801=CARTESIAN_POINT('Ctrl Pts',(0.00676566332945326,-3.9346951837804,
55.3007141751524));
#23802=CARTESIAN_POINT('Ctrl Pts',(0.122702517450103,-3.93279543557375,
55.3065841173888));
#23803=CARTESIAN_POINT('Ctrl Pts',(0.238449736136254,-3.92576498574947,
55.3124540596252));
#23804=CARTESIAN_POINT('Ctrl Pts',(0.354079825805363,-3.91874165030502,
55.3183180618436));
#23805=CARTESIAN_POINT('Ctrl Pts',(0.469520252391502,-3.90659796577246,
55.3241820640619));
#23806=CARTESIAN_POINT('Ctrl Pts',(0.584283913491771,-3.88935744158784,
55.3300460662803));
#23807=CARTESIAN_POINT('Ctrl Pts',(0.702260766242369,-3.87163421139833,
55.3360742508085));
#23808=CARTESIAN_POINT('Ctrl Pts',(0.819521952844152,-3.84852450042129,
55.3421024353367));
#23809=CARTESIAN_POINT('Ctrl Pts',(0.935542402147672,-3.82011117819675,
55.348130619865));
#23810=CARTESIAN_POINT('Ctrl Pts',(1.04827589861093,-3.79250282829172,55.3539880210668));
#23811=CARTESIAN_POINT('Ctrl Pts',(1.15983758917749,-3.75988744853935,55.3598454222687));
#23812=CARTESIAN_POINT('Ctrl Pts',(1.26975583177661,-3.72239293031636,55.3657028234706));
#23813=CARTESIAN_POINT('Ctrl Pts',(1.37965819680554,-3.68490382813562,55.3715593785772));
#23814=CARTESIAN_POINT('Ctrl Pts',(1.48791719562057,-3.64253712211225,55.3774159336839));
#23815=CARTESIAN_POINT('Ctrl Pts',(1.59407734706772,-3.59547026292327,55.3832724887905));
#23816=CARTESIAN_POINT('Ctrl Pts',(1.70024773937251,-3.54839886337712,55.3891296088563));
#23817=CARTESIAN_POINT('Ctrl Pts',(1.8043185047075,-3.49662657653291,55.3949867289221));
#23818=CARTESIAN_POINT('Ctrl Pts',(1.90585575589902,-3.44037829863324,55.4008438489879));
#23819=CARTESIAN_POINT('Ctrl Pts',(2.01258389972579,-3.38125443794923,55.4070004028187));
#23820=CARTESIAN_POINT('Ctrl Pts',(2.11651218828637,-3.31718506977655,55.4131569566495));
#23821=CARTESIAN_POINT('Ctrl Pts',(2.2171691653615,-3.24848424533199,55.4193135104803));
#23822=CARTESIAN_POINT('Ctrl Pts',(2.31307320469071,-3.183027416,55.4251793570205));
#23823=CARTESIAN_POINT('Ctrl Pts',(2.40600750894773,-3.11336682291932,55.4310452035606));
#23824=CARTESIAN_POINT('Ctrl Pts',(2.49559762194041,-3.03981603215809,55.4369110501008));
#23825=CARTESIAN_POINT('Ctrl Pts',(2.58524933476359,-2.96621466978696,55.4427809298444));
#23826=CARTESIAN_POINT('Ctrl Pts',(2.67155197165439,-2.88871805843014,55.4486508095881));
#23827=CARTESIAN_POINT('Ctrl Pts',(2.7541674591796,-2.80767708378227,55.4545206893317));
#23828=CARTESIAN_POINT('Ctrl Pts',(2.83690009587701,-2.7265211926293,55.460398892594));
#23829=CARTESIAN_POINT('Ctrl Pts',(2.91593487038186,-2.64181120977399,55.4662770958563));
#23830=CARTESIAN_POINT('Ctrl Pts',(2.99097353195254,-2.55393154394539,55.4721552991186));
#23831=CARTESIAN_POINT('Ctrl Pts',(3.0018974447618,-2.54113827462096,55.4730110310649));
#23832=CARTESIAN_POINT('Ctrl Pts',(3.01273674403921,-2.52827788128809,55.4738667630112));
#23833=CARTESIAN_POINT('Ctrl Pts',(3.02349058702999,-2.51535159970549,55.4747224949575));
#23834=CARTESIAN_POINT('Ctrl Pts',(3.09735158361245,-2.42656956702987,55.4805999486653));
#23835=CARTESIAN_POINT('Ctrl Pts',(3.16741983797865,-2.33438595917166,55.4864774023732));
#23836=CARTESIAN_POINT('Ctrl Pts',(3.23336643838967,-2.23915843010164,55.4923548560811));
#23837=CARTESIAN_POINT('Ctrl Pts',(3.29922875801771,-2.14405260329771,55.4982247983115));
#23838=CARTESIAN_POINT('Ctrl Pts',(3.36097966677623,-2.04591092800972,55.5040947405419));
#23839=CARTESIAN_POINT('Ctrl Pts',(3.41832971213729,-1.94512492635288,55.5099646827724));
#23840=CARTESIAN_POINT('Ctrl Pts',(3.475621722804,-1.84444091388829,55.5158286849848));
#23841=CARTESIAN_POINT('Ctrl Pts',(3.52852152580334,-1.74111825431264,55.5216926871972));
#23842=CARTESIAN_POINT('Ctrl Pts',(3.57678268341861,-1.63557776812864,55.5275566894096));
#23843=CARTESIAN_POINT('Ctrl Pts',(3.62639507325392,-1.52708232370292,55.5335848739401));
#23844=CARTESIAN_POINT('Ctrl Pts',(3.67110497330673,-1.41624338886802,55.5396130584705));
#23845=CARTESIAN_POINT('Ctrl Pts',(3.71069491913246,-1.30354601649673,55.545641243001));
#23846=CARTESIAN_POINT('Ctrl Pts',(3.74916324983053,-1.19404145166942,55.5514986441969));
#23847=CARTESIAN_POINT('Ctrl Pts',(3.78279769085203,-1.08278275245442,55.5573560453928));
#23848=CARTESIAN_POINT('Ctrl Pts',(3.81144767707452,-0.970234819475773,
55.5632134465887));
#23849=CARTESIAN_POINT('Ctrl Pts',(3.8400935248378,-0.857703143923043,55.5690700016895));
#23850=CARTESIAN_POINT('Ctrl Pts',(3.86375624780682,-0.743883004576842,
55.5749265567902));
#23851=CARTESIAN_POINT('Ctrl Pts',(3.88233561911942,-0.629252843073858,
55.5807831118909));
#23852=CARTESIAN_POINT('Ctrl Pts',(3.9009167827119,-0.514611623643904,55.5866402319508));
#23853=CARTESIAN_POINT('Ctrl Pts',(3.91441355383479,-0.399160633925395,
55.5924973520106));
#23854=CARTESIAN_POINT('Ctrl Pts',(3.92277724186476,-0.283386151227936,
55.5983544720705));
#23855=CARTESIAN_POINT('Ctrl Pts',(3.93156850704697,-0.161692925096254,
55.6045110259097));
#23856=CARTESIAN_POINT('Ctrl Pts',(3.93468792686195,-0.0396427617862714,
55.6106675797488));
#23857=CARTESIAN_POINT('Ctrl Pts',(3.93214095724448,0.0821978853767393,
55.616824133588));
#23858=CARTESIAN_POINT('Ctrl Pts',(3.92971425339454,0.198285319447808,55.6226899801223));
#23859=CARTESIAN_POINT('Ctrl Pts',(3.92214414325636,0.314182155224603,55.6285558266567));
#23860=CARTESIAN_POINT('Ctrl Pts',(3.90948867235328,0.429403447519139,55.6344216731911));
#23861=CARTESIAN_POINT('Ctrl Pts',(3.89682449987763,0.544703962976815,55.6402915529289));
#23862=CARTESIAN_POINT('Ctrl Pts',(3.87906806714342,0.659327603541924,55.6461614326668));
#23863=CARTESIAN_POINT('Ctrl Pts',(3.85632855470308,0.77279950710489,55.6520313124047));
#23864=CARTESIAN_POINT('Ctrl Pts',(3.83355679752063,0.886432314393349,55.6579095156613));
#23865=CARTESIAN_POINT('Ctrl Pts',(3.80578795958185,0.998909727187948,55.6637877189179));
#23866=CARTESIAN_POINT('Ctrl Pts',(3.77318105601108,1.10977192186461,55.6696659221745));
#23867=CARTESIAN_POINT('Ctrl Pts',(3.76843423641047,1.12591092253712,55.6705216541631));
#23868=CARTESIAN_POINT('Ctrl Pts',(3.76358496803087,1.1420157277089,55.6713773861517));
#23869=CARTESIAN_POINT('Ctrl Pts',(3.75863382545225,1.15808495636809,55.6722331181403));
#23870=CARTESIAN_POINT('Ctrl Pts',(3.72462772109122,1.26845379711713,55.6781105718487));
#23871=CARTESIAN_POINT('Ctrl Pts',(3.6857004396103,1.37750444857909,55.6839880255571));
#23872=CARTESIAN_POINT('Ctrl Pts',(3.64197183586831,1.4847660242415,55.6898654792655));
#23873=CARTESIAN_POINT('Ctrl Pts',(3.59829911796362,1.59189051793806,55.6957354214964));
#23874=CARTESIAN_POINT('Ctrl Pts',(3.54983743547528,1.69723010447361,55.7016053637274));
#23875=CARTESIAN_POINT('Ctrl Pts',(3.49675656829594,1.80032844283455,55.7074753059583));
#23876=CARTESIAN_POINT('Ctrl Pts',(3.44372941566734,1.90332245206109,55.7133393081712));
#23877=CARTESIAN_POINT('Ctrl Pts',(3.38609256410601,2.00407935992187,55.7192033103841));
#23878=CARTESIAN_POINT('Ctrl Pts',(3.32406383370634,2.10216284560579,55.7250673125969));
#23879=CARTESIAN_POINT('Ctrl Pts',(3.26029840193243,2.20299250589752,55.7310954971272));
#23880=CARTESIAN_POINT('Ctrl Pts',(3.1918916894103,2.30099641560372,55.7371236816575));
#23881=CARTESIAN_POINT('Ctrl Pts',(3.11913114405559,2.3957274273553,55.7431518661877));
#23882=CARTESIAN_POINT('Ctrl Pts',(3.04843196368654,2.48777463307257,55.749009267384));
#23883=CARTESIAN_POINT('Ctrl Pts',(2.97362260159842,2.57673155027685,55.7548666685803));
#23884=CARTESIAN_POINT('Ctrl Pts',(2.89501017746513,2.66221807378232,55.7607240697766));
#23885=CARTESIAN_POINT('Ctrl Pts',(2.81640910881105,2.7476922488524,55.7665806248776));
#23886=CARTESIAN_POINT('Ctrl Pts',(2.7340063496535,2.82969672350588,55.7724371799787));
#23887=CARTESIAN_POINT('Ctrl Pts',(2.6481478633288,2.9078861556029,55.7782937350797));
#23888=CARTESIAN_POINT('Ctrl Pts',(2.56228109456958,2.9860831303306,55.7841508551399));
#23889=CARTESIAN_POINT('Ctrl Pts',(2.47295824094942,3.06046405315319,55.7900079752));
#23890=CARTESIAN_POINT('Ctrl Pts',(2.38055998543373,3.13072246546252,55.7958650952602));
#23891=CARTESIAN_POINT('Ctrl Pts',(2.28343805027946,3.20457270133834,55.8020216490988));
#23892=CARTESIAN_POINT('Ctrl Pts',(2.18291834923423,3.2738674546978,55.8081782029373));
#23893=CARTESIAN_POINT('Ctrl Pts',(2.07947830021533,3.33830181363722,55.8143347567759));
#23894=CARTESIAN_POINT('Ctrl Pts',(1.98092260347625,3.39969363623825,55.8202006033105));
#23895=CARTESIAN_POINT('Ctrl Pts',(1.87971644562286,3.45667342848559,55.8260664498451));
#23896=CARTESIAN_POINT('Ctrl Pts',(1.77629770914611,3.50902485720495,55.8319322963796));
#23897=CARTESIAN_POINT('Ctrl Pts',(1.67280786463709,3.56141228140453,55.8378021761177));
#23898=CARTESIAN_POINT('Ctrl Pts',(1.56710278710126,3.60916483593996,55.8436720558557));
#23899=CARTESIAN_POINT('Ctrl Pts',(1.45963985147843,3.6521145250356,55.8495419355937));
#23900=CARTESIAN_POINT('Ctrl Pts',(1.35202453287753,3.69512511700434,55.8554201388504));
#23901=CARTESIAN_POINT('Ctrl Pts',(1.24264677007972,3.73331911858355,55.8612983421072));
#23902=CARTESIAN_POINT('Ctrl Pts',(1.1319785695324,3.76657848957371,55.8671765453639));
#23903=CARTESIAN_POINT('Ctrl Pts',(1.11586781001058,3.77142029349949,55.8680322773503));
#23904=CARTESIAN_POINT('Ctrl Pts',(1.09972971832541,3.77615760801281,55.8688880093368));
#23905=CARTESIAN_POINT('Ctrl Pts',(1.08356576507486,3.78079015984195,55.8697437413232));
#23906=CARTESIAN_POINT('Ctrl Pts',(0.972546323557523,3.81260807646786,55.8756211950469));
#23907=CARTESIAN_POINT('Ctrl Pts',(0.859942257719565,3.83958403344108,55.8814986487706));
#23908=CARTESIAN_POINT('Ctrl Pts',(0.746213444616676,3.86156114739535,55.8873761024944));
#23909=CARTESIAN_POINT('Ctrl Pts',(0.632629978708228,3.8835101742557,55.8932460447407));
#23910=CARTESIAN_POINT('Ctrl Pts',(0.517925025673935,3.900472985893,55.899115986987));
#23911=CARTESIAN_POINT('Ctrl Pts',(0.402573556405177,3.91234246094118,55.9049859292333));
#23912=CARTESIAN_POINT('Ctrl Pts',(0.287338815679251,3.92419992481573,55.9108499314616));
#23913=CARTESIAN_POINT('Ctrl Pts',(0.17145926806963,3.93097426257382,55.9167139336899));
#23914=CARTESIAN_POINT('Ctrl Pts',(0.0554193631486505,3.93260952729714,
55.9225779359182));
#23915=CARTESIAN_POINT('Ctrl Pts',(-0.0638694658513173,3.93429057670925,
55.9286061204427));
#23916=CARTESIAN_POINT('Ctrl Pts',(-0.183327329042966,3.9305404401863,55.9346343049672));
#23917=CARTESIAN_POINT('Ctrl Pts',(-0.302422667863923,3.92135557300815,
55.9406624894917));
#23918=CARTESIAN_POINT('Ctrl Pts',(-0.41814394001257,3.91243092049954,55.9465198907035));
#23919=CARTESIAN_POINT('Ctrl Pts',(-0.533522514949512,3.89837537764589,
55.9523772919152));
#23920=CARTESIAN_POINT('Ctrl Pts',(-0.648072238113552,3.87923850442152,
55.9582346931269));
#23921=CARTESIAN_POINT('Ctrl Pts',(-0.762605414694159,3.86010439549776,
55.9640912482434));
#23922=CARTESIAN_POINT('Ctrl Pts',(-0.876309570824094,3.83589048372245,
55.9699478033599));
#23923=CARTESIAN_POINT('Ctrl Pts',(-0.988706445761817,3.8066978556367,55.9758043584763));
#23924=CARTESIAN_POINT('Ctrl Pts',(-1.10111416318871,3.77750241145172,55.9816614785519));
#23925=CARTESIAN_POINT('Ctrl Pts',(-1.21221394946203,3.74332739991008,55.9875185986274));
#23926=CARTESIAN_POINT('Ctrl Pts',(-1.32154114196649,3.70432423123165,55.993375718703));
#23927=CARTESIAN_POINT('Ctrl Pts',(-1.43645747211256,3.66332710228396,55.9995322725199));
#23928=CARTESIAN_POINT('Ctrl Pts',(-1.54941469313502,3.61699526388156,56.0056888263368));
#23929=CARTESIAN_POINT('Ctrl Pts',(-1.65989658677665,3.56556199233827,56.0118453801538));
#23930=CARTESIAN_POINT('Ctrl Pts',(-1.76516161878899,3.51655735640159,56.0177112267035));
#23931=CARTESIAN_POINT('Ctrl Pts',(-1.86817940136615,3.46292229648925,56.0235770732532));
#23932=CARTESIAN_POINT('Ctrl Pts',(-1.96852950616077,3.40490537069307,56.0294429198029));
#23933=CARTESIAN_POINT('Ctrl Pts',(-2.06894860907477,3.34684855396921,56.035312799556));
#23934=CARTESIAN_POINT('Ctrl Pts',(-2.16669603517733,3.2844040935218,56.0411826793091));
#23935=CARTESIAN_POINT('Ctrl Pts',(-2.26138119176589,3.21786328260346,56.0470525590622));
#23936=CARTESIAN_POINT('Ctrl Pts',(-2.35620061237455,3.15122811648631,56.0529307623338));
#23937=CARTESIAN_POINT('Ctrl Pts',(-2.44794877365813,3.08048526014792,56.0588089656054));
#23938=CARTESIAN_POINT('Ctrl Pts',(-2.53626892964854,3.00596555477595,56.064687168877));
#23939=CARTESIAN_POINT('Ctrl Pts',(-2.54912632319468,2.99511719102291,56.0655429007533));
#23940=CARTESIAN_POINT('Ctrl Pts',(-2.56191113381532,2.98418884728861,56.0663986326297));
#23941=CARTESIAN_POINT('Ctrl Pts',(-2.57462232916952,2.97318160598067,56.0672543645061));
#23942=CARTESIAN_POINT('Ctrl Pts',(-2.66068396062302,2.89865666018549,56.0730481297119));
#23943=CARTESIAN_POINT('Ctrl Pts',(-2.74366779970919,2.82025249851762,56.0788418949177));
#23944=CARTESIAN_POINT('Ctrl Pts',(-2.82319664746214,2.73825668806973,56.0846356601235));
#23945=CARTESIAN_POINT('Ctrl Pts',(-2.90262312396697,2.65636642439754,56.0904219674697));
#23946=CARTESIAN_POINT('Ctrl Pts',(-2.97860315528158,2.57089400348787,56.096208274816));
#23947=CARTESIAN_POINT('Ctrl Pts',(-3.05079247440205,2.48216725426227,56.1019945821623));
#23948=CARTESIAN_POINT('Ctrl Pts',(-3.12290181329056,2.39353880747351,56.1077744787235));
#23949=CARTESIAN_POINT('Ctrl Pts',(-3.19122852740523,2.301663532516,56.1135543752848));
#23950=CARTESIAN_POINT('Ctrl Pts',(-3.2554657983641,2.20690539799096,56.1193342718461));
#23951=CARTESIAN_POINT('Ctrl Pts',(-3.31966367911436,2.11220536902725,56.1251106241825));
#23952=CARTESIAN_POINT('Ctrl Pts',(-3.37977686097575,2.01462634359139,56.1308869765189));
#23953=CARTESIAN_POINT('Ctrl Pts',(-3.43553970410726,1.91456416489567,56.1366633288554));
#23954=CARTESIAN_POINT('Ctrl Pts',(-3.49128270802699,1.81453758615581,56.1424376260907));
#23955=CARTESIAN_POINT('Ctrl Pts',(-3.54267824260044,1.71202998119307,56.1482119233261));
#23956=CARTESIAN_POINT('Ctrl Pts',(-3.58950526741073,1.60746413186443,56.1539862205615));
#23957=CARTESIAN_POINT('Ctrl Pts',(-3.6363276851416,1.50290857025266,56.1597599496923));
#23958=CARTESIAN_POINT('Ctrl Pts',(-3.67858231408159,1.39629555558776,56.1655336788232));
#23959=CARTESIAN_POINT('Ctrl Pts',(-3.71609552636559,1.28806950081343,56.171307407954));
#23960=CARTESIAN_POINT('Ctrl Pts',(-3.75363352304202,1.17977194277798,56.1770849516973));
#23961=CARTESIAN_POINT('Ctrl Pts',(-3.78642370412774,1.06985961776369,56.1828624954407));
#23962=CARTESIAN_POINT('Ctrl Pts',(-3.81434184516174,0.958793663020485,
56.188640039184));
#23963=CARTESIAN_POINT('Ctrl Pts',(-3.84226902337821,0.847691755908585,
56.1944194531349));
#23964=CARTESIAN_POINT('Ctrl Pts',(-3.86532093285606,0.735435891859941,
56.2001988670857));
#23965=CARTESIAN_POINT('Ctrl Pts',(-3.88342453340857,0.622497303866083,
56.2059782810366));
#23966=CARTESIAN_POINT('Ctrl Pts',(-3.90155186064883,0.509410697879598,
56.2117652695221));
#23967=CARTESIAN_POINT('Ctrl Pts',(-3.91471787359035,0.395640003337236,
56.2175522580076));
#23968=CARTESIAN_POINT('Ctrl Pts',(-3.92290144284473,0.281661622744134,
56.2233392464932));
#23969=CARTESIAN_POINT('Ctrl Pts',(-3.92970478800912,0.186906603222668,
56.2281502133104));
#23970=CARTESIAN_POINT('Ctrl Pts',(-3.93306556565048,0.0920082219184449,
56.2329611801277));
#23971=CARTESIAN_POINT('Ctrl Pts',(-3.93299903070378,-0.00276124668366241,
56.2377721469449));
#23972=CARTESIAN_POINT('',(-3.93299858145448,0.00334040074976491,57.4877721470256));
#23973=CARTESIAN_POINT('Ctrl Pts',(-3.93299903070322,-0.00276124747559212,
56.2377721469851));
#23974=CARTESIAN_POINT('Ctrl Pts',(-3.93287459502664,-0.180001932956672,
56.246769760553));
#23975=CARTESIAN_POINT('Ctrl Pts',(-3.92076827578561,-0.356823248188878,
56.2557673741209));
#23976=CARTESIAN_POINT('Ctrl Pts',(-3.89685364668713,-0.53199685741675,
56.2647649876888));
#23977=CARTESIAN_POINT('Ctrl Pts',(-3.88123204610195,-0.646424396524865,
56.2706424413929));
#23978=CARTESIAN_POINT('Ctrl Pts',(-3.86054048287139,-0.760350850911274,
56.2765198950971));
#23979=CARTESIAN_POINT('Ctrl Pts',(-3.83482071000186,-0.873292117301467,
56.2823973488012));
#23980=CARTESIAN_POINT('Ctrl Pts',(-3.80913380740383,-0.98608904298896,
56.2882672910277));
#23981=CARTESIAN_POINT('Ctrl Pts',(-3.7784315659522,-1.09790288606155,56.2941372332542));
#23982=CARTESIAN_POINT('Ctrl Pts',(-3.74280736362221,-1.20825578368798,
56.3000071754807));
#23983=CARTESIAN_POINT('Ctrl Pts',(-3.70721921078017,-1.31849701101181,
56.305871177689));
#23984=CARTESIAN_POINT('Ctrl Pts',(-3.66671913054122,-1.42727984335804,
56.3117351798972));
#23985=CARTESIAN_POINT('Ctrl Pts',(-3.62145115558799,-1.53413836654014,
56.3175991821055));
#23986=CARTESIAN_POINT('Ctrl Pts',(-3.57491575251127,-1.64398875091456,
56.3236273666374));
#23987=CARTESIAN_POINT('Ctrl Pts',(-3.52334161667332,-1.7518050444529,56.3296555511693));
#23988=CARTESIAN_POINT('Ctrl Pts',(-3.46693972427375,-1.85709933720648,
56.3356837357013));
#23989=CARTESIAN_POINT('Ctrl Pts',(-3.41213574307814,-1.95941055753205,
56.3415411368925));
#23990=CARTESIAN_POINT('Ctrl Pts',(-3.35277408902343,-2.05934037178854,
56.3473985380838));
#23991=CARTESIAN_POINT('Ctrl Pts',(-3.28909604162208,-2.15646382510489,
56.3532559392751));
#23992=CARTESIAN_POINT('Ctrl Pts',(-3.225427192447,-2.25357324904165,56.359112494371));
#23993=CARTESIAN_POINT('Ctrl Pts',(-3.15744341588601,-2.3478767732614,56.3649690494669));
#23994=CARTESIAN_POINT('Ctrl Pts',(-3.08542996722739,-2.43897743272365,
56.3708256045628));
#23995=CARTESIAN_POINT('Ctrl Pts',(-3.01340957171283,-2.53008688031048,
56.3766827246177));
#23996=CARTESIAN_POINT('Ctrl Pts',(-2.93735898716203,-2.61799252532131,
56.3825398446726));
#23997=CARTESIAN_POINT('Ctrl Pts',(-2.85760404489878,-2.70233012834816,
56.3883969647275));
#23998=CARTESIAN_POINT('Ctrl Pts',(-2.77377178742812,-2.79097932613792,
56.3945535185728));
#23999=CARTESIAN_POINT('Ctrl Pts',(-2.68584674290883,-2.87568564067674,
56.4007100724182));
#24000=CARTESIAN_POINT('Ctrl Pts',(-2.59425044351078,-2.95607064129804,
56.4068666262636));
#24001=CARTESIAN_POINT('Ctrl Pts',(-2.50697924465678,-3.03265992951386,
56.4127324727926));
#24002=CARTESIAN_POINT('Ctrl Pts',(-2.4163759413284,-3.10532645905232,56.4185983193216));
#24003=CARTESIAN_POINT('Ctrl Pts',(-2.32283744780661,-3.17378562462359,
56.4244641658506));
#24004=CARTESIAN_POINT('Ctrl Pts',(-2.22923463965204,-3.24229186093471,
56.430334045583));
#24005=CARTESIAN_POINT('Ctrl Pts',(-2.13269296506131,-3.30658474488133,
56.4362039253154));
#24006=CARTESIAN_POINT('Ctrl Pts',(-2.0336364255655,-3.36642419914859,56.4420738050477));
#24007=CARTESIAN_POINT('Ctrl Pts',(-1.93443942340472,-3.42634850605919,
56.4479520082987));
#24008=CARTESIAN_POINT('Ctrl Pts',(-1.83272080115182,-3.4818065858652,56.4538302115497));
#24009=CARTESIAN_POINT('Ctrl Pts',(-1.728927114159,-3.53260527570317,56.4597084148006));
#24010=CARTESIAN_POINT('Ctrl Pts',(-1.71381712594818,-3.54000040373856,
56.4605641468244));
#24011=CARTESIAN_POINT('Ctrl Pts',(-1.69866319141438,-3.54729687171511,
56.4614198788481));
#24012=CARTESIAN_POINT('Ctrl Pts',(-1.68346671721348,-3.55449417105085,
56.4622756108719));
#24013=CARTESIAN_POINT('Ctrl Pts',(-1.57909224872148,-3.60392763060304,
56.4681530646793));
#24014=CARTESIAN_POINT('Ctrl Pts',(-1.4723674951303,-3.64884093872592,56.4740305184866));
#24015=CARTESIAN_POINT('Ctrl Pts',(-1.36372073238838,-3.68900457631244,
56.479907972294));
#24016=CARTESIAN_POINT('Ctrl Pts',(-1.25521282189451,-3.72911688414713,
56.4857779146242));
#24017=CARTESIAN_POINT('Ctrl Pts',(-1.14478817082094,-3.76449145173836,
56.4916478569545));
#24018=CARTESIAN_POINT('Ctrl Pts',(-1.0328980336689,-3.79494540830866,56.4975177992847));
#24019=CARTESIAN_POINT('Ctrl Pts',(-0.921121122401242,-3.82536854736229,
56.5033818015971));
#24020=CARTESIAN_POINT('Ctrl Pts',(-0.807882070680306,-3.85088087245687,
56.5092458039095));
#24021=CARTESIAN_POINT('Ctrl Pts',(-0.69364980051294,-3.87134846716856,
56.5151098062218));
#24022=CARTESIAN_POINT('Ctrl Pts',(-0.576219219325438,-3.89238912003296,
56.5211379907149));
#24023=CARTESIAN_POINT('Ctrl Pts',(-0.457739395909401,-3.90809822122731,
56.5271661752079));
#24024=CARTESIAN_POINT('Ctrl Pts',(-0.338734249508409,-3.91838590598348,
56.5331943597009));
#24025=CARTESIAN_POINT('Ctrl Pts',(-0.223100612295275,-3.92838213255716,
56.5390517609966));
#24026=CARTESIAN_POINT('Ctrl Pts',(-0.106971456081406,-3.93325996686306,
56.5449091622923));
#24027=CARTESIAN_POINT('Ctrl Pts',(0.00916547212947215,-3.93298932036697,
56.550766563588));
#24028=CARTESIAN_POINT('Ctrl Pts',(0.125285624483332,-3.93271871296548,
56.5566231187882));
#24029=CARTESIAN_POINT('Ctrl Pts',(0.241413134207897,-3.92730110457721,
56.5624796739884));
#24030=CARTESIAN_POINT('Ctrl Pts',(0.357059671235795,-3.91675853112966,
56.5683362291887));
#24031=CARTESIAN_POINT('Ctrl Pts',(0.472717364229187,-3.90621494068162,
56.5741933493477));
#24032=CARTESIAN_POINT('Ctrl Pts',(0.587893581478536,-3.89054543983216,
56.5800504695067));
#24033=CARTESIAN_POINT('Ctrl Pts',(0.702105233804478,-3.86982392889707,
56.5859075896657));
#24034=CARTESIAN_POINT('Ctrl Pts',(0.822155728162672,-3.84804307220736,
56.5920641433648));
#24035=CARTESIAN_POINT('Ctrl Pts',(0.941139924894108,-3.8206800797011,56.5982206970638));
#24036=CARTESIAN_POINT('Ctrl Pts',(1.05851056277257,-3.78788125322044,56.6043772507629));
#24037=CARTESIAN_POINT('Ctrl Pts',(1.1703390620456,-3.7566311585669,56.6102430973946));
#24038=CARTESIAN_POINT('Ctrl Pts',(1.28070252045885,-3.72044703788001,56.6161089440264));
#24039=CARTESIAN_POINT('Ctrl Pts',(1.38914571081522,-3.67950583558766,56.6219747906581));
#24040=CARTESIAN_POINT('Ctrl Pts',(1.49766346387512,-3.63853648319461,56.6278446704926));
#24041=CARTESIAN_POINT('Ctrl Pts',(1.6042579417669,-3.59280369837456,56.6337145503272));
#24042=CARTESIAN_POINT('Ctrl Pts',(1.70849641291049,-3.54253144051989,56.6395844301617));
#24043=CARTESIAN_POINT('Ctrl Pts',(1.81288269469777,-3.49218789636649,56.6454626335136));
#24044=CARTESIAN_POINT('Ctrl Pts',(1.91490594185586,-3.43729222945618,56.6513408368654));
#24045=CARTESIAN_POINT('Ctrl Pts',(2.0141603940696,-3.37811292099026,56.6572190402173));
#24046=CARTESIAN_POINT('Ctrl Pts',(2.0286095606375,-3.36949777409936,56.6580747714964));
#24047=CARTESIAN_POINT('Ctrl Pts',(2.04300010392026,-3.36079191692025,56.6589305027755));
#24048=CARTESIAN_POINT('Ctrl Pts',(2.05733082942857,-3.35199624974174,56.6597862340546));
#24049=CARTESIAN_POINT('Ctrl Pts',(2.15575912719411,-3.29158461548147,56.6656636875792));
#24050=CARTESIAN_POINT('Ctrl Pts',(2.25168561722266,-3.22673490030129,56.6715411411037));
#24051=CARTESIAN_POINT('Ctrl Pts',(2.34468407574939,-3.1576804120948,56.6774185946283));
#24052=CARTESIAN_POINT('Ctrl Pts',(2.43756368079638,-3.08871417660072,56.6832885366756));
#24053=CARTESIAN_POINT('Ctrl Pts',(2.52752236816214,-3.01555409892089,56.6891584787229));
#24054=CARTESIAN_POINT('Ctrl Pts',(2.61416043040077,-2.93847821910029,56.6950284207702));
#24055=CARTESIAN_POINT('Ctrl Pts',(2.70071082028906,-2.86148033529396,56.7008924228));
#24056=CARTESIAN_POINT('Ctrl Pts',(2.78394696276826,-2.78057480411996,56.7067564248297));
#24057=CARTESIAN_POINT('Ctrl Pts',(2.86350049982774,-2.69608120936411,56.7126204268594));
#24058=CARTESIAN_POINT('Ctrl Pts',(2.94528140721404,-2.60922193065852,56.7186486114585));
#24059=CARTESIAN_POINT('Ctrl Pts',(3.02317008802361,-2.51857096006013,56.7246767960576));
#24060=CARTESIAN_POINT('Ctrl Pts',(3.09680503223868,-2.42451801236888,56.7307049806566));
#24061=CARTESIAN_POINT('Ctrl Pts',(3.16835383601571,-2.33312966447581,56.736562381672));
#24062=CARTESIAN_POINT('Ctrl Pts',(3.23588642041773,-2.23852985960576,56.7424197826874));
#24063=CARTESIAN_POINT('Ctrl Pts',(3.29911110420297,-2.14111067488922,56.7482771837027));
#24064=CARTESIAN_POINT('Ctrl Pts',(3.36232665526344,-2.0437055622494,56.754133738624));
#24065=CARTESIAN_POINT('Ctrl Pts',(3.42123531860403,-1.94348222553152,56.7599902935453));
#24066=CARTESIAN_POINT('Ctrl Pts',(3.47558875164533,-1.84086170839539,56.7658468484666));
#24067=CARTESIAN_POINT('Ctrl Pts',(3.52994742796367,-1.738231291833,56.7717039683483));
#24068=CARTESIAN_POINT('Ctrl Pts',(3.57974980736229,-1.63320359969469,56.7775610882301));
#24069=CARTESIAN_POINT('Ctrl Pts',(3.62479385001183,-1.52622362218527,56.7834182081118));
#24070=CARTESIAN_POINT('Ctrl Pts',(3.67214068442458,-1.41377449500485,56.7895747622056));
#24071=CARTESIAN_POINT('Ctrl Pts',(3.71422958870528,-1.29916865495173,56.7957313162994));
#24072=CARTESIAN_POINT('Ctrl Pts',(3.75088410301986,-1.1829443967122,56.8018878703932));
#24073=CARTESIAN_POINT('Ctrl Pts',(3.78580781945848,-1.07220815824482,56.8077537167543));
#24074=CARTESIAN_POINT('Ctrl Pts',(3.81579858269825,-0.960003272196668,
56.8136195631155));
#24075=CARTESIAN_POINT('Ctrl Pts',(3.84075588063964,-0.846807690879045,
56.8194854094766));
#24076=CARTESIAN_POINT('Ctrl Pts',(3.8657303385776,-0.733534279189309,56.8253552890429));
#24077=CARTESIAN_POINT('Ctrl Pts',(3.88566436910299,-0.619269221088189,
56.8312251686093));
#24078=CARTESIAN_POINT('Ctrl Pts',(3.90050912831131,-0.504497314125691,
56.8370950481756));
#24079=CARTESIAN_POINT('Ctrl Pts',(3.91537493747158,-0.389562659954418,
56.8429732512641));
#24080=CARTESIAN_POINT('Ctrl Pts',(3.92513704076069,-0.27412013200252,56.8488514543526));
#24081=CARTESIAN_POINT('Ctrl Pts',(3.92979861957694,-0.158656262312916,
56.8547296574411));
#24082=CARTESIAN_POINT('Ctrl Pts',(3.93047723989724,-0.141847337414223,
56.8555853907066));
#24083=CARTESIAN_POINT('Ctrl Pts',(3.93104785585078,-0.125037953337633,
56.8564411239721));
#24084=CARTESIAN_POINT('Ctrl Pts',(3.931510568873,-0.108229602419195,56.8572968572375));
#24085=CARTESIAN_POINT('Ctrl Pts',(3.93468863204792,0.00721560555963267,
56.8631743109679));
#24086=CARTESIAN_POINT('Ctrl Pts',(3.93278268651428,0.122990150236636,56.8690517646983));
#24087=CARTESIAN_POINT('Ctrl Pts',(3.92575527379227,0.238609577117339,56.8749292184287));
#24088=CARTESIAN_POINT('Ctrl Pts',(3.91873684221516,0.354081240536956,56.8807991606801));
#24089=CARTESIAN_POINT('Ctrl Pts',(3.90660998529077,0.46939777233163,56.8866691029314));
#24090=CARTESIAN_POINT('Ctrl Pts',(3.88938919745631,0.584072487547633,56.8925390451827));
#24091=CARTESIAN_POINT('Ctrl Pts',(3.87218583599748,0.69863115902154,56.8984030474144));
#24092=CARTESIAN_POINT('Ctrl Pts',(3.84989885818527,0.812548900263899,56.904267049646));
#24093=CARTESIAN_POINT('Ctrl Pts',(3.82259468146891,0.925342585859694,56.9101310518776));
#24094=CARTESIAN_POINT('Ctrl Pts',(3.79452603330295,1.04129430669781,56.9161592364003));
#24095=CARTESIAN_POINT('Ctrl Pts',(3.7611551099159,1.1560576545347,56.9221874209229));
#24096=CARTESIAN_POINT('Ctrl Pts',(3.72261080887317,1.2691169235577,56.9282156054455));
#24097=CARTESIAN_POINT('Ctrl Pts',(3.68515849885229,1.37897313263744,56.9340730066565));
#24098=CARTESIAN_POINT('Ctrl Pts',(3.64282214965559,1.487220106419,56.9399304078675));
#24099=CARTESIAN_POINT('Ctrl Pts',(3.59577078837762,1.59339933395558,56.9457878090785));
#24100=CARTESIAN_POINT('Ctrl Pts',(3.5487262236299,1.69956322399052,56.9516443641927));
#24101=CARTESIAN_POINT('Ctrl Pts',(3.49696816822327,1.80365958468784,56.9575009193069));
#24102=CARTESIAN_POINT('Ctrl Pts',(3.44071358844026,1.90525037785653,56.9633574744211));
#24103=CARTESIAN_POINT('Ctrl Pts',(3.38445358201128,2.00685097106765,56.9692145944929));
#24104=CARTESIAN_POINT('Ctrl Pts',(3.3236963887626,2.10594515538632,56.9750717145647));
#24105=CARTESIAN_POINT('Ctrl Pts',(3.25870432906919,2.20212059063659,56.9809288346365));
#24106=CARTESIAN_POINT('Ctrl Pts',(3.19038967815428,2.30321280585034,56.9870853884518));
#24107=CARTESIAN_POINT('Ctrl Pts',(3.11739598910982,2.4010795233256,56.9932419422672));
#24108=CARTESIAN_POINT('Ctrl Pts',(3.04007770569127,2.49527885082185,56.9993984960825));
#24109=CARTESIAN_POINT('Ctrl Pts',(2.96641032633423,2.58503016560828,57.0052643426248));
#24110=CARTESIAN_POINT('Ctrl Pts',(2.88881775321142,2.67145224474171,57.0111301891671));
#24111=CARTESIAN_POINT('Ctrl Pts',(2.80764538398454,2.75419977448809,57.0169960357093));
#24112=CARTESIAN_POINT('Ctrl Pts',(2.72641720276739,2.83700419926377,57.0228659154537));
#24113=CARTESIAN_POINT('Ctrl Pts',(2.64160462506545,2.9161287631432,57.0287357951981));
#24114=CARTESIAN_POINT('Ctrl Pts',(2.55358701072106,2.99126768756603,57.0346056749425));
#24115=CARTESIAN_POINT('Ctrl Pts',(2.46544458699009,3.06651315933323,57.0404838782037));
#24116=CARTESIAN_POINT('Ctrl Pts',(2.37408838188039,3.13776146185018,57.0463620814648));
#24117=CARTESIAN_POINT('Ctrl Pts',(2.27992763197877,3.20474944308282,57.052240284726));
#24118=CARTESIAN_POINT('Ctrl Pts',(2.26621998124525,3.21450136042672,57.0530960166241));
#24119=CARTESIAN_POINT('Ctrl Pts',(2.25245293796707,3.22416306909368,57.0539517485223));
#24120=CARTESIAN_POINT('Ctrl Pts',(2.23862780747392,3.23373383870789,57.0548074804205));
#24121=CARTESIAN_POINT('Ctrl Pts',(2.14367216270103,3.29946910248276,57.0606849348273));
#24122=CARTESIAN_POINT('Ctrl Pts',(2.04566303290193,3.36112614987088,57.0665623892341));
#24123=CARTESIAN_POINT('Ctrl Pts',(1.94498571113632,3.41840892572488,57.0724398436409));
#24124=CARTESIAN_POINT('Ctrl Pts',(1.84443705649401,3.4756184933344,57.078309786573));
#24125=CARTESIAN_POINT('Ctrl Pts',(1.74122734686845,3.52846470513796,57.0841797295052));
#24126=CARTESIAN_POINT('Ctrl Pts',(1.63577212790531,3.57669380092399,57.0900496724373));
#24127=CARTESIAN_POINT('Ctrl Pts',(1.53042362304631,3.62487409187323,57.0959136753534));
#24128=CARTESIAN_POINT('Ctrl Pts',(1.42283450183459,3.6684463900876,57.1017776782694));
#24129=CARTESIAN_POINT('Ctrl Pts',(1.31344569670922,3.70720236860574,57.1076416811854));
#24130=CARTESIAN_POINT('Ctrl Pts',(1.20099420520583,3.74704344360462,57.1136698654528));
#24131=CARTESIAN_POINT('Ctrl Pts',(1.08664114851458,3.78179429297267,57.1196980497202));
#24132=CARTESIAN_POINT('Ctrl Pts',(0.970888882770561,3.81128112021568,57.1257262339876));
#24133=CARTESIAN_POINT('Ctrl Pts',(0.858415953743547,3.83993256653009,57.1315836358874));
#24134=CARTESIAN_POINT('Ctrl Pts',(0.744622458318199,3.86361414435249,57.1374410377871));
#24135=CARTESIAN_POINT('Ctrl Pts',(0.629984773635399,3.88221691627188,57.1432984396869));
#24136=CARTESIAN_POINT('Ctrl Pts',(0.515363648261151,3.9008170010379,57.1491549954903));
#24137=CARTESIAN_POINT('Ctrl Pts',(0.399898983185378,3.91433967268589,57.1550115512937));
#24138=CARTESIAN_POINT('Ctrl Pts',(0.284076199998829,3.92272733090056,57.1608681070971));
#24139=CARTESIAN_POINT('Ctrl Pts',(0.168242243876824,3.93111579823724,57.1667252278578));
#24140=CARTESIAN_POINT('Ctrl Pts',(0.0520505124086948,3.93436823762812,
57.1725823486184));
#24141=CARTESIAN_POINT('Ctrl Pts',(-0.0640103171830569,3.9324790755062,
57.1784394693791));
#24142=CARTESIAN_POINT('Ctrl Pts',(-0.186004494975884,3.93049333423077,
57.1845960222311));
#24143=CARTESIAN_POINT('Ctrl Pts',(-0.307853524419974,3.9228263832232,57.1907525750831));
#24144=CARTESIAN_POINT('Ctrl Pts',(-0.428993645620601,3.90953366170662,
57.1969091279351));
#24145=CARTESIAN_POINT('Ctrl Pts',(-0.544413664051061,3.89686860782332,
57.202774975159));
#24146=CARTESIAN_POINT('Ctrl Pts',(-0.65918978509334,3.87909705182298,57.2086408223829));
#24147=CARTESIAN_POINT('Ctrl Pts',(-0.772844080756706,3.85631962197629,
57.2145066696068));
#24148=CARTESIAN_POINT('Ctrl Pts',(-0.886576522071217,3.83352653097859,
57.2203765500302));
#24149=CARTESIAN_POINT('Ctrl Pts',(-0.999185202731103,3.80572081111499,
57.2262464304536));
#24150=CARTESIAN_POINT('Ctrl Pts',(-1.11020675248651,3.77305313595414,57.232116310877));
#24151=CARTESIAN_POINT('Ctrl Pts',(-1.22138573115095,3.74033913792649,57.2379945148095));
#24152=CARTESIAN_POINT('Ctrl Pts',(-1.33097269973614,3.70274956109741,57.2438727187419));
#24153=CARTESIAN_POINT('Ctrl Pts',(-1.43852366699403,3.66048339150693,57.2497509226744));
#24154=CARTESIAN_POINT('Ctrl Pts',(-1.45418053515729,3.65433044038137,57.2506066496507));
#24155=CARTESIAN_POINT('Ctrl Pts',(-1.4697942979821,3.6480784602632,57.2514623766269));
#24156=CARTESIAN_POINT('Ctrl Pts',(-1.48536363059346,3.64172814538788,57.2523181036032));
#24157=CARTESIAN_POINT('Ctrl Pts',(-1.59229961531961,3.59811181375283,57.2581955557168));
#24158=CARTESIAN_POINT('Ctrl Pts',(-1.69748813306968,3.54970988500913,57.2640730078305));
#24159=CARTESIAN_POINT('Ctrl Pts',(-1.8004707162327,3.49668331422629,57.2699504599441));
#24160=CARTESIAN_POINT('Ctrl Pts',(-1.90332168602245,3.44372451224123,57.2758204005808));
#24161=CARTESIAN_POINT('Ctrl Pts',(-2.00397196448123,3.38615300965328,57.2816903412176));
#24162=CARTESIAN_POINT('Ctrl Pts',(-2.10198197991541,3.32417820763432,57.2875602818543));
#24163=CARTESIAN_POINT('Ctrl Pts',(-2.19989281529583,3.26226612026926,57.2934242824753));
#24164=CARTESIAN_POINT('Ctrl Pts',(-2.29516835563841,3.19595981612733,57.2992882830963));
#24165=CARTESIAN_POINT('Ctrl Pts',(-2.38739321211389,3.12551478172038,57.3051522837174));
#24166=CARTESIAN_POINT('Ctrl Pts',(-2.48220024644996,3.05309737657536,57.3111804688452));
#24167=CARTESIAN_POINT('Ctrl Pts',(-2.57378284453499,2.97630625682685,57.3172086539731));
#24168=CARTESIAN_POINT('Ctrl Pts',(-2.66172097930895,2.89546722107274,57.323236839101));
#24169=CARTESIAN_POINT('Ctrl Pts',(-2.7471677242768,2.81691844937905,57.3290942387213));
#24170=CARTESIAN_POINT('Ctrl Pts',(-2.82917341376195,2.73454834430281,57.3349516383417));
#24171=CARTESIAN_POINT('Ctrl Pts',(-2.90738653816944,2.64869638080154,57.340809037962));
#24172=CARTESIAN_POINT('Ctrl Pts',(-2.98558836488799,2.5628568184003,57.3466655914958));
#24173=CARTESIAN_POINT('Ctrl Pts',(-3.05999843816813,2.47353670255036,57.3525221450295));
#24174=CARTESIAN_POINT('Ctrl Pts',(-3.130303304737,2.38111113145789,57.3583786985632));
#24175=CARTESIAN_POINT('Ctrl Pts',(-3.20061495346844,2.28867664426503,57.3642358170664));
#24176=CARTESIAN_POINT('Ctrl Pts',(-3.26682035849011,2.1931364346237,57.3700929355695));
#24177=CARTESIAN_POINT('Ctrl Pts',(-3.32864786319633,2.09489675230991,57.3759500540726));
#24178=CARTESIAN_POINT('Ctrl Pts',(-3.39363621856898,1.99163469416537,57.3821066101321));
#24179=CARTESIAN_POINT('Ctrl Pts',(-3.45378692888341,1.88539027559086,57.3882631661915));
#24180=CARTESIAN_POINT('Ctrl Pts',(-3.50883841719906,1.77666596803903,57.394419722251));
#24181=CARTESIAN_POINT('Ctrl Pts',(-3.56129038796504,1.67307559517643,57.4002855672686));
#24182=CARTESIAN_POINT('Ctrl Pts',(-3.60911358120336,1.56723458939839,57.4061514122863));
#24183=CARTESIAN_POINT('Ctrl Pts',(-3.65213116331708,1.45959822071976,57.4120172573039));
#24184=CARTESIAN_POINT('Ctrl Pts',(-3.69517832331094,1.3518878437995,57.417887135539));
#24185=CARTESIAN_POINT('Ctrl Pts',(-3.73341315710086,1.24238003427091,57.423757013774));
#24186=CARTESIAN_POINT('Ctrl Pts',(-3.76670870051357,1.13154521141467,57.4296268920091));
#24187=CARTESIAN_POINT('Ctrl Pts',(-3.80005145734785,1.02055322364445,57.4355050937916));
#24188=CARTESIAN_POINT('Ctrl Pts',(-3.82844084754621,0.908230865923159,
57.441383295574));
#24189=CARTESIAN_POINT('Ctrl Pts',(-3.85180095910932,0.795058721985113,
57.4472614973565));
#24190=CARTESIAN_POINT('Ctrl Pts',(-3.85520170240365,0.778583226627879,
57.4481172404998));
#24191=CARTESIAN_POINT('Ctrl Pts',(-3.85849594864675,0.762089729330191,
57.448972983643));
#24192=CARTESIAN_POINT('Ctrl Pts',(-3.8616835554484,0.745579719131035,57.4498287267862));
#24193=CARTESIAN_POINT('Ctrl Pts',(-3.89349633805213,0.580807399979073,
57.4583691686516));
#24194=CARTESIAN_POINT('Ctrl Pts',(-3.91477062463092,0.4139403465271,57.466909610517));
#24195=CARTESIAN_POINT('Ctrl Pts',(-3.92529386198954,0.246083516366632,
57.4754500523825));
#24196=CARTESIAN_POINT('Ctrl Pts',(-3.93035481505268,0.165355931326066,
57.47955741725));
#24197=CARTESIAN_POINT('Ctrl Pts',(-3.93292973557021,0.0843997468008381,
57.4836647821176));
#24198=CARTESIAN_POINT('Ctrl Pts',(-3.9329985814538,0.0033404015496607,
57.4877721469851));
#24199=CARTESIAN_POINT('',(-3.93299997598709,-0.000434609756366564,58.7377721470271));
#24200=CARTESIAN_POINT('Ctrl Pts',(-3.93299858145448,0.00334040074973609,
57.4877721470256));
#24201=CARTESIAN_POINT('Ctrl Pts',(-3.93309550525033,-0.110777988079204,
57.4935546494572));
#24202=CARTESIAN_POINT('Ctrl Pts',(-3.92822141577198,-0.225058967539185,
57.4993371518887));
#24203=CARTESIAN_POINT('Ctrl Pts',(-3.91836055661331,-0.339027356384526,
57.5051196543202));
#24204=CARTESIAN_POINT('Ctrl Pts',(-3.90825529794007,-0.455820430022834,
57.5110454749722));
#24205=CARTESIAN_POINT('Ctrl Pts',(-3.89291276328519,-0.572284765183148,
57.5169712956243));
#24206=CARTESIAN_POINT('Ctrl Pts',(-3.87237285095124,-0.687908063054844,
57.5228971162763));
#24207=CARTESIAN_POINT('Ctrl Pts',(-3.85235870955178,-0.800571690584067,
57.5286712505817));
#24208=CARTESIAN_POINT('Ctrl Pts',(-3.82741013327092,-0.912436371183917,
57.5344453848871));
#24209=CARTESIAN_POINT('Ctrl Pts',(-3.79761646195819,-1.02303382537638,
57.5402195191925));
#24210=CARTESIAN_POINT('Ctrl Pts',(-3.76783009514474,-1.1336041644471,57.5459922378563));
#24211=CARTESIAN_POINT('Ctrl Pts',(-3.73320110443993,-1.24290748371754,
57.5517649565202));
#24212=CARTESIAN_POINT('Ctrl Pts',(-3.69386947882092,-1.35048779092421,
57.557537675184));
#24213=CARTESIAN_POINT('Ctrl Pts',(-3.65453736283475,-1.45806943938867,
57.5633104658192));
#24214=CARTESIAN_POINT('Ctrl Pts',(-3.61050264242728,-1.56392763358175,
57.5690832564544));
#24215=CARTESIAN_POINT('Ctrl Pts',(-3.56195420950007,-1.66762442097279,
57.5748560470896));
#24216=CARTESIAN_POINT('Ctrl Pts',(-3.51115626516457,-1.77612604123223,
57.5808963223296));
#24217=CARTESIAN_POINT('Ctrl Pts',(-3.45541646261234,-1.88226066750435,
57.5869365975695));
#24218=CARTESIAN_POINT('Ctrl Pts',(-3.39500539199336,-1.98555468026849,
57.5929768728094));
#24219=CARTESIAN_POINT('Ctrl Pts',(-3.33719109215317,-2.084408598341,57.5987575067274));
#24220=CARTESIAN_POINT('Ctrl Pts',(-3.27509907872395,-2.18066071817606,
57.6045381406453));
#24221=CARTESIAN_POINT('Ctrl Pts',(-3.20901054362121,-2.27392619293767,
57.6103187745633));
#24222=CARTESIAN_POINT('Ctrl Pts',(-3.14287855809915,-2.36725298580807,
57.6161032090037));
#24223=CARTESIAN_POINT('Ctrl Pts',(-3.07274508360941,-2.45758889200227,
57.6218876434442));
#24224=CARTESIAN_POINT('Ctrl Pts',(-2.99893087505149,-2.54458299268524,
57.6276720778847));
#24225=CARTESIAN_POINT('Ctrl Pts',(-2.92501327916339,-2.63169894101769,
57.6334646142509));
#24226=CARTESIAN_POINT('Ctrl Pts',(-2.84740495560434,-2.71546343896211,
57.6392571506171));
#24227=CARTESIAN_POINT('Ctrl Pts',(-2.7664625042894,-2.79556330859469,57.6450496869833));
#24228=CARTESIAN_POINT('Ctrl Pts',(-2.75579757715864,-2.80611721768611,
57.6458129079785));
#24229=CARTESIAN_POINT('Ctrl Pts',(-2.74507481257095,-2.81660756592347,
57.6465761289737));
#24230=CARTESIAN_POINT('Ctrl Pts',(-2.73429506597381,-2.82703369137888,
57.6473393499689));
#24231=CARTESIAN_POINT('Ctrl Pts',(-2.65128173977405,-2.90732383044949,
57.653216808485));
#24232=CARTESIAN_POINT('Ctrl Pts',(-2.56459287448662,-2.98408606550775,
57.659094267001));
#24233=CARTESIAN_POINT('Ctrl Pts',(-2.47456054136355,-3.05696567320056,
57.6649717255171));
#24234=CARTESIAN_POINT('Ctrl Pts',(-2.38464327049678,-3.12975213999823,
57.6708416725801));
#24235=CARTESIAN_POINT('Ctrl Pts',(-2.29139134749635,-3.1986655904819,57.6767116196432));
#24236=CARTESIAN_POINT('Ctrl Pts',(-2.19517356620747,-3.26338811884581,
57.6825815667062));
#24237=CARTESIAN_POINT('Ctrl Pts',(-2.09905315097321,-3.32804515227577,
57.6884455737697));
#24238=CARTESIAN_POINT('Ctrl Pts',(-1.99997318774395,-3.38851947061545,
57.6943095808331));
#24239=CARTESIAN_POINT('Ctrl Pts',(-1.89833490173518,-3.44453387279819,
57.7001735878965));
#24240=CARTESIAN_POINT('Ctrl Pts',(-1.79385103043734,-3.50211652022676,
57.7062017706155));
#24241=CARTESIAN_POINT('Ctrl Pts',(-1.68666381001068,-3.55498554751881,
57.7122299533345));
#24242=CARTESIAN_POINT('Ctrl Pts',(-1.57724068230134,-3.60288784589441,
57.7182581360534));
#24243=CARTESIAN_POINT('Ctrl Pts',(-1.4709174798734,-3.64943308613357,57.7241155421148));
#24244=CARTESIAN_POINT('Ctrl Pts',(-1.36248375739337,-3.69128905536023,
57.7299729481762));
#24245=CARTESIAN_POINT('Ctrl Pts',(-1.25239186243257,-3.72827086233185,
57.7358303542376));
#24246=CARTESIAN_POINT('Ctrl Pts',(-1.14231587017115,-3.7652473273066,57.7416869142007));
#24247=CARTESIAN_POINT('Ctrl Pts',(-1.03058257265253,-3.79735089876927,
57.7475434741638));
#24248=CARTESIAN_POINT('Ctrl Pts',(-0.917661582905724,-3.8244458708758,
57.7534000341269));
#24249=CARTESIAN_POINT('Ctrl Pts',(-0.804729700281146,-3.8515434566879,
57.7592571590406));
#24250=CARTESIAN_POINT('Ctrl Pts',(-0.690610298803393,-3.87363138643092,
57.7651142839544));
#24251=CARTESIAN_POINT('Ctrl Pts',(-0.57578465712533,-3.89062476070606,
57.7709714088682));
#24252=CARTESIAN_POINT('Ctrl Pts',(-0.455089013286741,-3.90848685334629,
57.7771279558918));
#24253=CARTESIAN_POINT('Ctrl Pts',(-0.333613513951472,-3.92071965581202,
57.7832845029155));
#24254=CARTESIAN_POINT('Ctrl Pts',(-0.211923433336705,-3.92728627151151,
57.7894410499391));
#24255=CARTESIAN_POINT('Ctrl Pts',(-0.0959792332007362,-3.93354282916215,
57.7953069012612));
#24256=CARTESIAN_POINT('Ctrl Pts',(0.0201593256405265,-3.93465611332302,
57.8011727525832));
#24257=CARTESIAN_POINT('Ctrl Pts',(0.136004315335366,-3.93064776165585,
57.8070386039053));
#24258=CARTESIAN_POINT('Ctrl Pts',(0.251928956505384,-3.92663665396856,
57.8129084884075));
#24259=CARTESIAN_POINT('Ctrl Pts',(0.367559216520916,-3.91749693078149,
57.8187783729097));
#24260=CARTESIAN_POINT('Ctrl Pts',(0.482413400481056,-3.90330197538396,
57.8246482574119));
#24261=CARTESIAN_POINT('Ctrl Pts',(0.597430446905614,-3.88908689163464,
57.830526465371));
#24262=CARTESIAN_POINT('Ctrl Pts',(0.711668816482015,-3.86980234051534,
57.8364046733302));
#24263=CARTESIAN_POINT('Ctrl Pts',(0.82465808600255,-3.84557252450017,57.8422828812893));
#24264=CARTESIAN_POINT('Ctrl Pts',(0.841106059963436,-3.84204536316365,
57.8431385785768));
#24265=CARTESIAN_POINT('Ctrl Pts',(0.857527593346193,-3.83841349227568,
57.8439942758644));
#24266=CARTESIAN_POINT('Ctrl Pts',(0.873921266230486,-3.8346773815316,57.8448499731519));
#24267=CARTESIAN_POINT('Ctrl Pts',(0.986522809923481,-3.80901553990768,
57.8507274135638));
#24268=CARTESIAN_POINT('Ctrl Pts',(1.09817767466564,-3.77834778367696,57.8566048539757));
#24269=CARTESIAN_POINT('Ctrl Pts',(1.20840733454266,-3.7427584364775,57.8624822943876));
#24270=CARTESIAN_POINT('Ctrl Pts',(1.31849611878142,-3.7072145731524,57.8683522233169));
#24271=CARTESIAN_POINT('Ctrl Pts',(1.42716293148851,-3.66676175352668,57.8742221522463));
#24272=CARTESIAN_POINT('Ctrl Pts',(1.53394001998351,-3.62153517380309,57.8800920811756));
#24273=CARTESIAN_POINT('Ctrl Pts',(1.64060905662699,-3.57635436059875,57.8859560700976));
#24274=CARTESIAN_POINT('Ctrl Pts',(1.74539179526742,-3.52640955642787,57.8918200590196));
#24275=CARTESIAN_POINT('Ctrl Pts',(1.84783685675272,-3.47188535968949,57.8976840479416));
#24276=CARTESIAN_POINT('Ctrl Pts',(1.95315053552432,-3.41583440264642,57.903712237458));
#24277=CARTESIAN_POINT('Ctrl Pts',(2.05599326083579,-3.3549439344886,57.9097404269743));
#24278=CARTESIAN_POINT('Ctrl Pts',(2.15589764895159,-3.28946717984006,57.9157686164907));
#24279=CARTESIAN_POINT('Ctrl Pts',(2.25297136636655,-3.22584563029778,57.9216260045061));
#24280=CARTESIAN_POINT('Ctrl Pts',(2.3472706518138,-3.15789443962736,57.9274833925216));
#24281=CARTESIAN_POINT('Ctrl Pts',(2.43839351015087,-3.08589145785364,57.933340780537));
#24282=CARTESIAN_POINT('Ctrl Pts',(2.52950320684809,-3.01389887607539,57.9391973225206));
#24283=CARTESIAN_POINT('Ctrl Pts',(2.61743706519509,-2.93785592262794,57.9450538645043));
#24284=CARTESIAN_POINT('Ctrl Pts',(2.70182485264192,-2.85808178078347,57.9509104064879));
#24285=CARTESIAN_POINT('Ctrl Pts',(2.78622078178691,-2.77829994236343,57.9567675135083));
#24286=CARTESIAN_POINT('Ctrl Pts',(2.86706966014709,-2.69478648331711,57.9626246205287));
#24287=CARTESIAN_POINT('Ctrl Pts',(2.94403743498049,-2.60789811561599,57.968481727549));
#24288=CARTESIAN_POINT('Ctrl Pts',(3.02494046039717,-2.51656727182126,57.9746382999478));
#24289=CARTESIAN_POINT('Ctrl Pts',(3.10155467196922,-2.42150765840215,57.9807948723466));
#24290=CARTESIAN_POINT('Ctrl Pts',(3.17354032432473,-2.32317257427958,57.9869514447454));
#24291=CARTESIAN_POINT('Ctrl Pts',(3.24212651904858,-2.22948127598435,57.9928172785548));
#24292=CARTESIAN_POINT('Ctrl Pts',(3.30651113921793,-2.13281718287333,57.9986831123642));
#24293=CARTESIAN_POINT('Ctrl Pts',(3.36644573060327,-2.03360078257827,58.0045489461735));
#24294=CARTESIAN_POINT('Ctrl Pts',(3.42642153266298,-1.93431616166687,58.0104188132959));
#24295=CARTESIAN_POINT('Ctrl Pts',(3.48194101623978,-1.83247610023236,58.0162886804183));
#24296=CARTESIAN_POINT('Ctrl Pts',(3.53280247247931,-1.72852413649448,58.0221585475406));
#24297=CARTESIAN_POINT('Ctrl Pts',(3.58373605267083,-1.62442476395245,58.0280367384124));
#24298=CARTESIAN_POINT('Ctrl Pts',(3.62999826139828,-1.51820788985982,58.0339149292841));
#24299=CARTESIAN_POINT('Ctrl Pts',(3.67143611213218,-1.41033537661496,58.0397931201558));
#24300=CARTESIAN_POINT('Ctrl Pts',(3.6774691868759,-1.3946298580209,58.0406489455488));
#24301=CARTESIAN_POINT('Ctrl Pts',(3.68340008502672,-1.37888926644417,58.0415047709417));
#24302=CARTESIAN_POINT('Ctrl Pts',(3.68922842404239,-1.36311504842313,58.0423605963347));
#24303=CARTESIAN_POINT('Ctrl Pts',(3.72925510536922,-1.25478408205178,58.0482380599109));
#24304=CARTESIAN_POINT('Ctrl Pts',(3.76457179281869,-1.14451102670765,58.0541155234872));
#24305=CARTESIAN_POINT('Ctrl Pts',(3.79498766993197,-1.03274274873477,58.0599929870635));
#24306=CARTESIAN_POINT('Ctrl Pts',(3.82536467469992,-0.921117313760708,
58.0658629390762));
#24307=CARTESIAN_POINT('Ctrl Pts',(3.85085321809989,-0.808000851035608,
58.0717328910889));
#24308=CARTESIAN_POINT('Ctrl Pts',(3.87131097836753,-0.69385899775889,58.0776028431016));
#24309=CARTESIAN_POINT('Ctrl Pts',(3.89174803634702,-0.579832650652215,
58.0834668549999));
#24310=CARTESIAN_POINT('Ctrl Pts',(3.90716436552608,-0.464783380736541,
58.0893308668981));
#24311=CARTESIAN_POINT('Ctrl Pts',(3.91746796700674,-0.349190102202228,
58.0951948787963));
#24312=CARTESIAN_POINT('Ctrl Pts',(3.92806002826915,-0.230360672506577,
58.1012230596597));
#24313=CARTESIAN_POINT('Ctrl Pts',(3.93324873810663,-0.110956751342765,
58.1072512405231));
#24314=CARTESIAN_POINT('Ctrl Pts',(3.93299083247968,0.00849185673065156,
58.1132794213865));
#24315=CARTESIAN_POINT('Ctrl Pts',(3.93274023297324,0.124556645937995,58.1191368319708));
#24316=CARTESIAN_POINT('Ctrl Pts',(3.92734746710776,0.240663184613262,58.1249942425552));
#24317=CARTESIAN_POINT('Ctrl Pts',(3.91682562021546,0.356322972629773,58.1308516531395));
#24318=CARTESIAN_POINT('Ctrl Pts',(3.90630529341633,0.471966051255202,58.1367082175026));
#24319=CARTESIAN_POINT('Ctrl Pts',(3.89065739645109,0.587162096868206,58.1425647818658));
#24320=CARTESIAN_POINT('Ctrl Pts',(3.86994698709251,0.701426629871944,58.1484213462289));
#24321=CARTESIAN_POINT('Ctrl Pts',(3.84923458036361,0.81570218286964,58.1542784754156));
#24322=CARTESIAN_POINT('Ctrl Pts',(3.82345876422852,0.929045638766885,58.1601356046023));
#24323=CARTESIAN_POINT('Ctrl Pts',(3.79273579573425,1.04098231673549,58.1659927337891));
#24324=CARTESIAN_POINT('Ctrl Pts',(3.76044229612203,1.15864109919484,58.1721492742664));
#24325=CARTESIAN_POINT('Ctrl Pts',(3.72268260755957,1.27474498151757,58.1783058147438));
#24326=CARTESIAN_POINT('Ctrl Pts',(3.67965076860994,1.3887617582106,58.1844623552212));
#24327=CARTESIAN_POINT('Ctrl Pts',(3.63865070715375,1.49739515537782,58.1903282104598));
#24328=CARTESIAN_POINT('Ctrl Pts',(3.59286519680946,1.60413366828352,58.1961940656984));
#24329=CARTESIAN_POINT('Ctrl Pts',(3.54251067677579,1.7085394654293,58.202059920937));
#24330=CARTESIAN_POINT('Ctrl Pts',(3.49212153558816,1.81301704658127,58.2079298092332));
#24331=CARTESIAN_POINT('Ctrl Pts',(3.43715732435433,1.91515835608604,58.2137996975294));
#24332=CARTESIAN_POINT('Ctrl Pts',(3.3778793279353,2.01455212042461,58.2196695858256));
#24333=CARTESIAN_POINT('Ctrl Pts',(3.31851727774101,2.11408682105717,58.2255477973833));
#24334=CARTESIAN_POINT('Ctrl Pts',(3.25482946277169,2.21086585963588,58.2314260089411));
#24335=CARTESIAN_POINT('Ctrl Pts',(3.18711913504503,2.30450875872272,58.2373042204989));
#24336=CARTESIAN_POINT('Ctrl Pts',(3.1772628296522,2.31813995860402,58.2381598868385));
#24337=CARTESIAN_POINT('Ctrl Pts',(3.16732135603069,2.3317047665503,58.239015553178));
#24338=CARTESIAN_POINT('Ctrl Pts',(3.15729571616681,2.34520207246084,58.2398712195176));
#24339=CARTESIAN_POINT('Ctrl Pts',(3.08843061494,2.43791369490481,58.2457487046349));
#24340=CARTESIAN_POINT('Ctrl Pts',(3.01536557255422,2.52774145148418,58.2516261897521));
#24341=CARTESIAN_POINT('Ctrl Pts',(2.93837061745917,2.61428137629684,58.2575036748694));
#24342=CARTESIAN_POINT('Ctrl Pts',(2.86147405986521,2.70071070539146,58.2633736487173));
#24343=CARTESIAN_POINT('Ctrl Pts',(2.78065784949517,2.78386025355741,58.2692436225652));
#24344=CARTESIAN_POINT('Ctrl Pts',(2.69623423127772,2.8633564168797,58.2751135964131));
#24345=CARTESIAN_POINT('Ctrl Pts',(2.61189604166093,2.94277213771287,58.2809776304107));
#24346=CARTESIAN_POINT('Ctrl Pts',(2.52395800393851,3.01854154625617,58.2868416644083));
#24347=CARTESIAN_POINT('Ctrl Pts',(2.4327709769061,3.0903259332833,58.2927056984059));
#24348=CARTESIAN_POINT('Ctrl Pts',(2.33903155703685,3.16411961879518,58.2987338710849));
#24349=CARTESIAN_POINT('Ctrl Pts',(2.24185886899489,3.23370156412764,58.3047620437638));
#24350=CARTESIAN_POINT('Ctrl Pts',(2.14167301494458,3.29874607950629,58.3107902164427));
#24351=CARTESIAN_POINT('Ctrl Pts',(2.04432478387846,3.36194830074489,58.3166476496344));
#24352=CARTESIAN_POINT('Ctrl Pts',(1.94413215200164,3.42086643555492,58.3225050828262));
#24353=CARTESIAN_POINT('Ctrl Pts',(1.84151141899156,3.4752445516429,58.3283625160179));
#24354=CARTESIAN_POINT('Ctrl Pts',(1.73890550896687,3.52961481311908,58.3342191031365));
#24355=CARTESIAN_POINT('Ctrl Pts',(1.63387255962941,3.57944616682173,58.340075690255));
#24356=CARTESIAN_POINT('Ctrl Pts',(1.52685389817576,3.62452840706559,58.3459322773736));
#24357=CARTESIAN_POINT('Ctrl Pts',(1.41982491334592,3.66961499609237,58.3517894294381));
#24358=CARTESIAN_POINT('Ctrl Pts',(1.31081021577677,3.70995140082501,58.3576465815025));
#24359=CARTESIAN_POINT('Ctrl Pts',(1.20027089819499,3.74537565151296,58.363503733567));
#24360=CARTESIAN_POINT('Ctrl Pts',(1.08408195406364,3.78261042348478,58.3696602426614));
#24361=CARTESIAN_POINT('Ctrl Pts',(0.966208905409569,3.8144174858749,58.3758167517559));
#24362=CARTESIAN_POINT('Ctrl Pts',(0.847203506495735,3.840668590048,58.3819732608503));
#24363=CARTESIAN_POINT('Ctrl Pts',(0.733816006300927,3.86568045595248,58.3878391390585));
#24364=CARTESIAN_POINT('Ctrl Pts',(0.619401048536494,3.88564892764175,58.3937050172667));
#24365=CARTESIAN_POINT('Ctrl Pts',(0.504443596768991,3.9005160758134,58.3995708954749));
#24366=CARTESIAN_POINT('Ctrl Pts',(0.389407105984118,3.91539344589554,58.4054408067688));
#24367=CARTESIAN_POINT('Ctrl Pts',(0.273827788375325,3.92516247373269,58.4113107180626));
#24368=CARTESIAN_POINT('Ctrl Pts',(0.158192865142057,3.92981730076834,58.4171806293565));
#24369=CARTESIAN_POINT('Ctrl Pts',(0.0423939789340578,3.93447872805299,
58.4230588638116));
#24370=CARTESIAN_POINT('Ctrl Pts',(-0.0734602595775473,3.93401148640706,
58.4289370982668));
#24371=CARTESIAN_POINT('Ctrl Pts',(-0.188885493857291,3.92846169259804,
58.4348153327219));
#24372=CARTESIAN_POINT('Ctrl Pts',(-0.205684189554592,3.92765398969008,
58.4356708360481));
#24373=CARTESIAN_POINT('Ctrl Pts',(-0.222473813232077,3.92673872131916,
58.4365263393742));
#24374=CARTESIAN_POINT('Ctrl Pts',(-0.239252888532522,3.92571612006381,
58.4373818427004));
#24375=CARTESIAN_POINT('Ctrl Pts',(-0.3545258843286,3.91869080382328,58.4432591887134));
#24376=CARTESIAN_POINT('Ctrl Pts',(-0.469678179270346,3.90657243372861,
58.4491365347265));
#24377=CARTESIAN_POINT('Ctrl Pts',(-0.58422391822207,3.88936645398415,58.4550138807396));
#24378=CARTESIAN_POINT('Ctrl Pts',(-0.69862326109188,3.87218246447734,58.4608837151644));
#24379=CARTESIAN_POINT('Ctrl Pts',(-0.81241718536282,3.84992385745057,58.4667535495892));
#24380=CARTESIAN_POINT('Ctrl Pts',(-0.925122199257555,3.82264802413731,
58.472623384014));
#24381=CARTESIAN_POINT('Ctrl Pts',(-1.03771316091207,3.79539979270071,58.478487278439));
#24382=CARTESIAN_POINT('Ctrl Pts',(-1.14921700547454,3.76314453084539,58.484351172864));
#24383=CARTESIAN_POINT('Ctrl Pts',(-1.25915836950832,3.72599103601944,58.4902150672889));
#24384=CARTESIAN_POINT('Ctrl Pts',(-1.37218074418515,3.68779634697153,58.4962432922304));
#24385=CARTESIAN_POINT('Ctrl Pts',(-1.48355132852975,3.64442488787103,58.5022715171718));
#24386=CARTESIAN_POINT('Ctrl Pts',(-1.59276778428541,3.59605058158844,58.5082997421132));
#24387=CARTESIAN_POINT('Ctrl Pts',(-1.69888739854487,3.54904793269951,58.5141570362456));
#24388=CARTESIAN_POINT('Ctrl Pts',(-1.8029730017585,3.49732251472514,58.5200143303779));
#24389=CARTESIAN_POINT('Ctrl Pts',(-1.90458280629988,3.44108316289318,58.5258716245103));
#24390=CARTESIAN_POINT('Ctrl Pts',(-2.00617794100624,3.38485193057307,58.5317280730005));
#24391=CARTESIAN_POINT('Ctrl Pts',(-2.10529762699227,3.32410826002245,58.5375845214906));
#24392=CARTESIAN_POINT('Ctrl Pts',(-2.20152470130567,3.25910693128363,58.5434409699808));
#24393=CARTESIAN_POINT('Ctrl Pts',(-2.29776106777071,3.19409932570217,58.5492979839979));
#24394=CARTESIAN_POINT('Ctrl Pts',(-2.39110392544248,3.12483347554203,58.555154998015));
#24395=CARTESIAN_POINT('Ctrl Pts',(-2.48116571288909,3.05160706926427,58.5610120120322));
#24396=CARTESIAN_POINT('Ctrl Pts',(-2.57583576307342,2.97463382951768,58.5671687165198));
#24397=CARTESIAN_POINT('Ctrl Pts',(-2.66687968578266,2.89328431438268,58.5733254210074));
#24398=CARTESIAN_POINT('Ctrl Pts',(-2.75388856641615,2.80795063413915,58.579482125495));
#24399=CARTESIAN_POINT('Ctrl Pts',(-2.83678546754567,2.72664976458811,58.5853478683878));
#24400=CARTESIAN_POINT('Ctrl Pts',(-2.91601974679324,2.64173304362052,58.5912136112807));
#24401=CARTESIAN_POINT('Ctrl Pts',(-2.9912779436942,2.5535749966603,58.5970793541736));
#24402=CARTESIAN_POINT('Ctrl Pts',(-3.06658789782654,2.46535632086997,58.6029491311069));
#24403=CARTESIAN_POINT('Ctrl Pts',(-3.13791607168383,2.37389220472495,58.6088189080402));
#24404=CARTESIAN_POINT('Ctrl Pts',(-3.20499138435813,2.27958751229038,58.6146886849736));
#24405=CARTESIAN_POINT('Ctrl Pts',(-3.27216183241156,2.18514906404743,58.6205667872271));
#24406=CARTESIAN_POINT('Ctrl Pts',(-3.33506716014055,2.08786234517067,58.6264448894806));
#24407=CARTESIAN_POINT('Ctrl Pts',(-3.39348138473765,1.9881582158971,58.6323229917341));
#24408=CARTESIAN_POINT('Ctrl Pts',(-3.40199285287121,1.97363044419508,58.6331794831172));
#24409=CARTESIAN_POINT('Ctrl Pts',(-3.41040905280243,1.95905138454428,58.6340359745003));
#24410=CARTESIAN_POINT('Ctrl Pts',(-3.41872937063379,1.94442240533429,58.6348924658833));
#24411=CARTESIAN_POINT('Ctrl Pts',(-3.47820543226259,1.83985018986187,58.6410149164095));
#24412=CARTESIAN_POINT('Ctrl Pts',(-3.53295935359999,1.73240702198956,58.6471373669357));
#24413=CARTESIAN_POINT('Ctrl Pts',(-3.58271656562753,1.62253844650233,58.6532598174618));
#24414=CARTESIAN_POINT('Ctrl Pts',(-3.63239088497217,1.51285290580777,58.6593720683339));
#24415=CARTESIAN_POINT('Ctrl Pts',(-3.67708492333178,1.40075033324975,58.665484319206));
#24416=CARTESIAN_POINT('Ctrl Pts',(-3.71656924016522,1.28670201797378,58.6715965700781));
#24417=CARTESIAN_POINT('Ctrl Pts',(-3.75597208802662,1.17288902142062,58.6776962093911));
#24418=CARTESIAN_POINT('Ctrl Pts',(-3.79018652288456,1.0571386266198,58.6837958487041));
#24419=CARTESIAN_POINT('Ctrl Pts',(-3.81903093378893,0.939942406088445,
58.6898954880171));
#24420=CARTESIAN_POINT('Ctrl Pts',(-3.84783991649881,0.822890132005107,
58.6959876354382));
#24421=CARTESIAN_POINT('Ctrl Pts',(-3.87129192094621,0.704395919129239,
58.7020797828594));
#24422=CARTESIAN_POINT('Ctrl Pts',(-3.88925465038843,0.584967746488714,
58.7081719302805));
#24423=CARTESIAN_POINT('Ctrl Pts',(-3.90719108832866,0.465714377240255,
58.7142551608103));
#24424=CARTESIAN_POINT('Ctrl Pts',(-3.91965421122248,0.34553013120326,58.7203383913401));
#24425=CARTESIAN_POINT('Ctrl Pts',(-3.9265625930753,0.224933773946519,58.7264216218699));
#24426=CARTESIAN_POINT('Ctrl Pts',(-3.93085931016457,0.149928014252427,
58.7302051302416));
#24427=CARTESIAN_POINT('Ctrl Pts',(-3.93300828556888,0.0747630755042776,
58.7339886386134));
#24428=CARTESIAN_POINT('Ctrl Pts',(-3.93299997598718,-0.000434608922615996,
58.7377721469851));
#24429=CARTESIAN_POINT('Ctrl Pts',(-3.93299997598709,-0.000434609756364034,
58.737772147027));
#24430=CARTESIAN_POINT('Ctrl Pts',(-3.93298638829109,-0.123396433039988,
58.7439588679526));
#24431=CARTESIAN_POINT('Ctrl Pts',(-3.92720208159448,-0.24622899957672,
58.7501455888783));
#24432=CARTESIAN_POINT('Ctrl Pts',(-3.91570891145027,-0.368392074818398,
58.7563323098039));
#24433=CARTESIAN_POINT('Ctrl Pts',(-3.90393241978397,-0.493566628006301,
58.762671541409));
#24434=CARTESIAN_POINT('Ctrl Pts',(-3.8861620251258,-0.618037871898027,
58.7690107730142));
#24435=CARTESIAN_POINT('Ctrl Pts',(-3.8625194007969,-0.741237396835596,
58.7753500046194));
#24436=CARTESIAN_POINT('Ctrl Pts',(-3.83934346399611,-0.862005056301857,
58.7815641045858));
#24437=CARTESIAN_POINT('Ctrl Pts',(-3.81052514587804,-0.981550438922573,
58.7877782045522));
#24438=CARTESIAN_POINT('Ctrl Pts',(-3.77622924634803,-1.09935511961599,
58.7939923045186));
#24439=CARTESIAN_POINT('Ctrl Pts',(-3.74089743603393,-1.22071810147133,
58.8003941019432));
#24440=CARTESIAN_POINT('Ctrl Pts',(-3.69975207331446,-1.34023319123688,
58.8067958993678));
#24441=CARTESIAN_POINT('Ctrl Pts',(-3.65302592841248,-1.45735739142676,
58.8131976967924));
#24442=CARTESIAN_POINT('Ctrl Pts',(-3.6062997835105,-1.57448159161665,58.819599494217));
#24443=CARTESIAN_POINT('Ctrl Pts',(-3.55399308169572,-1.68921458270921,
58.8260012916416));
#24444=CARTESIAN_POINT('Ctrl Pts',(-3.49638884021169,-1.80104249756723,
58.8324030890661));
#24445=CARTESIAN_POINT('Ctrl Pts',(-3.44350101193356,-1.90371437389691,
58.838280731999));
#24446=CARTESIAN_POINT('Ctrl Pts',(-3.38600025284171,-2.00422289819233,
58.8441583749319));
#24447=CARTESIAN_POINT('Ctrl Pts',(-3.32408739703009,-2.10212558542675,
58.8500360178648));
#24448=CARTESIAN_POINT('Ctrl Pts',(-3.26225364615663,-2.19990318416516,
58.8559061510395));
#24449=CARTESIAN_POINT('Ctrl Pts',(-3.19601922821315,-2.29508122176198,
58.8617762842141));
#24450=CARTESIAN_POINT('Ctrl Pts',(-3.12563156484665,-2.38724031484774,
58.8676464173887));
#24451=CARTESIAN_POINT('Ctrl Pts',(-3.05531510950412,-2.47930617473615,
58.8735106120144));
#24452=CARTESIAN_POINT('Ctrl Pts',(-2.98085401545927,-2.56835883939158,
58.8793748066401));
#24453=CARTESIAN_POINT('Ctrl Pts',(-2.90253947355337,-2.65400708447897,
58.8852390012658));
#24454=CARTESIAN_POINT('Ctrl Pts',(-2.82203585200479,-2.74204940383647,
58.8912671142234));
#24455=CARTESIAN_POINT('Ctrl Pts',(-2.73746041099675,-2.82649379389863,
58.8972952271811));
#24456=CARTESIAN_POINT('Ctrl Pts',(-2.64917473959605,-2.90695067021893,
58.9033233401387));
#24457=CARTESIAN_POINT('Ctrl Pts',(-2.5633864010418,-2.98513166646979,58.9091809361341));
#24458=CARTESIAN_POINT('Ctrl Pts',(-2.47409524585201,-3.05954741859253,
58.9150385321296));
#24459=CARTESIAN_POINT('Ctrl Pts',(-2.38167048197705,-3.12987774765713,
58.9208961281251));
#24460=CARTESIAN_POINT('Ctrl Pts',(-2.28925905977581,-3.20019792441769,
58.9267528785664));
#24461=CARTESIAN_POINT('Ctrl Pts',(-2.19371525654455,-3.26643360112181,
58.9326096290078));
#24462=CARTESIAN_POINT('Ctrl Pts',(-2.09544040396874,-3.32830565204209,
58.9384663794492));
#24463=CARTESIAN_POINT('Ctrl Pts',(-1.99715606608524,-3.39018367473873,
58.9443236951734));
#24464=CARTESIAN_POINT('Ctrl Pts',(-1.89614050391788,-3.44769701463841,
58.9501810108975));
#24465=CARTESIAN_POINT('Ctrl Pts',(-1.79282238876367,-3.50061092987321,
58.9560383266217));
#24466=CARTESIAN_POINT('Ctrl Pts',(-1.68423075796155,-3.55622565279857,
58.9621946087573));
#24467=CARTESIAN_POINT('Ctrl Pts',(-1.57309576447285,-3.60675879098142,
58.9683508908929));
#24468=CARTESIAN_POINT('Ctrl Pts',(-1.45994091604914,-3.65199418422944,
58.9745071730285));
#24469=CARTESIAN_POINT('Ctrl Pts',(-1.35212080864639,-3.69509693259904,
58.9803732142129));
#24470=CARTESIAN_POINT('Ctrl Pts',(-1.24246737256233,-3.73338998665922,
58.9862392553973));
#24471=CARTESIAN_POINT('Ctrl Pts',(-1.13144973577546,-3.76673738073331,
58.9921052965816));
#24472=CARTESIAN_POINT('Ctrl Pts',(-1.0203557757963,-3.80010770071039,58.9979753705936));
#24473=CARTESIAN_POINT('Ctrl Pts',(-0.907896146386374,-3.82852548957049,
59.0038454446055));
#24474=CARTESIAN_POINT('Ctrl Pts',(-0.794550664326466,-3.85190579347657,
59.0097155186175));
#24475=CARTESIAN_POINT('Ctrl Pts',(-0.681044496122018,-3.87531924286693,
59.0155939144394));
#24476=CARTESIAN_POINT('Ctrl Pts',(-0.566650374805284,-3.89368089219465,
59.0214723102613));
#24477=CARTESIAN_POINT('Ctrl Pts',(-0.451853736377204,-3.90695753763999,
59.0273507060832));
#24478=CARTESIAN_POINT('Ctrl Pts',(-0.435169791696756,-3.90888709604157,
59.0282050414718));
#24479=CARTESIAN_POINT('Ctrl Pts',(-0.418477344820747,-3.91070933780461,
59.0290593768604));
#24480=CARTESIAN_POINT('Ctrl Pts',(-0.40177788411543,-3.91242425253649,
59.0299137122491));
#24481=CARTESIAN_POINT('Ctrl Pts',(-0.286909493420838,-3.92422041164043,
59.0357903170649));
#24482=CARTESIAN_POINT('Ctrl Pts',(-0.171332551631751,-3.93097286977808,
59.0416669218808));
#24483=CARTESIAN_POINT('Ctrl Pts',(-0.0555272300337676,-3.93260800572912,
59.0475435266966));
#24484=CARTESIAN_POINT('Ctrl Pts',(0.0601300414201887,-3.93424105125711,
59.0534126186264));
#24485=CARTESIAN_POINT('Ctrl Pts',(0.176014703109235,-3.93076977955394,
59.0592817105561));
#24486=CARTESIAN_POINT('Ctrl Pts',(0.291640467311843,-3.92217220909869,
59.0651508024859));
#24487=CARTESIAN_POINT('Ctrl Pts',(0.407149200849934,-3.9135833406779,59.0710139540119));
#24488=CARTESIAN_POINT('Ctrl Pts',(0.522399149025639,-3.89987852482489,
59.0768771055379));
#24489=CARTESIAN_POINT('Ctrl Pts',(0.636903685379811,-3.88108782373571,
59.0827402570638));
#24490=CARTESIAN_POINT('Ctrl Pts',(0.754637461873528,-3.8617671900505,59.0887687603292));
#24491=CARTESIAN_POINT('Ctrl Pts',(0.871582712350225,-3.83706952811667,
59.0947972635945));
#24492=CARTESIAN_POINT('Ctrl Pts',(0.987215344586107,-3.80708482482512,
59.1008257668599));
#24493=CARTESIAN_POINT('Ctrl Pts',(1.09954983810318,-3.77795536203952,59.1066823217776));
#24494=CARTESIAN_POINT('Ctrl Pts',(1.21064515363453,-3.74383649058138,59.1125388766954));
#24495=CARTESIAN_POINT('Ctrl Pts',(1.32003153369388,-3.70486244684654,59.1183954316132));
#24496=CARTESIAN_POINT('Ctrl Pts',(1.4294021684974,-3.66589401309979,59.1242511435289));
#24497=CARTESIAN_POINT('Ctrl Pts',(1.53706396837671,-3.62207193522498,59.1301068554445));
#24498=CARTESIAN_POINT('Ctrl Pts',(1.64256400733718,-3.57357978528539,59.1359625673601));
#24499=CARTESIAN_POINT('Ctrl Pts',(1.74807429704893,-3.5250829236796,59.1418188482371));
#24500=CARTESIAN_POINT('Ctrl Pts',(1.85142203335346,-3.471915260312,59.1476751291141));
#24501=CARTESIAN_POINT('Ctrl Pts',(1.95217652726788,-3.41430751491196,59.1535314099911));
#24502=CARTESIAN_POINT('Ctrl Pts',(2.0581175454533,-3.35373430407106,59.1596891537778));
#24503=CARTESIAN_POINT('Ctrl Pts',(2.1611907829416,-3.28825196343846,59.1658468975645));
#24504=CARTESIAN_POINT('Ctrl Pts',(2.26092875103528,-3.21818119172026,59.1720046413513));
#24505=CARTESIAN_POINT('Ctrl Pts',(2.35592550779208,-3.15144135147784,59.1778696664752));
#24506=CARTESIAN_POINT('Ctrl Pts',(2.44789649712951,-3.08053958472428,59.1837346915992));
#24507=CARTESIAN_POINT('Ctrl Pts',(2.53647167680405,-3.00579447613618,59.1895997167231));
#24508=CARTESIAN_POINT('Ctrl Pts',(2.62510786062882,-2.93099788854629,59.1954687812504));
#24509=CARTESIAN_POINT('Ctrl Pts',(2.71034327535287,-2.85235296739318,59.2013378457776));
#24510=CARTESIAN_POINT('Ctrl Pts',(2.79184477099934,-2.77021511342415,59.2072069103048));
#24511=CARTESIAN_POINT('Ctrl Pts',(2.8734620420719,-2.68796058006211,59.213084312022));
#24512=CARTESIAN_POINT('Ctrl Pts',(2.95133453412424,-2.60220351727131,59.2189617137391));
#24513=CARTESIAN_POINT('Ctrl Pts',(3.02516937696303,-2.51333229810247,59.2248391154563));
#24514=CARTESIAN_POINT('Ctrl Pts',(3.03599498323125,-2.50030207022755,59.2257008554482));
#24515=CARTESIAN_POINT('Ctrl Pts',(3.04673386801589,-2.48720494651646,59.2265625954401));
#24516=CARTESIAN_POINT('Ctrl Pts',(3.05738518806404,-2.47404220089443,59.227424335432));
#24517=CARTESIAN_POINT('Ctrl Pts',(3.13004555183358,-2.3842495854459,59.2333028876681));
#24518=CARTESIAN_POINT('Ctrl Pts',(3.19886580446545,-2.2911063406,59.2391814399041));
#24519=CARTESIAN_POINT('Ctrl Pts',(3.26352187689826,-2.19497470577826,59.2450599921402));
#24520=CARTESIAN_POINT('Ctrl Pts',(3.32809529196935,-2.09896596718288,59.2509310291407));
#24521=CARTESIAN_POINT('Ctrl Pts',(3.38851488609573,-1.99997677564306,59.2568020661411));
#24522=CARTESIAN_POINT('Ctrl Pts',(3.44449651071182,-1.89840269376494,59.2626731031416));
#24523=CARTESIAN_POINT('Ctrl Pts',(3.50042144825045,-1.79693146595523,59.2685381951212));
#24524=CARTESIAN_POINT('Ctrl Pts',(3.5519171575756,-1.69288091346448,59.2744032871007));
#24525=CARTESIAN_POINT('Ctrl Pts',(3.59874290193592,-1.58667530571499,59.2802683790802));
#24526=CARTESIAN_POINT('Ctrl Pts',(3.64686746882529,-1.47752383478829,59.2862961532275));
#24527=CARTESIAN_POINT('Ctrl Pts',(3.69005895967147,-1.36609637212501,59.2923239273748));
#24528=CARTESIAN_POINT('Ctrl Pts',(3.72810663232228,-1.25288065594236,59.2983517015221));
#24529=CARTESIAN_POINT('Ctrl Pts',(3.76508565851155,-1.14284483398345,59.3042101733424));
#24530=CARTESIAN_POINT('Ctrl Pts',(3.79720583164214,-1.03112029185799,59.3100686451628));
#24531=CARTESIAN_POINT('Ctrl Pts',(3.82432286679152,-0.918174063310112,
59.3159271169831));
#24532=CARTESIAN_POINT('Ctrl Pts',(3.85143594431274,-0.805244318834775,
59.3217847337818));
#24533=CARTESIAN_POINT('Ctrl Pts',(3.87354723963922,-0.691093643335088,
59.3276423505805));
#24534=CARTESIAN_POINT('Ctrl Pts',(3.89056298456905,-0.576201929102187,
59.3334999673792));
#24535=CARTESIAN_POINT('Ctrl Pts',(3.90758034144363,-0.46129933088524,59.3393581390848));
#24536=CARTESIAN_POINT('Ctrl Pts',(3.91950112792571,-0.345655962286249,
59.3452163107904));
#24537=CARTESIAN_POINT('Ctrl Pts',(3.92628321296247,-0.229758855344093,
59.351074482496));
#24538=CARTESIAN_POINT('Ctrl Pts',(3.93340898608571,-0.107988561218616,
59.3572295221725));
#24539=CARTESIAN_POINT('Ctrl Pts',(3.93486154728916,0.0140613566219913,
59.3633845618491));
#24540=CARTESIAN_POINT('Ctrl Pts',(3.9306539578738,0.135825120839118,59.3695396015257));
#24541=CARTESIAN_POINT('Ctrl Pts',(3.9266433659979,0.251887957617895,59.3754064648733));
#24542=CARTESIAN_POINT('Ctrl Pts',(3.91749072180953,0.367690413961021,59.3812733282208));
#24543=CARTESIAN_POINT('Ctrl Pts',(3.90326057992152,0.482748221364511,59.3871401915684));
#24544=CARTESIAN_POINT('Ctrl Pts',(3.88902068475051,0.597884888934454,59.3930110760409));
#24545=CARTESIAN_POINT('Ctrl Pts',(3.86969643059257,0.712275485802583,59.3988819605135));
#24546=CARTESIAN_POINT('Ctrl Pts',(3.84540336846444,0.825446505718101,59.404752844986));
#24547=CARTESIAN_POINT('Ctrl Pts',(3.82107596005679,0.938777530307518,59.4106320298958));
#24548=CARTESIAN_POINT('Ctrl Pts',(3.79176582972588,1.05088514016715,59.4165112148057));
#24549=CARTESIAN_POINT('Ctrl Pts',(3.75763815878209,1.16131152911896,59.4223903997155));
#24550=CARTESIAN_POINT('Ctrl Pts',(3.75271458121455,1.17724267462267,59.4232385860153));
#24551=CARTESIAN_POINT('Ctrl Pts',(3.74769081402651,1.19313886356976,59.424086772315));
#24552=CARTESIAN_POINT('Ctrl Pts',(3.74256743438735,1.20899875891715,59.4249349586148));
#24553=CARTESIAN_POINT('Ctrl Pts',(3.70705934153858,1.31891734317774,59.4308133982399));
#24554=CARTESIAN_POINT('Ctrl Pts',(3.66664671419419,1.42744985201521,59.436691837865));
#24555=CARTESIAN_POINT('Ctrl Pts',(3.62145598834394,1.53412695839938,59.44257027749));
#24556=CARTESIAN_POINT('Ctrl Pts',(3.5763229008701,1.6406680037866,59.4484412194769));
#24557=CARTESIAN_POINT('Ctrl Pts',(3.52642399432385,1.74535797677613,59.4543121614637));
#24558=CARTESIAN_POINT('Ctrl Pts',(3.47193542213628,1.84774279176386,59.4601831034505));
#24559=CARTESIAN_POINT('Ctrl Pts',(3.41750186398949,1.95002423457351,59.466048117878));
#24560=CARTESIAN_POINT('Ctrl Pts',(3.35848805055208,2.05000478708441,59.4719131323055));
#24561=CARTESIAN_POINT('Ctrl Pts',(3.29511789235706,2.14725105087139,59.477778146733));
#24562=CARTESIAN_POINT('Ctrl Pts',(3.22998876693747,2.24719658187791,59.4838059565274));
#24563=CARTESIAN_POINT('Ctrl Pts',(3.16025808282592,2.34425339745184,59.4898337663218));
#24564=CARTESIAN_POINT('Ctrl Pts',(3.08621931271244,2.43797853842906,59.4958615761161));
#24565=CARTESIAN_POINT('Ctrl Pts',(3.01426091902777,2.5290701460051,59.501720013656));
#24566=CARTESIAN_POINT('Ctrl Pts',(2.93823359066717,2.61701447246204,59.5075784511959));
#24567=CARTESIAN_POINT('Ctrl Pts',(2.85844974123687,2.70143555851751,59.5134368887357));
#24568=CARTESIAN_POINT('Ctrl Pts',(2.77867731787939,2.78584455438827,59.519294487272));
#24569=CARTESIAN_POINT('Ctrl Pts',(2.69514972639875,2.86673101362479,59.5251520858084));
#24570=CARTESIAN_POINT('Ctrl Pts',(2.60821774187903,2.9437542714954,59.5310096843447));
#24571=CARTESIAN_POINT('Ctrl Pts',(2.52127728521412,3.02078503583474,59.536867853746));
#24572=CARTESIAN_POINT('Ctrl Pts',(2.43093208457753,3.09395157690207,59.5427260231472));
#24573=CARTESIAN_POINT('Ctrl Pts',(2.33756709784436,3.16295258628318,59.5485841925485));
#24574=CARTESIAN_POINT('Ctrl Pts',(2.23946950746874,3.23545120691831,59.5547393083193));
#24575=CARTESIAN_POINT('Ctrl Pts',(2.13803836325414,3.30335061655387,59.5608944240901));
#24576=CARTESIAN_POINT('Ctrl Pts',(2.03375474315252,3.36635272137437,59.5670495398608));
#24577=CARTESIAN_POINT('Ctrl Pts',(1.93435423171398,3.42640473562894,59.572916440674));
#24578=CARTESIAN_POINT('Ctrl Pts',(1.83236272648546,3.48200754090552,59.5787833414872));
#24579=CARTESIAN_POINT('Ctrl Pts',(1.72822113911942,3.53295070646347,59.5846502423004));
#24580=CARTESIAN_POINT('Ctrl Pts',(1.62400793238906,3.58392890622078,59.5905211778486));
#24581=CARTESIAN_POINT('Ctrl Pts',(1.51764207618984,3.63024092116307,59.5963921133968));
#24582=CARTESIAN_POINT('Ctrl Pts',(1.40958331825366,3.67172491737888,59.602263048945));
#24583=CARTESIAN_POINT('Ctrl Pts',(1.30137143848424,3.71326769740521,59.6081423037486));
#24584=CARTESIAN_POINT('Ctrl Pts',(1.19146225961509,3.74996867734835,59.6140215585523));
#24585=CARTESIAN_POINT('Ctrl Pts',(1.08032948423019,3.78171617199161,59.6199008133559));
#24586=CARTESIAN_POINT('Ctrl Pts',(1.06429529911185,3.78629668574546,59.6207490695032));
#24587=CARTESIAN_POINT('Ctrl Pts',(1.04823565714201,3.79077417225764,59.6215973256504));
#24588=CARTESIAN_POINT('Ctrl Pts',(1.03215199383441,3.79514838466477,59.6224455817977));
#24589=CARTESIAN_POINT('Ctrl Pts',(0.920833718315192,3.82542319038558,59.6283165335643));
#24590=CARTESIAN_POINT('Ctrl Pts',(0.807997354646353,3.85084640293736,59.6341874853308));
#24591=CARTESIAN_POINT('Ctrl Pts',(0.69410380974655,3.871267092477,59.6400584370974));
#24592=CARTESIAN_POINT('Ctrl Pts',(0.580356270243658,3.89166160379131,59.6459218626197));
#24593=CARTESIAN_POINT('Ctrl Pts',(0.465554647974981,3.90706627292493,59.6517852881421));
#24594=CARTESIAN_POINT('Ctrl Pts',(0.350174337588973,3.91738011090245,59.6576487136643));
#24595=CARTESIAN_POINT('Ctrl Pts',(0.234911052071881,3.92768348803503,59.6635061921875));
#24596=CARTESIAN_POINT('Ctrl Pts',(0.119070655354441,3.93290626773586,59.6693636707107));
#24597=CARTESIAN_POINT('Ctrl Pts',(0.00313738484995835,3.93299874864159,
59.6752211492339));
#24598=CARTESIAN_POINT('Ctrl Pts',(-0.116222907459339,3.93309396331027,
59.6812517765567));
#24599=CARTESIAN_POINT('Ctrl Pts',(-0.235681210891267,3.92775076617025,
59.6872824038795));
#24600=CARTESIAN_POINT('Ctrl Pts',(-0.35470450151807,3.91697251925551,59.6933130312022));
#24601=CARTESIAN_POINT('Ctrl Pts',(-0.470180628499413,3.90651548851128,
59.6991639321716));
#24602=CARTESIAN_POINT('Ctrl Pts',(-0.585246863951679,3.89094281569465,
59.7050148331409));
#24603=CARTESIAN_POINT('Ctrl Pts',(-0.69941862137128,3.87031039996524,59.7108657341102));
#24604=CARTESIAN_POINT('Ctrl Pts',(-0.813574253703784,3.8496808982621,59.7167158087256));
#24605=CARTESIAN_POINT('Ctrl Pts',(-0.926835252369466,3.82399314808559,
59.7225658833409));
#24606=CARTESIAN_POINT('Ctrl Pts',(-1.03872561286469,3.79335446553297,59.7284159579562));
#24607=CARTESIAN_POINT('Ctrl Pts',(-1.15062728847733,3.76271268458751,59.7342666241711));
#24608=CARTESIAN_POINT('Ctrl Pts',(-1.26115765152597,3.7271190851998,59.7401172903859));
#24609=CARTESIAN_POINT('Ctrl Pts',(-1.36985498049327,3.68673111745592,59.7459679566008));
#24610=CARTESIAN_POINT('Ctrl Pts',(-1.47858964580015,3.64632927688837,59.7518206324552));
#24611=CARTESIAN_POINT('Ctrl Pts',(-1.58548963766565,3.60112993735095,59.7576733083097));
#24612=CARTESIAN_POINT('Ctrl Pts',(-1.69011303260906,3.55133875278113,59.7635259841642));
#24613=CARTESIAN_POINT('Ctrl Pts',(-1.79485550045048,3.50149090038243,59.7693853210057));
#24614=CARTESIAN_POINT('Ctrl Pts',(-1.89731582659599,3.44704095049977,59.7752446578472));
#24615=CARTESIAN_POINT('Ctrl Pts',(-1.9970764577922,3.38824063810884,59.7811039946887));
#24616=CARTESIAN_POINT('Ctrl Pts',(-2.09690534358347,3.32940009550421,59.7869673403927));
#24617=CARTESIAN_POINT('Ctrl Pts',(-2.1940305109698,3.26620348883162,59.7928306860968));
#24618=CARTESIAN_POINT('Ctrl Pts',(-2.28806461775223,3.19894503000448,59.7986940318009));
#24619=CARTESIAN_POINT('Ctrl Pts',(-2.38223514931497,3.13158899253506,59.8045658840531));
#24620=CARTESIAN_POINT('Ctrl Pts',(-2.4733053472488,3.0601595974302,59.8104377363053));
#24621=CARTESIAN_POINT('Ctrl Pts',(-2.56092203913391,2.98499033658038,59.8163095885574));
#24622=CARTESIAN_POINT('Ctrl Pts',(-2.57905967009159,2.969429462467,59.8175251273651));
#24623=CARTESIAN_POINT('Ctrl Pts',(-2.59704943683639,2.95370844251526,59.8187406661728));
#24624=CARTESIAN_POINT('Ctrl Pts',(-2.61488841530372,2.9378304198014,59.8199562049805));
#24625=CARTESIAN_POINT('Ctrl Pts',(-2.70005904694706,2.86202219870492,59.8257596879673));
#24626=CARTESIAN_POINT('Ctrl Pts',(-2.78208717217367,2.78236726364629,59.8315631709542));
#24627=CARTESIAN_POINT('Ctrl Pts',(-2.86059898584348,2.69915958071977,59.837366653941));
#24628=CARTESIAN_POINT('Ctrl Pts',(-2.93900947422837,2.61605928344372,59.8431626471051));
#24629=CARTESIAN_POINT('Ctrl Pts',(-3.01391238330406,2.52941565788114,59.8489586402692));
#24630=CARTESIAN_POINT('Ctrl Pts',(-3.08496744691924,2.43956243032406,59.8547546334334));
#24631=CARTESIAN_POINT('Ctrl Pts',(-3.1559427125746,2.34981011189123,59.8605441174424));
#24632=CARTESIAN_POINT('Ctrl Pts',(-3.22307846824127,2.25685569311537,59.8663336014514));
#24633=CARTESIAN_POINT('Ctrl Pts',(-3.2860724371803,2.16106847129007,59.8721230854604));
#24634=CARTESIAN_POINT('Ctrl Pts',(-3.3490272798566,2.06534074398576,59.8779089735558));
#24635=CARTESIAN_POINT('Ctrl Pts',(-3.40784521526477,1.96678406291508,59.8836948616511));
#24636=CARTESIAN_POINT('Ctrl Pts',(-3.46226560101986,1.86579899989111,59.8894807497465));
#24637=CARTESIAN_POINT('Ctrl Pts',(-3.51666611407386,1.76485081359897,59.8952645250082));
#24638=CARTESIAN_POINT('Ctrl Pts',(-3.56667206870605,1.66147638095618,59.9010483002699));
#24639=CARTESIAN_POINT('Ctrl Pts',(-3.61206779602966,1.55610257916551,59.9068320755315));
#24640=CARTESIAN_POINT('Ctrl Pts',(-3.65745856371834,1.45074028981484,59.9126152188964));
#24641=CARTESIAN_POINT('Ctrl Pts',(-3.6982399392204,1.3433794556174,59.9183983622613));
#24642=CARTESIAN_POINT('Ctrl Pts',(-3.73424395708088,1.23446792951662,59.9241815056262));
#24643=CARTESIAN_POINT('Ctrl Pts',(-3.77026966288204,1.12549079777353,59.9299681326154));
#24644=CARTESIAN_POINT('Ctrl Pts',(-3.80151212814882,1.01496151105195,59.9357547596045));
#24645=CARTESIAN_POINT('Ctrl Pts',(-3.8278530225736,0.903343919874489,59.9415413865937));
#24646=CARTESIAN_POINT('Ctrl Pts',(-3.8542021824487,0.791691304462895,59.9473298293556));
#24647=CARTESIAN_POINT('Ctrl Pts',(-3.87564662640377,0.678950120736433,
59.9531182721175));
#24648=CARTESIAN_POINT('Ctrl Pts',(-3.89211932283257,0.565593649923186,
59.9589067148794));
#24649=CARTESIAN_POINT('Ctrl Pts',(-3.90861163564203,0.452102189450431,
59.9647020507627));
#24650=CARTESIAN_POINT('Ctrl Pts',(-3.92012033260397,0.337994400458905,
59.9704973866461));
#24651=CARTESIAN_POINT('Ctrl Pts',(-3.92663034482843,0.22374792752712,59.9762927225294));
#24652=CARTESIAN_POINT('Ctrl Pts',(-3.93092869755112,0.148314637841466,
59.9801191973368));
#24653=CARTESIAN_POINT('Ctrl Pts',(-3.93304893094804,0.0728209313073551,
59.9839456721443));
#24654=CARTESIAN_POINT('Ctrl Pts',(-3.9329991429617,-0.00259643266824124,
59.9877721469517));
#24655=CARTESIAN_POINT('Origin',(-9.35406549764863E-15,0.,41.4527091182931));
#24656=CARTESIAN_POINT('',(3.08633327008855,-0.927720059309073,50.1419356690201));
#24657=CARTESIAN_POINT('Ctrl Pts',(3.08633327008855,-0.927720059309073,
50.1419356690201));
#24658=CARTESIAN_POINT('Ctrl Pts',(3.13685348859573,-0.759649713490565,
50.1534735349637));
#24659=CARTESIAN_POINT('Ctrl Pts',(3.17356710806874,-0.587711993181435,
50.16542241742));
#24660=CARTESIAN_POINT('Ctrl Pts',(3.2122200237151,-0.289034929219761,50.1857202293767));
#24661=CARTESIAN_POINT('Ctrl Pts',(3.22104582932805,-0.163606356509486,
50.1941131152217));
#24662=CARTESIAN_POINT('Ctrl Pts',(3.2232399976714,0.0225944212214418,50.2062819931546));
#24663=CARTESIAN_POINT('Ctrl Pts',(3.22224602972785,0.0831735796066807,
50.2101967129909));
#24664=CARTESIAN_POINT('Ctrl Pts',(3.21722795830564,0.195607969746975,50.2173784201255));
#24665=CARTESIAN_POINT('Ctrl Pts',(3.21365538769434,0.247462636076168,50.2206573898647));
#24666=CARTESIAN_POINT('Ctrl Pts',(3.20549926368679,0.334931489911482,50.2261354927619));
#24667=CARTESIAN_POINT('Ctrl Pts',(3.20157210717137,0.370595247070645,50.2283541934687));
#24668=CARTESIAN_POINT('Ctrl Pts',(3.19294606514685,0.438489784230139,50.232552046447));
#24669=CARTESIAN_POINT('Ctrl Pts',(3.18835255187181,0.470729208883945,50.2345341454286));
#24670=CARTESIAN_POINT('Ctrl Pts',(3.17489470238123,0.555916046152079,50.2397452301427));
#24671=CARTESIAN_POINT('Ctrl Pts',(3.16519459434201,0.608722172473708,50.2429483781026));
#24672=CARTESIAN_POINT('Ctrl Pts',(3.10582757262411,0.89189854007648,50.2600222140235));
#24673=CARTESIAN_POINT('Ctrl Pts',(3.03232745225429,1.11653350180377,50.273130271094));
#24674=CARTESIAN_POINT('Ctrl Pts',(2.89343794092022,1.42276206254468,50.2920934009401));
#24675=CARTESIAN_POINT('Ctrl Pts',(2.84762737509321,1.51236608636721,50.2977988153934));
#24676=CARTESIAN_POINT('Ctrl Pts',(2.77623870771935,1.63721913016987,50.3061675042645));
#24677=CARTESIAN_POINT('Ctrl Pts',(2.75401971170232,1.67432462506036,50.308710414296));
#24678=CARTESIAN_POINT('Ctrl Pts',(2.71275607925004,1.74018990650942,50.3133460520374));
#24679=CARTESIAN_POINT('Ctrl Pts',(2.69398338432274,1.76911270729488,50.3154252790585));
#24680=CARTESIAN_POINT('Ctrl Pts',(2.66297650078571,1.81524633915605,50.3188222229089));
#24681=CARTESIAN_POINT('Ctrl Pts',(2.6510304220032,1.83264856437271,50.3201225024542));
#24682=CARTESIAN_POINT('Ctrl Pts',(2.626605590923,1.86749041659045,50.3227669347323));
#24683=CARTESIAN_POINT('Ctrl Pts',(2.61412204161715,1.88492526914433,50.3241114260391));
#24684=CARTESIAN_POINT('Ctrl Pts',(2.5796599132161,1.93205515471179,50.3278011760857));
#24685=CARTESIAN_POINT('Ctrl Pts',(2.55734377894605,1.96149813185895,50.33016697198));
#24686=CARTESIAN_POINT('Ctrl Pts',(2.42039429742089,2.13587321435007,50.3445162771805));
#24687=CARTESIAN_POINT('Ctrl Pts',(2.29398182210057,2.27110132943294,50.3570511377045));
#24688=CARTESIAN_POINT('Ctrl Pts',(2.02288472296532,2.51524962568076,50.3816548591468));
#24689=CARTESIAN_POINT('Ctrl Pts',(1.87919905759162,2.62434162094821,50.3936820365134));
#24690=CARTESIAN_POINT('Ctrl Pts',(1.67376853888951,2.75474356212943,50.4093571201811));
#24691=CARTESIAN_POINT('Ctrl Pts',(1.6194135196018,2.78704394382615,50.4133765314517));
#24692=CARTESIAN_POINT('Ctrl Pts',(1.53111321739769,2.83606008353103,50.419707988439));
#24693=CARTESIAN_POINT('Ctrl Pts',(1.4977651725816,2.85381221542383,50.4220557201799));
#24694=CARTESIAN_POINT('Ctrl Pts',(1.43293144078974,2.88687548898488,50.4265395535711));
#24695=CARTESIAN_POINT('Ctrl Pts',(1.40149344491668,2.90226788485684,50.428678228009));
#24696=CARTESIAN_POINT('Ctrl Pts',(1.32654251036697,2.9374627470053,50.433697102474));
#24697=CARTESIAN_POINT('Ctrl Pts',(1.28282684860697,2.95681552568822,50.4365618254308));
#24698=CARTESIAN_POINT('Ctrl Pts',(1.12596652202807,3.02212300216649,50.4466392108348));
#24699=CARTESIAN_POINT('Ctrl Pts',(1.01065553947981,3.0626145086386,50.4536758175758));
#24700=CARTESIAN_POINT('Ctrl Pts',(0.697565891709428,3.1529393280572,50.4721644283239));
#24701=CARTESIAN_POINT('Ctrl Pts',(0.496912601079402,3.19072037772553,50.4833634460264));
#24702=CARTESIAN_POINT('Ctrl Pts',(0.204902367362186,3.21747502615022,50.5001312974058));
#24703=CARTESIAN_POINT('Ctrl Pts',(0.1154662521291,3.22192417344698,50.50533442865));
#24704=CARTESIAN_POINT('Ctrl Pts',(-0.00312374491549286,3.22287980685227,
50.5124542150706));
#24705=CARTESIAN_POINT('Ctrl Pts',(-0.0322172045423297,3.22272026765864,
50.514218522677));
#24706=CARTESIAN_POINT('Ctrl Pts',(-0.0811194089388643,3.2217898787515,
50.5172195995788));
#24707=CARTESIAN_POINT('Ctrl Pts',(-0.10093111086254,3.22123008758901,50.5184452959748));
#24708=CARTESIAN_POINT('Ctrl Pts',(-0.143319967612828,3.21964092412135,
50.5210908262252));
#24709=CARTESIAN_POINT('Ctrl Pts',(-0.165893164453825,3.21855676997438,
50.522513313459));
#24710=CARTESIAN_POINT('Ctrl Pts',(-0.232057580356062,3.2146811328333,50.5267192284953));
#24711=CARTESIAN_POINT('Ctrl Pts',(-0.27560408052192,3.21124080028935,50.5295338102967));
#24712=CARTESIAN_POINT('Ctrl Pts',(-0.520130950457913,3.18691216874051,
50.5455514951931));
#24713=CARTESIAN_POINT('Ctrl Pts',(-0.718860105977541,3.14804369002197,
50.5593488360495));
#24714=CARTESIAN_POINT('Ctrl Pts',(-1.08341101543709,3.04040230833409,50.5849400854615));
#24715=CARTESIAN_POINT('Ctrl Pts',(-1.24973669728024,2.97590325680127,50.5967368707795));
#24716=CARTESIAN_POINT('Ctrl Pts',(-1.45511732340627,2.87598323464553,50.611296362327));
#24717=CARTESIAN_POINT('Ctrl Pts',(-1.49981439933665,2.85292888320626,50.6144664192762));
#24718=CARTESIAN_POINT('Ctrl Pts',(-1.57475538528106,2.81202671375218,50.619786862669));
#24719=CARTESIAN_POINT('Ctrl Pts',(-1.60527934530082,2.79471414286986,50.621955523527));
#24720=CARTESIAN_POINT('Ctrl Pts',(-1.66684612988226,2.75845312799999,50.6263353849259));
#24721=CARTESIAN_POINT('Ctrl Pts',(-1.69786318909509,2.73947083167311,50.6285449572063));
#24722=CARTESIAN_POINT('Ctrl Pts',(-1.77686688864992,2.68926356531442,50.6341855497439));
#24723=CARTESIAN_POINT('Ctrl Pts',(-1.82435576520394,2.65727700792887,50.6375881702418));
#24724=CARTESIAN_POINT('Ctrl Pts',(-2.04138047685718,2.50253603299261,50.6532414743377));
#24725=CARTESIAN_POINT('Ctrl Pts',(-2.19955331342346,2.36471892350634,50.6649119598523));
#24726=CARTESIAN_POINT('Ctrl Pts',(-2.46501678096647,2.08357034282935,50.6865539904165));
#24727=CARTESIAN_POINT('Ctrl Pts',(-2.57591155249613,1.94479767804143,50.6964910790293));
#24728=CARTESIAN_POINT('Ctrl Pts',(-2.6930441691688,1.77050796956148,50.7090249300383));
#24729=CARTESIAN_POINT('Ctrl Pts',(-2.71085700133695,1.74311201550285,50.7109968903079));
#24730=CARTESIAN_POINT('Ctrl Pts',(-2.73908901553656,1.6982118883219,50.71423982233));
#24731=CARTESIAN_POINT('Ctrl Pts',(-2.74976478067043,1.68087057179405,50.7154949397547));
#24732=CARTESIAN_POINT('Ctrl Pts',(-2.77127601933335,1.64517507374303,50.718086196289));
#24733=CARTESIAN_POINT('Ctrl Pts',(-2.78209496726725,1.62681262971739,50.7194230991081));
#24734=CARTESIAN_POINT('Ctrl Pts',(-2.8111454408908,1.57636937556066,50.7231034608115));
#24735=CARTESIAN_POINT('Ctrl Pts',(-2.82900885013162,1.54408152604282,50.7254676619173));
#24736=CARTESIAN_POINT('Ctrl Pts',(-2.93264936737491,1.34891500678954,50.7397771430256));
#24737=CARTESIAN_POINT('Ctrl Pts',(-3.00489103698888,1.17924753251186,50.7522739254275));
#24738=CARTESIAN_POINT('Ctrl Pts',(-3.1051649512933,0.873515310599367,50.7739931373521));
#24739=CARTESIAN_POINT('Ctrl Pts',(-3.13965133148799,0.740049616714836,
50.7832303132723));
#24740=CARTESIAN_POINT('Ctrl Pts',(-3.17739305073633,0.542503971100684,
50.7964072906922));
#24741=CARTESIAN_POINT('Ctrl Pts',(-3.18745101811869,0.479889564815537,
50.8005145078508));
#24742=CARTESIAN_POINT('Ctrl Pts',(-3.20258902322406,0.363884727118246,
50.8079933740099));
#24743=CARTESIAN_POINT('Ctrl Pts',(-3.20819653648734,0.31058666027832,50.8113792965692));
#24744=CARTESIAN_POINT('Ctrl Pts',(-3.21533538737369,0.221411086604464,
50.8169639182265));
#24745=CARTESIAN_POINT('Ctrl Pts',(-3.21760089447557,0.185604877272735,
50.819184766121));
#24746=CARTESIAN_POINT('Ctrl Pts',(-3.22094185891495,0.113790316646707,
50.8235983556407));
#24747=CARTESIAN_POINT('Ctrl Pts',(-3.22201242244565,0.0777869219772379,
50.8257906351577));
#24748=CARTESIAN_POINT('Ctrl Pts',(-3.22318388300327,-0.0125848122350477,
50.8312466371793));
#24749=CARTESIAN_POINT('Ctrl Pts',(-3.22251307841298,-0.0669528803071431,
50.8344863849312));
#24750=CARTESIAN_POINT('Ctrl Pts',(-3.21152665457355,-0.358685216055101,
50.851686127683));
#24751=CARTESIAN_POINT('Ctrl Pts',(-3.17636421075039,-0.594372392630117,
50.8648583487903));
#24752=CARTESIAN_POINT('Ctrl Pts',(-3.08898906648665,-0.924718045923707,
50.8840560188992));
#24753=CARTESIAN_POINT('Ctrl Pts',(-3.05750694141818,-1.02401455906482,
50.889938640144));
#24754=CARTESIAN_POINT('Ctrl Pts',(-3.00595299420508,-1.16288558383963,
50.8985371769));
#24755=CARTESIAN_POINT('Ctrl Pts',(-2.98978532652108,-1.20384369531999,
50.9011209426701));
#24756=CARTESIAN_POINT('Ctrl Pts',(-2.95932421911207,-1.27660988032735,
50.9058188869767));
#24757=CARTESIAN_POINT('Ctrl Pts',(-2.94534384396209,-1.30854195213678,
50.9079184760733));
#24758=CARTESIAN_POINT('Ctrl Pts',(-2.92214512621198,-1.35927313639041,
50.9113250061042));
#24759=CARTESIAN_POINT('Ctrl Pts',(-2.91325636743957,-1.37822091096904,
50.9126134084705));
#24760=CARTESIAN_POINT('Ctrl Pts',(-2.89510964291145,-1.41594346140055,
50.915213388997));
#24761=CARTESIAN_POINT('Ctrl Pts',(-2.8858520432938,-1.43471727358412,50.9165249220915));
#24762=CARTESIAN_POINT('Ctrl Pts',(-2.86062661436476,-1.48464075896815,
50.9200570934682));
#24763=CARTESIAN_POINT('Ctrl Pts',(-2.84433346285337,-1.51562189639145,
50.9222958825958));
#24764=CARTESIAN_POINT('Ctrl Pts',(-2.72864510662595,-1.72716368864217,
50.9378768465314));
#24765=CARTESIAN_POINT('Ctrl Pts',(-2.61263775555365,-1.89808128277749,
50.9519269314204));
#24766=CARTESIAN_POINT('Ctrl Pts',(-2.36102051270327,-2.20161557159665,
50.9784949113271));
#24767=CARTESIAN_POINT('Ctrl Pts',(-2.22845255021441,-2.33571126030287,
50.9909899126789));
#24768=CARTESIAN_POINT('Ctrl Pts',(-2.04619088503711,-2.49034133099285,
51.0062308344743));
#24769=CARTESIAN_POINT('Ctrl Pts',(-2.00668919870367,-2.52227992252108,
51.0094335987568));
#24770=CARTESIAN_POINT('Ctrl Pts',(-1.93844643854729,-2.57483826159254,
51.0148026120983));
#24771=CARTESIAN_POINT('Ctrl Pts',(-1.91009196339019,-2.59594212507118,
51.0169874751686));
#24772=CARTESIAN_POINT('Ctrl Pts',(-1.85170995302399,-2.63792050912542,
51.0213962416543));
#24773=CARTESIAN_POINT('Ctrl Pts',(-1.82166279008571,-2.65875896046727,
51.0236185659754));
#24774=CARTESIAN_POINT('Ctrl Pts',(-1.74348776548612,-2.71102771996091,
51.0292865800497));
#24775=CARTESIAN_POINT('Ctrl Pts',(-1.69486101335956,-2.74169065105194,
51.0327038878865));
#24776=CARTESIAN_POINT('Ctrl Pts',(-1.49421570631325,-2.8608335058814,51.0464129326366));
#24777=CARTESIAN_POINT('Ctrl Pts',(-1.33589178380515,-2.93810311525452,
51.056322416913));
#24778=CARTESIAN_POINT('Ctrl Pts',(-1.03787918618702,-3.05445038454346,
51.0742508374183));
#24779=CARTESIAN_POINT('Ctrl Pts',(-0.900364279575766,-3.09777344529481,
51.0822731865236));
#24780=CARTESIAN_POINT('Ctrl Pts',(-0.709491233437202,-3.14411936337167,
51.0935803218847));
#24781=CARTESIAN_POINT('Ctrl Pts',(-0.658269286571034,-3.15524094146588,
51.0966318516028));
#24782=CARTESIAN_POINT('Ctrl Pts',(-0.568185561978951,-3.17251142354894,
51.1020634826264));
#24783=CARTESIAN_POINT('Ctrl Pts',(-0.529439230667669,-3.17920703288653,
51.1044205117754));
#24784=CARTESIAN_POINT('Ctrl Pts',(-0.49058209429631,-3.18519179505032,
51.1068136617517));
#24785=CARTESIAN_POINT('',(1.91684063918175,2.59072181572651,50.1419356690201));
#24786=CARTESIAN_POINT('Origin',(-1.041818884589E-14,0.,50.1419356690201));
#24787=CARTESIAN_POINT('',(-3.22274873162613,0.00285924854630651,50.5811622197476));
#24788=CARTESIAN_POINT('Ctrl Pts',(-3.22274873162613,0.00285924854630654,
50.5811622197476));
#24789=CARTESIAN_POINT('Ctrl Pts',(-3.22262606019522,0.141126066550874,
50.5726197745096));
#24790=CARTESIAN_POINT('Ctrl Pts',(-3.21360167581526,0.279007275896255,
50.5640773292716));
#24791=CARTESIAN_POINT('Ctrl Pts',(-3.19584473577038,0.415564660851703,
50.5555348840336));
#24792=CARTESIAN_POINT('Ctrl Pts',(-3.1829722359087,0.514558908425243,50.5493422278177));
#24793=CARTESIAN_POINT('Ctrl Pts',(-3.16551157989265,0.612858278864528,
50.5431495716017));
#24794=CARTESIAN_POINT('Ctrl Pts',(-3.14354197865906,0.710113646473836,
50.5369569153858));
#24795=CARTESIAN_POINT('Ctrl Pts',(-3.1218293532884,0.80623142939279,50.5308366939473));
#24796=CARTESIAN_POINT('Ctrl Pts',(-3.09566276943955,0.90153560505576,50.5247164725087));
#24797=CARTESIAN_POINT('Ctrl Pts',(-3.06511720146087,0.995577271641297,
50.5185962510702));
#24798=CARTESIAN_POINT('Ctrl Pts',(-3.03461292647625,1.08949180809844,50.5124843032466));
#24799=CARTESIAN_POINT('Ctrl Pts',(-2.99974156371624,1.18214680967076,50.506372355423));
#24800=CARTESIAN_POINT('Ctrl Pts',(-2.96062902974355,1.27310380988347,50.5002604075994));
#24801=CARTESIAN_POINT('Ctrl Pts',(-2.92155733029939,1.36396584856231,50.4941548408124));
#24802=CARTESIAN_POINT('Ctrl Pts',(-2.87825343276076,1.45313300486155,50.4880492740253));
#24803=CARTESIAN_POINT('Ctrl Pts',(-2.83089263567421,1.54018325136511,50.4819437072382));
#24804=CARTESIAN_POINT('Ctrl Pts',(-2.78356365430523,1.62717501983984,50.4758422420077));
#24805=CARTESIAN_POINT('Ctrl Pts',(-2.73218339858752,1.71205231641932,50.4697407767772));
#24806=CARTESIAN_POINT('Ctrl Pts',(-2.67697431528342,1.79441524676228,50.4636393115467));
#24807=CARTESIAN_POINT('Ctrl Pts',(-2.62178396127082,1.87675023606295,50.4575399161952));
#24808=CARTESIAN_POINT('Ctrl Pts',(-2.56276760522076,1.9565721859484,50.4514405208437));
#24809=CARTESIAN_POINT('Ctrl Pts',(-2.50019191985115,2.03350877215002,50.4453411254922));
#24810=CARTESIAN_POINT('Ctrl Pts',(-2.43762003683202,2.11044068337501,50.4392421007645));
#24811=CARTESIAN_POINT('Ctrl Pts',(-2.3714895334439,2.18448723608768,50.4331430760367));
#24812=CARTESIAN_POINT('Ctrl Pts',(-2.30210770264219,2.25530877884505,50.427044051309));
#24813=CARTESIAN_POINT('Ctrl Pts',(-2.23271076539457,2.32614574151556,50.4209436986459));
#24814=CARTESIAN_POINT('Ctrl Pts',(-2.16006140450322,2.39375598379192,50.4148433459829));
#24815=CARTESIAN_POINT('Ctrl Pts',(-2.08450332668258,2.45783714748339,50.4087429933198));
#24816=CARTESIAN_POINT('Ctrl Pts',(-2.00885443188885,2.52199533347991,50.4026353083426));
#24817=CARTESIAN_POINT('Ctrl Pts',(-1.93029017833084,2.58261568575184,50.3965276233653));
#24818=CARTESIAN_POINT('Ctrl Pts',(-1.84918674915733,2.63943666892028,50.3904199383881));
#24819=CARTESIAN_POINT('Ctrl Pts',(-1.768032317762,2.69629338419545,50.3843084125683));
#24820=CARTESIAN_POINT('Ctrl Pts',(-1.68433590672813,2.74934573955533,50.3781968867485));
#24821=CARTESIAN_POINT('Ctrl Pts',(-1.59850005921721,2.79837723032164,50.3720853609287));
#24822=CARTESIAN_POINT('Ctrl Pts',(-1.51250737215979,2.8474983115912,50.3659626681085));
#24823=CARTESIAN_POINT('Ctrl Pts',(-1.4243678359665,2.89258365598401,50.3598399752884));
#24824=CARTESIAN_POINT('Ctrl Pts',(-1.33450590411258,2.93346408779598,50.3537172824682));
#24825=CARTESIAN_POINT('Ctrl Pts',(-1.26468810812105,2.96522594278185,50.3489602857131));
#24826=CARTESIAN_POINT('Ctrl Pts',(-1.19383105609949,2.99445049063284,50.344203288958));
#24827=CARTESIAN_POINT('Ctrl Pts',(-1.12213954345542,3.02107934478949,50.3394462922029));
#24828=CARTESIAN_POINT('Ctrl Pts',(-1.0265657642302,3.05657894766191,50.3331046188182));
#24829=CARTESIAN_POINT('Ctrl Pts',(-0.929169554246279,3.08758984486248,
50.3267629454334));
#24830=CARTESIAN_POINT('Ctrl Pts',(-0.830398224371547,3.11392940694882,
50.3204212720487));
#24831=CARTESIAN_POINT('Ctrl Pts',(-0.731773318293886,3.14022992188757,
50.314088999893));
#24832=CARTESIAN_POINT('Ctrl Pts',(-0.631777738060152,3.16187277887449,
50.3077567277373));
#24833=CARTESIAN_POINT('Ctrl Pts',(-0.530876565142943,3.1787242150086,50.3014244555816));
#24834=CARTESIAN_POINT('Ctrl Pts',(-0.424986417318397,3.19640885644247,
50.2947790894749));
#24835=CARTESIAN_POINT('Ctrl Pts',(-0.31809923935474,3.20881592952247,50.2881337233682));
#24836=CARTESIAN_POINT('Ctrl Pts',(-0.210769145412158,3.21585042093724,
50.2814883572615));
#24837=CARTESIAN_POINT('Ctrl Pts',(-0.108748201975073,3.22253694681617,
50.2751717083629));
#24838=CARTESIAN_POINT('Ctrl Pts',(-0.00632757651942337,3.22436963666028,
50.2688550594643));
#24839=CARTESIAN_POINT('Ctrl Pts',(0.0960087647114913,3.22131958669092,
50.2625384105657));
#24840=CARTESIAN_POINT('Ctrl Pts',(0.198275729533058,3.21827160442804,50.2562260438841));
#24841=CARTESIAN_POINT('Ctrl Pts',(0.300458119624661,3.21034748182014,50.2499136772025));
#24842=CARTESIAN_POINT('Ctrl Pts',(0.402071203165288,3.19757037609576,50.2436013105208));
#24843=CARTESIAN_POINT('Ctrl Pts',(0.503636990654584,3.18479921750562,50.2372918819453));
#24844=CARTESIAN_POINT('Ctrl Pts',(0.604633597356732,3.16717962291273,50.2309824533698));
#24845=CARTESIAN_POINT('Ctrl Pts',(0.704581288421044,3.14478660174374,50.2246730247942));
#24846=CARTESIAN_POINT('Ctrl Pts',(0.804503681232043,3.12239924858284,50.2183651932293));
#24847=CARTESIAN_POINT('Ctrl Pts',(0.903377291858967,3.09524096409745,50.2120573616644));
#24848=CARTESIAN_POINT('Ctrl Pts',(1.00073308481727,3.06343775119588,50.2057495300994));
#24849=CARTESIAN_POINT('Ctrl Pts',(1.09811106106199,3.03162729168104,50.1994402612452));
#24850=CARTESIAN_POINT('Ctrl Pts',(1.19397014176976,2.99516991119222,50.1931309923911));
#24851=CARTESIAN_POINT('Ctrl Pts',(1.28785719676933,2.95424125677464,50.1868217235369));
#24852=CARTESIAN_POINT('Ctrl Pts',(1.38175496784341,2.913307930845,50.1805117345558));
#24853=CARTESIAN_POINT('Ctrl Pts',(1.47367989593232,2.86790248302421,50.1742017455747));
#24854=CARTESIAN_POINT('Ctrl Pts',(1.56320057919852,2.81824795071218,50.1678917565936));
#24855=CARTESIAN_POINT('Ctrl Pts',(1.65278085478603,2.76856036426409,50.1615775671654));
#24856=CARTESIAN_POINT('Ctrl Pts',(1.73995333823911,2.71461824789198,50.1552633777373));
#24857=CARTESIAN_POINT('Ctrl Pts',(1.82431303210882,2.65668957979247,50.1489491883091));
#24858=CARTESIAN_POINT('Ctrl Pts',(1.85554735742454,2.63524138834548,50.1466113485463));
#24859=CARTESIAN_POINT('Ctrl Pts',(1.88639638224608,2.61324711681045,50.1442735087836));
#24860=CARTESIAN_POINT('Ctrl Pts',(1.91684063918178,2.59072181572649,50.1419356690208));
#24861=CARTESIAN_POINT('Ctrl Pts',(-3.22274870145484,0.00289305568448681,
50.5817658723809));
#24862=CARTESIAN_POINT('Ctrl Pts',(-3.22294593790816,-0.216820490517224,
50.5940710088782));
#24863=CARTESIAN_POINT('Ctrl Pts',(-3.20067541107489,-0.435964380627837,
50.6063421177884));
#24864=CARTESIAN_POINT('Ctrl Pts',(-3.14577957458053,-0.702062716046087,
50.622387585657));
#24865=CARTESIAN_POINT('Ctrl Pts',(-3.13404357799902,-0.752722786275725,
50.6254923413925));
#24866=CARTESIAN_POINT('Ctrl Pts',(-3.1121464086732,-0.837824431242347,
50.6308043780983));
#24867=CARTESIAN_POINT('Ctrl Pts',(-3.1026256862327,-0.872421193767486,
50.6329912168688));
#24868=CARTESIAN_POINT('Ctrl Pts',(-3.08336780646881,-0.938094142503432,
50.6371977604574));
#24869=CARTESIAN_POINT('Ctrl Pts',(-3.07373335171097,-0.969195961374662,
50.6392139493982));
#24870=CARTESIAN_POINT('Ctrl Pts',(-3.04697821554796,-1.05115185498848,
50.6445928861539));
#24871=CARTESIAN_POINT('Ctrl Pts',(-3.02905646767004,-1.10173174930548,
50.6479808315215));
#24872=CARTESIAN_POINT('Ctrl Pts',(-2.92568908737845,-1.37184214798474,
50.6664531184552));
#24873=CARTESIAN_POINT('Ctrl Pts',(-2.81764048990057,-1.58192199893996,
50.682265881946));
#24874=CARTESIAN_POINT('Ctrl Pts',(-2.63213206238254,-1.86229357301267,
50.7048793763472));
#24875=CARTESIAN_POINT('Ctrl Pts',(-2.57266218212015,-1.94362229042128,
50.7116337837267));
#24876=CARTESIAN_POINT('Ctrl Pts',(-2.48233007528408,-2.05573037319448,
50.7211120505662));
#24877=CARTESIAN_POINT('Ctrl Pts',(-2.45450345960228,-2.08887602857737,
50.7239365132111));
#24878=CARTESIAN_POINT('Ctrl Pts',(-2.40331016691311,-2.14741883010464,
50.7289513877557));
#24879=CARTESIAN_POINT('Ctrl Pts',(-2.38018727660624,-2.17302004890099,
50.7311538498141));
#24880=CARTESIAN_POINT('Ctrl Pts',(-2.34225760734563,-2.21368301599351,
50.7346605935914));
#24881=CARTESIAN_POINT('Ctrl Pts',(-2.32770663230663,-2.22897848471628,
50.7359816691638));
#24882=CARTESIAN_POINT('Ctrl Pts',(-2.29807837871757,-2.25951607225457,
50.7386212568842));
#24883=CARTESIAN_POINT('Ctrl Pts',(-2.28299724290356,-2.2747528999986,50.7399392973703));
#24884=CARTESIAN_POINT('Ctrl Pts',(-2.24153356794207,-2.31581687015043,
50.7434980565896));
#24885=CARTESIAN_POINT('Ctrl Pts',(-2.2148566712145,-2.34134377961174,50.7457175606291));
#24886=CARTESIAN_POINT('Ctrl Pts',(-2.05150091703217,-2.49236629606847,
50.7589359388627));
#24887=CARTESIAN_POINT('Ctrl Pts',(-1.90461716824201,-2.60633731052415,
50.7692977867751));
#24888=CARTESIAN_POINT('Ctrl Pts',(-1.57824147938978,-2.81717334016311,
50.7910864900979));
#24889=CARTESIAN_POINT('Ctrl Pts',(-1.39775205847823,-2.91094318019762,
50.8024888642781));
#24890=CARTESIAN_POINT('Ctrl Pts',(-1.16193759080524,-3.00643787871655,
50.8175239224694));
#24891=CARTESIAN_POINT('Ctrl Pts',(-1.11376821521377,-3.02461363007976,
50.8205995517256));
#24892=CARTESIAN_POINT('Ctrl Pts',(-1.03159753188286,-3.05339002568585,
50.8258651688267));
#24893=CARTESIAN_POINT('Ctrl Pts',(-0.997817527671875,-3.06459526573084,
50.8280351190038));
#24894=CARTESIAN_POINT('Ctrl Pts',(-0.92889730297866,-3.08619666055815,
50.8324763958555));
#24895=CARTESIAN_POINT('Ctrl Pts',(-0.893751576129889,-3.09655743895753,
50.8347484926124));
#24896=CARTESIAN_POINT('Ctrl Pts',(-0.803271344232077,-3.12156186672095,
50.8406195768897));
#24897=CARTESIAN_POINT('Ctrl Pts',(-0.74771139666121,-3.13533416857717,
50.8442455191745));
#24898=CARTESIAN_POINT('Ctrl Pts',(-0.625114591955927,-3.16227978483002,
50.8522958948133));
#24899=CARTESIAN_POINT('Ctrl Pts',(-0.558001847543211,-3.17480783705022,
50.8567349905582));
#24900=CARTESIAN_POINT('Ctrl Pts',(-0.490581718709063,-3.18519185289811,
50.8612231915357));
#24901=CARTESIAN_POINT('Ctrl Pts',(0.500000469481149,-0.249903141644244,
19.1419331299125));
#24902=CARTESIAN_POINT('Ctrl Pts',(0.499985698745681,-0.249901829979438,
19.1419329611828));
#24903=CARTESIAN_POINT('Ctrl Pts',(0.499943925319444,-0.225581315070387,
19.1419270874343));
#24904=CARTESIAN_POINT('Ctrl Pts',(0.499905220847302,-0.0968326406578691,
19.1419269431202));
#24905=CARTESIAN_POINT('Ctrl Pts',(0.499905354496604,0.0576085255888102,
19.1419269231968));
#24906=CARTESIAN_POINT('Ctrl Pts',(0.499924487070724,0.161824164743378,
19.1419270312494));
#24907=CARTESIAN_POINT('Ctrl Pts',(0.499957970023252,0.233166151920814,
19.1419290385144));
#24908=CARTESIAN_POINT('Ctrl Pts',(0.499985738380631,0.249901825150789,
19.1419329686928));
#24909=CARTESIAN_POINT('Ctrl Pts',(0.500000469481149,0.249903141644244,
19.1419331299125));
#24910=CARTESIAN_POINT('Ctrl Pts',(0.50000579870514,-1.07273214192946,19.141904307727));
#24911=CARTESIAN_POINT('Ctrl Pts',(0.617766930419002,-1.05838545165019,
19.1642183664756));
#24912=CARTESIAN_POINT('Ctrl Pts',(0.961751310472008,-0.926346421353011,
19.2125872476967));
#24913=CARTESIAN_POINT('Ctrl Pts',(1.28046455179809,-0.399644119496195,
19.2137755873294));
#24914=CARTESIAN_POINT('Ctrl Pts',(1.27936400811516,0.237312123921118,19.2139396493409));
#24915=CARTESIAN_POINT('Ctrl Pts',(1.12181620701011,0.66571216146587,19.2130498921711));
#24916=CARTESIAN_POINT('Ctrl Pts',(0.846099822863789,0.968022143869402,
19.1965205779324));
#24917=CARTESIAN_POINT('Ctrl Pts',(0.617440555450805,1.05842521350129,19.1641565230633));
#24918=CARTESIAN_POINT('Ctrl Pts',(0.500005798705135,1.07273214192946,19.141904307727));
#24919=CARTESIAN_POINT('Ctrl Pts',(0.374651423361831,-2.49809918431546,
19.8198617495831));
#24920=CARTESIAN_POINT('Ctrl Pts',(0.709304215540434,-2.46080219696565,
19.8562164416348));
#24921=CARTESIAN_POINT('Ctrl Pts',(1.68368133342979,-2.14239899065394,19.9350988623808));
#24922=CARTESIAN_POINT('Ctrl Pts',(2.57589462505932,-0.923785761636194,
19.9392568404695));
#24923=CARTESIAN_POINT('Ctrl Pts',(2.57299273739104,0.549303191743538,19.9396328253395));
#24924=CARTESIAN_POINT('Ctrl Pts',(2.13168844086288,1.54026272327316,19.9369090432763));
#24925=CARTESIAN_POINT('Ctrl Pts',(1.35624450163379,2.24246685246118,19.9089996947345));
#24926=CARTESIAN_POINT('Ctrl Pts',(0.708376725350636,2.46090556556345,19.8561156846084));
#24927=CARTESIAN_POINT('Ctrl Pts',(0.374651423361818,2.49809918431547,19.8198617495831));
#24928=CARTESIAN_POINT('Ctrl Pts',(0.11219973762821,-3.,21.2392862649499));
#24929=CARTESIAN_POINT('Ctrl Pts',(0.545410746577862,-2.98330036684517,
21.254809362827));
#24930=CARTESIAN_POINT('Ctrl Pts',(1.84334280227898,-2.65791740981921,21.2909019746354));
#24931=CARTESIAN_POINT('Ctrl Pts',(3.03119172810009,-1.14304804845867,21.2989264987267));
#24932=CARTESIAN_POINT('Ctrl Pts',(3.02359011539719,0.679678385818526,21.298996417349));
#24933=CARTESIAN_POINT('Ctrl Pts',(2.443255756993,1.90810517204302,21.2948760084178));
#24934=CARTESIAN_POINT('Ctrl Pts',(1.40427963606369,2.75990594888198,21.2788873186408));
#24935=CARTESIAN_POINT('Ctrl Pts',(0.54421010229727,2.98334664987728,21.2547663405623));
#24936=CARTESIAN_POINT('Ctrl Pts',(0.112199737628194,3.,21.2392862649499));
#24937=CARTESIAN_POINT('Ctrl Pts',(1.76595225516049E-15,-3.,21.846099125618));
#24938=CARTESIAN_POINT('Ctrl Pts',(0.443076107560806,-3.,21.8529261923905));
#24939=CARTESIAN_POINT('Ctrl Pts',(1.79348225283645,-2.70799686462405,21.8711225067259));
#24940=CARTESIAN_POINT('Ctrl Pts',(3.03256681393803,-1.16243291399857,21.8807881756829));
#24941=CARTESIAN_POINT('Ctrl Pts',(3.02252392263477,0.691564152912778,21.8807213059649));
#24942=CARTESIAN_POINT('Ctrl Pts',(2.42127463370821,1.94262419136537,21.876015661462));
#24943=CARTESIAN_POINT('Ctrl Pts',(1.33503220965341,2.79906458058143,21.8649899286495));
#24944=CARTESIAN_POINT('Ctrl Pts',(0.441848122160112,3.,21.8529072711754));
#24945=CARTESIAN_POINT('Ctrl Pts',(-1.48930058907191E-14,3.,21.846099125618));
#24946=CARTESIAN_POINT('',(0.500000234886957,0.250003172331033,19.141934398682));
#24947=CARTESIAN_POINT('',(0.499951141785782,2.95746651812731,21.8534599521462));
#24948=CARTESIAN_POINT('Ctrl Pts',(0.500000469773915,0.250006344662067,
19.1419331283439));
#24949=CARTESIAN_POINT('Ctrl Pts',(0.500000469773915,0.267897236481739,
19.141933220399));
#24950=CARTESIAN_POINT('Ctrl Pts',(0.5,0.285781329534287,19.142122715469));
#24951=CARTESIAN_POINT('Ctrl Pts',(0.5,0.647586433160097,19.1497655967622));
#24952=CARTESIAN_POINT('Ctrl Pts',(0.500000000105589,0.988807525496054,
19.2265788097412));
#24953=CARTESIAN_POINT('Ctrl Pts',(0.500000000105589,1.62419548103609,19.4977571124707));
#24954=CARTESIAN_POINT('Ctrl Pts',(0.500000000129562,1.9184510407218,19.6932861554111));
#24955=CARTESIAN_POINT('Ctrl Pts',(0.500000000129562,2.44456182345909,20.2134324331408));
#24956=CARTESIAN_POINT('Ctrl Pts',(0.499999999835962,2.62278482582048,20.5122279848983));
#24957=CARTESIAN_POINT('Ctrl Pts',(0.499999999835962,2.81085326210919,20.9561451281499));
#24958=CARTESIAN_POINT('Ctrl Pts',(0.499999999999019,2.86545844391283,21.1318314683005));
#24959=CARTESIAN_POINT('Ctrl Pts',(0.499999999999019,2.93869926777347,21.4893795880377));
#24960=CARTESIAN_POINT('Ctrl Pts',(0.499999999999999,2.95754601494669,21.6714083748326));
#24961=CARTESIAN_POINT('Ctrl Pts',(0.499999999999999,2.95745819674082,21.8534588950701));
#24962=CARTESIAN_POINT('',(0.500115911061517,-2.95873774531605,21.8534555877921));
#24963=CARTESIAN_POINT('Ctrl Pts',(0.499951141785782,2.95746651812731,21.8534599521462));
#24964=CARTESIAN_POINT('Ctrl Pts',(0.773041654135478,2.91095214720846,21.8573003801108));
#24965=CARTESIAN_POINT('Ctrl Pts',(1.47173378593617,2.69128316033362,21.8663774964905));
#24966=CARTESIAN_POINT('Ctrl Pts',(2.42127463370821,1.94262419136537,21.876015661462));
#24967=CARTESIAN_POINT('Ctrl Pts',(3.02252392263477,0.691564152912778,21.8807213059649));
#24968=CARTESIAN_POINT('Ctrl Pts',(3.03256681393803,-1.16243291399857,21.8807881756829));
#24969=CARTESIAN_POINT('Ctrl Pts',(1.91000174505638,-2.56265704491053,21.8720314348768));
#24970=CARTESIAN_POINT('Ctrl Pts',(0.775090389504859,-2.91314338265178,
21.8573170895367));
#24971=CARTESIAN_POINT('Ctrl Pts',(0.500115911061517,-2.95873774531605,
21.8534555877921));
#24972=CARTESIAN_POINT('',(0.500000234886961,-0.250003167770416,19.141934398682));
#24973=CARTESIAN_POINT('Ctrl Pts',(0.500000000000001,-2.95875696259953,
21.8534539603318));
#24974=CARTESIAN_POINT('Ctrl Pts',(0.500000000000001,-2.95871463188845,
21.67146735895));
#24975=CARTESIAN_POINT('Ctrl Pts',(0.499999999998967,-2.93976167349618,
21.4895125652458));
#24976=CARTESIAN_POINT('Ctrl Pts',(0.499999999998967,-2.86636194368596,
21.132115489418));
#24977=CARTESIAN_POINT('Ctrl Pts',(0.499999999825066,-2.81170123842746,
20.9565020048332));
#24978=CARTESIAN_POINT('Ctrl Pts',(0.499999999825066,-2.6234386591811,20.5124823848305));
#24979=CARTESIAN_POINT('Ctrl Pts',(0.50000000005703,-2.44498892439426,20.2134765044685));
#24980=CARTESIAN_POINT('Ctrl Pts',(0.500000000057029,-1.91831791688,19.6930503466231));
#24981=CARTESIAN_POINT('Ctrl Pts',(0.500000000109665,-1.62378550938661,
19.4974427643328));
#24982=CARTESIAN_POINT('Ctrl Pts',(0.500000000109665,-0.988277937574047,
19.2264560225243));
#24983=CARTESIAN_POINT('Ctrl Pts',(0.5,-0.647284047492248,19.1497487087651));
#24984=CARTESIAN_POINT('Ctrl Pts',(0.5,-0.285729480193629,19.1421221661827));
#24985=CARTESIAN_POINT('Ctrl Pts',(0.500000469773922,-0.267871311676459,
19.1419332201691));
#24986=CARTESIAN_POINT('Ctrl Pts',(0.500000469773922,-0.250006335540832,
19.1419331283438));
#24987=CARTESIAN_POINT('',(0.5,1.66533453693774E-16,19.1419356690201));
#24988=CARTESIAN_POINT('Origin',(0.5,2.22044604925031E-16,0.));
#24989=CARTESIAN_POINT('',(0.500000000000001,-2.95803989154981,24.3207730140306));
#24990=CARTESIAN_POINT('',(0.500000000000001,-2.95803989154981,39.1419356690201));
#24991=CARTESIAN_POINT('',(0.499999999999999,2.95803989154981,24.3207730140306));
#24992=CARTESIAN_POINT('Origin',(0.5,2.22044604925031E-16,0.));
#24993=CARTESIAN_POINT('',(0.499999999999999,2.95803989154981,39.1419356690201));
#24994=CARTESIAN_POINT('Origin',(-9.07107736682793E-15,0.,39.1419356690201));
#24995=CARTESIAN_POINT('',(-0.499940024180695,-2.95805002868819,21.8534578776881));
#24996=CARTESIAN_POINT('',(-2.99999997692161,-0.000372116104727271,21.880545165042));
#24997=CARTESIAN_POINT('Ctrl Pts',(-0.499940024180695,-2.95805002868819,
21.8534578776881));
#24998=CARTESIAN_POINT('Ctrl Pts',(-0.59094175739541,-2.94266982610114,
21.8547370166103));
#24999=CARTESIAN_POINT('Ctrl Pts',(-0.68138174282413,-2.92306085113225,
21.8559764996555));
#25000=CARTESIAN_POINT('Ctrl Pts',(-0.770826195716954,-2.89928042382874,
21.8571725494205));
#25001=CARTESIAN_POINT('Ctrl Pts',(-0.860457040630935,-2.87545044083154,
21.8583710916166));
#25002=CARTESIAN_POINT('Ctrl Pts',(-0.949087732495046,-2.84743164098335,
21.8595260193239));
#25003=CARTESIAN_POINT('Ctrl Pts',(-1.03628975548556,-2.81533364677718,
21.860633531475));
#25004=CARTESIAN_POINT('Ctrl Pts',(-1.12349177847607,-2.78323565257101,
21.8617410436262));
#25005=CARTESIAN_POINT('Ctrl Pts',(-1.20926467836655,-2.74705858859954,
21.8628011402213));
#25006=CARTESIAN_POINT('Ctrl Pts',(-1.29319483960894,-2.70696270879538,
21.8638100201928));
#25007=CARTESIAN_POINT('Ctrl Pts',(-1.38514368549922,-2.66303607004747,
21.8649152885213));
#25008=CARTESIAN_POINT('Ctrl Pts',(-1.47489907524035,-2.61439837108066,
21.8659590862581));
#25009=CARTESIAN_POINT('Ctrl Pts',(-1.56199166539876,-2.56128523152437,
21.8669430860832));
#25010=CARTESIAN_POINT('Ctrl Pts',(-1.64895250576959,-2.50825243915768,
21.8679255973573));
#25011=CARTESIAN_POINT('Ctrl Pts',(-1.73325829906695,-2.45075788734509,
21.8688484915021));
#25012=CARTESIAN_POINT('Ctrl Pts',(-1.81446583003367,-2.38908219859432,
21.8697134336183));
#25013=CARTESIAN_POINT('Ctrl Pts',(-1.89558530704206,-2.32747338527323,
21.8705774378709));
#25014=CARTESIAN_POINT('Ctrl Pts',(-1.97361295219982,-2.26169267203088,
21.8713836157024));
#25015=CARTESIAN_POINT('Ctrl Pts',(-2.04813532502368,-2.19206334087092,
21.8721336268026));
#25016=CARTESIAN_POINT('Ctrl Pts',(-2.12254248874703,-2.1225416543324,21.8728824784107));
#25017=CARTESIAN_POINT('Ctrl Pts',(-2.1934549447046,-2.0491834436902,21.8735753368172));
#25018=CARTESIAN_POINT('Ctrl Pts',(-2.2604935455019,-1.97235111751034,21.8742138540263));
#25019=CARTESIAN_POINT('Ctrl Pts',(-2.28764065829647,-1.94123806025276,
21.8744724199643));
#25020=CARTESIAN_POINT('Ctrl Pts',(-2.31415291921105,-1.90955575635341,
21.8747220748988));
#25021=CARTESIAN_POINT('Ctrl Pts',(-2.34000681387336,-1.87733004850673,
21.8749629285299));
#25022=CARTESIAN_POINT('Ctrl Pts',(-2.39854704458456,-1.80436230431125,
21.8755082864853));
#25023=CARTESIAN_POINT('Ctrl Pts',(-2.45373755903258,-1.72857059033661,
21.8760085208243));
#25024=CARTESIAN_POINT('Ctrl Pts',(-2.50529548516313,-1.65030134582181,
21.8764659088202));
#25025=CARTESIAN_POINT('Ctrl Pts',(-2.55682438665815,-1.57207616313154,
21.8769230393287));
#25026=CARTESIAN_POINT('Ctrl Pts',(-2.60472450989376,-1.49137659468018,
21.8773373717214));
#25027=CARTESIAN_POINT('Ctrl Pts',(-2.64875480042251,-1.40858013873501,
21.8777111794279));
#25028=CARTESIAN_POINT('Ctrl Pts',(-2.6927693533044,-1.32581327653925,21.8780848535252));
#25029=CARTESIAN_POINT('Ctrl Pts',(-2.73291661193963,-1.24095141659554,
21.8784180319004));
#25030=CARTESIAN_POINT('Ctrl Pts',(-2.76900090393528,-1.15439767584903,
21.8787129855462));
#25031=CARTESIAN_POINT('Ctrl Pts',(-2.80509635843587,-1.06781716011249,
21.8790080304346));
#25032=CARTESIAN_POINT('Ctrl Pts',(-2.83712615654066,-0.979544134173076,
21.8792648269406));
#25033=CARTESIAN_POINT('Ctrl Pts',(-2.86494263903965,-0.890002064611414,
21.8794856481653));
#25034=CARTESIAN_POINT('Ctrl Pts',(-2.88763543272642,-0.816953298976749,
21.8796657949719));
#25035=CARTESIAN_POINT('Ctrl Pts',(-2.90752498795916,-0.743060415173017,
21.8798219989361));
#25036=CARTESIAN_POINT('Ctrl Pts',(-2.92455591077185,-0.668560187843599,
21.8799554942307));
#25037=CARTESIAN_POINT('Ctrl Pts',(-2.94760321776225,-0.567741833547698,
21.8801361483897));
#25038=CARTESIAN_POINT('Ctrl Pts',(-2.96542055692276,-0.465785336223467,
21.8802752157295));
#25039=CARTESIAN_POINT('Ctrl Pts',(-2.9779300558943,-0.363225249950262,
21.8803728029858));
#25040=CARTESIAN_POINT('Ctrl Pts',(-2.99045336542708,-0.260551936731979,
21.880470497979));
#25041=CARTESIAN_POINT('Ctrl Pts',(-2.99765709289031,-0.157274008900583,
21.8805266212497));
#25042=CARTESIAN_POINT('Ctrl Pts',(-2.99951519597997,-0.0539313367649988,
21.8805412798873));
#25043=CARTESIAN_POINT('Ctrl Pts',(-2.99983617653992,-0.0360792655033546,
21.8805438121137));
#25044=CARTESIAN_POINT('Ctrl Pts',(-2.99999776244028,-0.0182252642061044,
21.8805451069813));
#25045=CARTESIAN_POINT('Ctrl Pts',(-2.99999997692161,-0.000372116104727271,
21.880545165042));
#25046=CARTESIAN_POINT('',(-0.499999999999999,-2.95803989154981,24.3207730140306));
#25047=CARTESIAN_POINT('',(-0.499999999999999,-2.95803989154981,39.1419356690201));
#25048=CARTESIAN_POINT('Ctrl Pts',(-0.499999999999998,-2.95803989154981,
24.3207730140306));
#25049=CARTESIAN_POINT('Ctrl Pts',(-0.331796881873697,-2.98647140773842,
24.3173150006272));
#25050=CARTESIAN_POINT('Ctrl Pts',(-0.163503365753256,-3.,24.3156328315757));
#25051=CARTESIAN_POINT('Ctrl Pts',(0.163503365753248,-3.,24.3156328315757));
#25052=CARTESIAN_POINT('Ctrl Pts',(0.331796881873693,-2.98647140773842,
24.3173150006272));
#25053=CARTESIAN_POINT('Ctrl Pts',(0.5,-2.95803989154981,24.3207730140306));
#25054=CARTESIAN_POINT('',(-0.500000000000001,2.95803989154981,24.3207730140306));
#25055=CARTESIAN_POINT('Ctrl Pts',(0.499999999999998,2.95803989154981,24.3207730140306));
#25056=CARTESIAN_POINT('Ctrl Pts',(0.331796881873692,2.98647140773842,24.3173150006272));
#25057=CARTESIAN_POINT('Ctrl Pts',(0.163503365753246,3.,24.3156328315757));
#25058=CARTESIAN_POINT('Ctrl Pts',(-7.97972798949331E-15,3.,24.3156328315757));
#25059=CARTESIAN_POINT('Ctrl Pts',(-0.163503365753258,3.,24.3156328315757));
#25060=CARTESIAN_POINT('Ctrl Pts',(-0.331796881873699,2.98647140773842,
24.3173150006272));
#25061=CARTESIAN_POINT('Ctrl Pts',(-0.500000000000002,2.95803989154981,
24.3207730140306));
#25062=CARTESIAN_POINT('',(-0.500010187139659,2.95803816959088,21.8534623270851));
#25063=CARTESIAN_POINT('',(-0.500000000000001,2.95803989154981,39.1419356690201));
#25064=CARTESIAN_POINT('Ctrl Pts',(-2.9999999769217,-0.000372115392980615,
21.880545165042));
#25065=CARTESIAN_POINT('Ctrl Pts',(-3.00001277286105,0.102788942964087,
21.8805455005347));
#25066=CARTESIAN_POINT('Ctrl Pts',(-2.99470013233285,0.205905330647462,
21.8805045404221));
#25067=CARTESIAN_POINT('Ctrl Pts',(-2.98410189910898,0.308441008515781,
21.8804223912109));
#25068=CARTESIAN_POINT('Ctrl Pts',(-2.97349464501599,0.411063961395882,
21.8803401720769));
#25069=CARTESIAN_POINT('Ctrl Pts',(-2.95759284574052,0.513104906228459,
21.8802166936969));
#25070=CARTESIAN_POINT('Ctrl Pts',(-2.93648808754871,0.61403396623034,21.8800520628496));
#25071=CARTESIAN_POINT('Ctrl Pts',(-2.93249958683041,0.633108130674964,
21.8800209499486));
#25072=CARTESIAN_POINT('Ctrl Pts',(-2.92832540577109,0.65214261275552,21.8799883672603));
#25073=CARTESIAN_POINT('Ctrl Pts',(-2.92396636693129,0.671133880127263,
21.8799543155056));
#25074=CARTESIAN_POINT('Ctrl Pts',(-2.90131348256699,0.769826963514177,
21.8797773566643));
#25075=CARTESIAN_POINT('Ctrl Pts',(-2.87365814172373,0.867378355378354,
21.8795607237316));
#25076=CARTESIAN_POINT('Ctrl Pts',(-2.84113958094458,0.963289095541988,
21.879301307984));
#25077=CARTESIAN_POINT('Ctrl Pts',(-2.80862422134745,1.05919039409045,21.8790419177738));
#25078=CARTESIAN_POINT('Ctrl Pts',(-2.77124670666013,1.15345103353225,21.8787397531715));
#25079=CARTESIAN_POINT('Ctrl Pts',(-2.72919572627057,1.24558849051623,21.878391706372));
#25080=CARTESIAN_POINT('Ctrl Pts',(-2.68715425179392,1.33770511919527,21.8780437382508));
#25081=CARTESIAN_POINT('Ctrl Pts',(-2.6404415648864,1.42769920755386,21.8776499086739));
#25082=CARTESIAN_POINT('Ctrl Pts',(-2.58929383883054,1.51510970434297,21.8772071119431));
#25083=CARTESIAN_POINT('Ctrl Pts',(-2.5381556180301,1.60250395683029,21.8767643975013));
#25084=CARTESIAN_POINT('Ctrl Pts',(-2.48258417734381,1.68731527556145,21.8762727341039));
#25085=CARTESIAN_POINT('Ctrl Pts',(-2.42286082065673,1.76910865797627,21.875729017784));
#25086=CARTESIAN_POINT('Ctrl Pts',(-2.39643455500711,1.80530042233742,21.8754884353267));
#25087=CARTESIAN_POINT('Ctrl Pts',(-2.36919597786386,1.84090168069933,21.8752376615998));
#25088=CARTESIAN_POINT('Ctrl Pts',(-2.34117214558247,1.8758765910232,21.8749764277025));
#25089=CARTESIAN_POINT('Ctrl Pts',(-2.282548149704,1.94904178049793,21.8744299437397));
#25090=CARTESIAN_POINT('Ctrl Pts',(-2.22046648084456,2.01948669411621,21.8738376841246));
#25091=CARTESIAN_POINT('Ctrl Pts',(-2.15521897788651,2.08687114057333,21.8731985334558));
#25092=CARTESIAN_POINT('Ctrl Pts',(-2.08994940172927,2.15427838315662,21.8725591665625));
#25093=CARTESIAN_POINT('Ctrl Pts',(-2.0215121604408,2.21862275891459,21.8718728768836));
#25094=CARTESIAN_POINT('Ctrl Pts',(-1.95023698961227,2.27959989567207,21.8711385478849));
#25095=CARTESIAN_POINT('Ctrl Pts',(-1.87895152209695,2.34058584142251,21.8704041128022));
#25096=CARTESIAN_POINT('Ctrl Pts',(-1.80482766067384,2.39820329494175,21.8696216245189));
#25097=CARTESIAN_POINT('Ctrl Pts',(-1.72822787640916,2.45218849340794,21.8687899660169));
#25098=CARTESIAN_POINT('Ctrl Pts',(-1.65154355910333,2.5062332681908,21.8679573897236));
#25099=CARTESIAN_POINT('Ctrl Pts',(-1.57237823920555,2.55663753166712,21.8670755346263));
#25100=CARTESIAN_POINT('Ctrl Pts',(-1.49112266929207,2.60318135847722,21.8661432800049));
#25101=CARTESIAN_POINT('Ctrl Pts',(-1.42636912281268,2.64027269702651,21.8654003550212));
#25102=CARTESIAN_POINT('Ctrl Pts',(-1.36028872917732,2.67491323132945,21.8646254228678));
#25103=CARTESIAN_POINT('Ctrl Pts',(-1.29308896453722,2.70701328585437,21.8638179163547));
#25104=CARTESIAN_POINT('Ctrl Pts',(-1.20152769001504,2.75075037214142,21.862717669562));
#25105=CARTESIAN_POINT('Ctrl Pts',(-1.10785107791141,2.78978775972883,21.8615569494174));
#25106=CARTESIAN_POINT('Ctrl Pts',(-1.01255088571331,2.82395833960793,21.8603402470613));
#25107=CARTESIAN_POINT('Ctrl Pts',(-0.91698029339272,2.85822587342566,21.8591200924933));
#25108=CARTESIAN_POINT('Ctrl Pts',(-0.819777235734428,2.8875988784158,21.8578436375807));
#25109=CARTESIAN_POINT('Ctrl Pts',(-0.72144856800572,2.91196015833365,21.8565154118015));
#25110=CARTESIAN_POINT('Ctrl Pts',(-0.648189723848912,2.93011029959139,
21.8555258297436));
#25111=CARTESIAN_POINT('Ctrl Pts',(-0.574306323359667,2.94547956728581,
21.8545075104328));
#25112=CARTESIAN_POINT('Ctrl Pts',(-0.500010187139659,2.95803816959088,
21.8534623270851));
#25113=CARTESIAN_POINT('',(-3.00000000000001,-3.67394039744206E-16,50.1419356690201));
#25114=CARTESIAN_POINT('',(-3.00000000000001,3.67394039744206E-16,39.1419356690201));
#25115=CARTESIAN_POINT('Origin',(-1.041818884589E-14,0.,50.1419356690201));
#25116=CARTESIAN_POINT('Ctrl Pts',(-0.500000469469731,0.249901395376665,
19.1419331299742));
#25117=CARTESIAN_POINT('Ctrl Pts',(-0.499985448781684,0.249900114156667,
19.1419329138876));
#25118=CARTESIAN_POINT('Ctrl Pts',(-0.499957241892457,0.233340033373888,
19.1419289227389));
#25119=CARTESIAN_POINT('Ctrl Pts',(-0.499923116233831,0.161617725953644,
19.141926874418));
#25120=CARTESIAN_POINT('Ctrl Pts',(-0.499903664359004,0.0578516765404966,
19.1419267769168));
#25121=CARTESIAN_POINT('Ctrl Pts',(-0.499903654163716,-0.057515157620163,
19.141926775308));
#25122=CARTESIAN_POINT('Ctrl Pts',(-0.49992318239623,-0.161934834392146,
19.1419268788806));
#25123=CARTESIAN_POINT('Ctrl Pts',(-0.499957222592849,-0.233146393750517,
19.1419289247299));
#25124=CARTESIAN_POINT('Ctrl Pts',(-0.499985489109375,-0.249900109243623,
19.1419329215289));
#25125=CARTESIAN_POINT('Ctrl Pts',(-0.500000469469731,-0.249901395376665,
19.1419331299742));
#25126=CARTESIAN_POINT('Ctrl Pts',(-0.500005900053987,1.07273098952165,
19.1419037595993));
#25127=CARTESIAN_POINT('Ctrl Pts',(-0.617766856411166,1.05838431779768,
19.1642178069961));
#25128=CARTESIAN_POINT('Ctrl Pts',(-0.846046992725819,0.968758392758925,
19.1965193366959));
#25129=CARTESIAN_POINT('Ctrl Pts',(-1.12222824035265,0.664689422677935,
19.213096972248));
#25130=CARTESIAN_POINT('Ctrl Pts',(-1.27965361509687,0.238169805111735,
19.2138860499928));
#25131=CARTESIAN_POINT('Ctrl Pts',(-1.27973612410747,-0.237098012192637,
19.2138990693925));
#25132=CARTESIAN_POINT('Ctrl Pts',(-1.12169278387221,-0.666446671624522,
19.2130608557749));
#25133=CARTESIAN_POINT('Ctrl Pts',(-0.846203186258647,-0.968026539109895,
19.196503222222));
#25134=CARTESIAN_POINT('Ctrl Pts',(-0.61744048192897,-1.05842407959735,
19.1641559636152));
#25135=CARTESIAN_POINT('Ctrl Pts',(-0.500005900053987,-1.07273098952165,
19.1419037595993));
#25136=CARTESIAN_POINT('Ctrl Pts',(-0.374651529457775,2.49809898142235,
19.8198611757815));
#25137=CARTESIAN_POINT('Ctrl Pts',(-0.709304281794272,2.46080198574607,
19.8562158762544));
#25138=CARTESIAN_POINT('Ctrl Pts',(-1.35614981263617,2.24374050137417,19.9090264719253));
#25139=CARTESIAN_POINT('Ctrl Pts',(-2.13291772239582,1.53846891438119,19.9370353986983));
#25140=CARTESIAN_POINT('Ctrl Pts',(-2.57376446971679,0.551283320370357,
19.9395318251872));
#25141=CARTESIAN_POINT('Ctrl Pts',(-2.57408736573143,-0.547866663199184,
19.9396043925739));
#25142=CARTESIAN_POINT('Ctrl Pts',(-2.131400781918,-1.5414737450019,19.9369687673424));
#25143=CARTESIAN_POINT('Ctrl Pts',(-1.35656745347333,-2.24213214922828,
19.9089983547958));
#25144=CARTESIAN_POINT('Ctrl Pts',(-0.708376791714899,-2.46090535436693,
19.8561151192046));
#25145=CARTESIAN_POINT('Ctrl Pts',(-0.374651529457774,-2.49809898142235,
19.8198611757815));
#25146=CARTESIAN_POINT('Ctrl Pts',(-0.112199737628213,3.,21.2392862649499));
#25147=CARTESIAN_POINT('Ctrl Pts',(-0.545410746577865,2.98330036684518,
21.254809362827));
#25148=CARTESIAN_POINT('Ctrl Pts',(-1.40427372201026,2.76191164610531,21.2789029635529));
#25149=CARTESIAN_POINT('Ctrl Pts',(-2.44430047244797,1.90558668934363,21.2949283871888));
#25150=CARTESIAN_POINT('Ctrl Pts',(-3.02549086011703,0.682397094945288,
21.2989773348059));
#25151=CARTESIAN_POINT('Ctrl Pts',(-3.02590131894121,-0.678601175881948,
21.2990103838934));
#25152=CARTESIAN_POINT('Ctrl Pts',(-2.44234533102359,-1.90963444251436,
21.2948917804808));
#25153=CARTESIAN_POINT('Ctrl Pts',(-1.40492064000836,-2.75971763396258,
21.2788949026146));
#25154=CARTESIAN_POINT('Ctrl Pts',(-0.544210102297275,-2.98334664987728,
21.2547663405623));
#25155=CARTESIAN_POINT('Ctrl Pts',(-0.112199737628212,-3.,21.2392862649499));
#25156=CARTESIAN_POINT('Ctrl Pts',(-7.45975288878436E-15,3.,21.846099125618));
#25157=CARTESIAN_POINT('Ctrl Pts',(-0.443076107560811,3.,21.8529261923905));
#25158=CARTESIAN_POINT('Ctrl Pts',(-1.33511668480881,2.80117070574288,21.864996243952));
#25159=CARTESIAN_POINT('Ctrl Pts',(-2.42205080766271,1.94015854780963,21.8760313557109));
#25160=CARTESIAN_POINT('Ctrl Pts',(-3.02500193874651,0.694487451784985,
21.8807368994193));
#25161=CARTESIAN_POINT('Ctrl Pts',(-3.02547311532246,-0.690448134612415,
21.8807469396456));
#25162=CARTESIAN_POINT('Ctrl Pts',(-2.42004712161993,-1.94396598412946,
21.8760083073826));
#25163=CARTESIAN_POINT('Ctrl Pts',(-1.33584762052156,-2.79884623232731,
21.8649974020032));
#25164=CARTESIAN_POINT('Ctrl Pts',(-0.44184812216012,-3.,21.8529072711754));
#25165=CARTESIAN_POINT('Ctrl Pts',(-6.13614521966489E-15,-3.,21.846099125618));
#25166=CARTESIAN_POINT('',(-0.500000234886957,-0.25000317233103,19.141934398682));
#25167=CARTESIAN_POINT('Ctrl Pts',(-0.500000469773915,-0.250006344662061,
19.1419331283439));
#25168=CARTESIAN_POINT('Ctrl Pts',(-0.500000469773915,-0.267897236362903,
19.141933220399));
#25169=CARTESIAN_POINT('Ctrl Pts',(-0.5,-0.285781329331433,19.142122715467));
#25170=CARTESIAN_POINT('Ctrl Pts',(-0.5,-0.64758885702648,19.1497656467621));
#25171=CARTESIAN_POINT('Ctrl Pts',(-0.500000000107091,-0.988812928155548,
19.2265798854459));
#25172=CARTESIAN_POINT('Ctrl Pts',(-0.500000000107091,-1.62419910157496,
19.497759752549));
#25173=CARTESIAN_POINT('Ctrl Pts',(-0.500000000136194,-1.91845070856788,
19.6932873379294));
#25174=CARTESIAN_POINT('Ctrl Pts',(-0.500000000136194,-2.44455442803125,
20.2134309729014));
#25175=CARTESIAN_POINT('Ctrl Pts',(-0.499999999833597,-2.6227758687745,
20.5122259888824));
#25176=CARTESIAN_POINT('Ctrl Pts',(-0.499999999833597,-2.81084481109436,
20.956140074914));
#25177=CARTESIAN_POINT('Ctrl Pts',(-0.499999999999005,-2.86545145668325,
21.1318273751738));
#25178=CARTESIAN_POINT('Ctrl Pts',(-0.499999999999005,-2.93869500034237,
21.489376554184));
#25179=CARTESIAN_POINT('Ctrl Pts',(-0.499999999999999,-2.95754295724416,
21.6714024771996));
#25180=CARTESIAN_POINT('Ctrl Pts',(-0.499999999999999,-2.95745528673186,
21.8534537921611));
#25181=CARTESIAN_POINT('',(-0.500000234886961,0.250003167770442,19.141934398682));
#25182=CARTESIAN_POINT('Ctrl Pts',(-0.500000000000001,2.9579076296201,21.8534495050302));
#25183=CARTESIAN_POINT('Ctrl Pts',(-0.500000000000001,2.95794617404091,
21.6714260178936));
#25184=CARTESIAN_POINT('Ctrl Pts',(-0.499999999999072,2.93905792987264,
21.4894257571556));
#25185=CARTESIAN_POINT('Ctrl Pts',(-0.499999999999072,2.86575578974211,
21.131933596822));
#25186=CARTESIAN_POINT('Ctrl Pts',(-0.499999999845839,2.81112780850596,
20.9562698452876));
#25187=CARTESIAN_POINT('Ctrl Pts',(-0.499999999845839,2.62298756861714,
20.5123154976842));
#25188=CARTESIAN_POINT('Ctrl Pts',(-0.500000000065174,2.44468731250608,
20.2134475716897));
#25189=CARTESIAN_POINT('Ctrl Pts',(-0.500000000065174,1.91839767990519,
19.693207353235));
#25190=CARTESIAN_POINT('Ctrl Pts',(-0.500000000096103,1.6240521846631,19.4976513579156));
#25191=CARTESIAN_POINT('Ctrl Pts',(-0.500000000096103,0.988611016087444,
19.2265302537515));
#25192=CARTESIAN_POINT('Ctrl Pts',(-0.5,0.647449189595379,19.1497522054971));
#25193=CARTESIAN_POINT('Ctrl Pts',(-0.5,0.285729471252588,19.1421221660728));
#25194=CARTESIAN_POINT('Ctrl Pts',(-0.500000469773922,0.267871306763669,
19.141933220169));
#25195=CARTESIAN_POINT('Ctrl Pts',(-0.500000469773922,0.250006335540885,
19.1419331283438));
#25196=CARTESIAN_POINT('',(-0.5,-5.55111512312568E-17,19.1419356690201));
#25197=CARTESIAN_POINT('Origin',(-0.5,0.,0.));
#25198=CARTESIAN_POINT('Origin',(-0.5,0.,0.));
#25199=CARTESIAN_POINT('Origin',(-0.5,0.,0.));
#25200=CARTESIAN_POINT('Ctrl Pts',(-3.18327948107155,-0.464668609862618,
60.6133098318917));
#25201=CARTESIAN_POINT('Ctrl Pts',(-3.3370532982496,0.588781153171032,60.5474729574974));
#25202=CARTESIAN_POINT('Ctrl Pts',(-2.51393860486939,2.84257920150003,60.4157992087088));
#25203=CARTESIAN_POINT('Ctrl Pts',(1.01311494220538,3.66090406549081,60.2182885855259));
#25204=CARTESIAN_POINT('Ctrl Pts',(3.61694504820724,1.15041235324949,60.0207779623431));
#25205=CARTESIAN_POINT('Ctrl Pts',(2.94104075517665,-2.40027689070238,59.8232673391602));
#25206=CARTESIAN_POINT('Ctrl Pts',(-0.404228016077643,-3.77497842620744,
59.6257567159773));
#25207=CARTESIAN_POINT('Ctrl Pts',(-3.38226164936567,-1.7237444337863,59.4282460927945));
#25208=CARTESIAN_POINT('Ctrl Pts',(-3.29180676033138,1.89099555051049,59.2307354696115));
#25209=CARTESIAN_POINT('Ctrl Pts',(-0.214572769937683,3.79025880578182,
59.0332248464286));
#25210=CARTESIAN_POINT('Ctrl Pts',(3.05728290832011,2.25050459215375,58.8357142232458));
#25211=CARTESIAN_POINT('Ctrl Pts',(3.55529376345934,-1.33107756875446,58.6382036000628));
#25212=CARTESIAN_POINT('Ctrl Pts',(0.827568737366059,-3.70500041251386,
58.4406929768801));
#25213=CARTESIAN_POINT('Ctrl Pts',(-2.65100241828356,-2.71735937131622,
58.2431823536971));
#25214=CARTESIAN_POINT('Ctrl Pts',(-3.72432089987947,0.735736741130725,
58.0456717305143));
#25215=CARTESIAN_POINT('Ctrl Pts',(-1.4185583128274,3.52130193062268,57.8481611073313));
#25216=CARTESIAN_POINT('Ctrl Pts',(2.1742623397949,3.11198543505612,57.6506504841485));
#25217=CARTESIAN_POINT('Ctrl Pts',(3.79437361613089,-0.12083688877652,57.4531398609656));
#25218=CARTESIAN_POINT('Ctrl Pts',(1.97184661356077,-3.24402426334415,57.2556292377827));
#25219=CARTESIAN_POINT('Ctrl Pts',(-1.63973818462279,-3.42390575612951,
57.0581186145998));
#25220=CARTESIAN_POINT('Ctrl Pts',(-3.76358735442354,-0.497275092791353,
56.860607991417));
#25221=CARTESIAN_POINT('Ctrl Pts',(-2.47273085453206,2.88053369334928,56.6630973682341));
#25222=CARTESIAN_POINT('Ctrl Pts',(1.06163619548771,3.64483206301732,56.4655867450512));
#25223=CARTESIAN_POINT('Ctrl Pts',(3.63277993397126,1.10217157297284,56.2680761218683));
#25224=CARTESIAN_POINT('Ctrl Pts',(2.90789970035265,-2.44049002193061,56.0705654986855));
#25225=CARTESIAN_POINT('Ctrl Pts',(-0.45532011802947,-3.76889317954298,
55.8730548755026));
#25226=CARTESIAN_POINT('Ctrl Pts',(-3.40542765166225,-1.677776720555,55.6755442523197));
#25227=CARTESIAN_POINT('Ctrl Pts',(-3.26578811328327,1.93558782065046,55.4780336291368));
#25228=CARTESIAN_POINT('Ctrl Pts',(-0.16309656227425,3.79279207493464,55.2805230059539));
#25229=CARTESIAN_POINT('Ctrl Pts',(3.08757262307394,2.20879322526724,55.0830123827711));
#25230=CARTESIAN_POINT('Ctrl Pts',(3.53688484260436,-1.37924538021458,54.8855017595881));
#25231=CARTESIAN_POINT('Ctrl Pts',(0.777178784528909,-3.71589361410309,
54.6879911364054));
#25232=CARTESIAN_POINT('Ctrl Pts',(-2.68766217377324,-2.68110877522757,
54.4904805132223));
#25233=CARTESIAN_POINT('Ctrl Pts',(-3.71398521084471,0.786248073317566,
54.2929698900396));
#25234=CARTESIAN_POINT('Ctrl Pts',(-1.37060668705354,3.54024145318923,54.0954592668566));
#25235=CARTESIAN_POINT('Ctrl Pts',(2.21632434779813,3.08217109804834,53.8979486436738));
#25236=CARTESIAN_POINT('Ctrl Pts',(3.79238256933727,-0.17235541405342,53.7004380204909));
#25237=CARTESIAN_POINT('Ctrl Pts',(1.92760936000513,-3.27050372936606,53.502927397308));
#25238=CARTESIAN_POINT('Ctrl Pts',(-1.68608552885002,-3.40132154932197,
53.3054167741251));
#25239=CARTESIAN_POINT('Ctrl Pts',(-3.76999323703601,-0.446117768032975,
53.1079061509423));
#25240=CARTESIAN_POINT('Ctrl Pts',(-2.43338426356776,2.91384900077535,52.9103955277594));
#25241=CARTESIAN_POINT('Ctrl Pts',(1.11103811731961,3.63007837648053,52.7128849045765));
#25242=CARTESIAN_POINT('Ctrl Pts',(3.64741072255014,1.05273491233617,52.5153742813936));
#25243=CARTESIAN_POINT('Ctrl Pts',(2.87449292200031,-2.47975573659254,52.3178636582107));
#25244=CARTESIAN_POINT('Ctrl Pts',(-0.506470599677197,-3.76236212640368,
52.1203530350279));
#25245=CARTESIAN_POINT('Ctrl Pts',(-3.42788079845058,-1.63137455307642,
51.9228424118449));
#25246=CARTESIAN_POINT('Ctrl Pts',(-3.23923631769043,1.97976043160802,51.7253317886621));
#25247=CARTESIAN_POINT('Ctrl Pts',(-0.111502357959493,3.79465718393418,
51.5278211654792));
#25248=CARTESIAN_POINT('Ctrl Pts',(3.1171426479274,2.16665882183862,51.3303105422963));
#25249=CARTESIAN_POINT('Ctrl Pts',(3.51811058329886,-1.427151124091,51.1327999191135));
#25250=CARTESIAN_POINT('Ctrl Pts',(0.726079346912793,-3.72610502504112,
50.9352892959306));
#25251=CARTESIAN_POINT('Ctrl Pts',(-2.72269906505329,-2.64436190137017,
50.7377786727477));
#25252=CARTESIAN_POINT('Ctrl Pts',(-3.70522749830404,0.83660602953753,50.5402680495648));
#25253=CARTESIAN_POINT('Ctrl Pts',(-1.31715611094438,3.55923486122354,50.3427135111009));
#25254=CARTESIAN_POINT('Ctrl Pts',(1.05918636994692,3.21910041479783,50.2109958470314));
#25255=CARTESIAN_POINT('Ctrl Pts',(1.9151416701175,2.58484374727087,50.1451150573561));
#25256=CARTESIAN_POINT('Ctrl Pts',(-3.42030586252901,-0.49926774569958,
60.4750123196129));
#25257=CARTESIAN_POINT('Ctrl Pts',(-3.58552964872969,0.632621685250075,
60.4091754452186));
#25258=CARTESIAN_POINT('Ctrl Pts',(-2.70112599267545,3.05423710528894,60.2775016964301));
#25259=CARTESIAN_POINT('Ctrl Pts',(1.08855128707529,3.9334942821733,60.0799910732471));
#25260=CARTESIAN_POINT('Ctrl Pts',(3.88626208486859,1.2360718370919,59.8824804500643));
#25261=CARTESIAN_POINT('Ctrl Pts',(3.16003008742461,-2.57900104900582,59.6849698268814));
#25262=CARTESIAN_POINT('Ctrl Pts',(-0.434326756858761,-4.05606259797573,
59.4874592036985));
#25263=CARTESIAN_POINT('Ctrl Pts',(-3.63410420502517,-1.85209411471355,
59.2899485805156));
#25264=CARTESIAN_POINT('Ctrl Pts',(-3.53691406225007,2.03179871760746,59.0924379573328));
#25265=CARTESIAN_POINT('Ctrl Pts',(-0.230549817356877,4.07248075169131,
58.8949273341499));
#25266=CARTESIAN_POINT('Ctrl Pts',(3.28492760906342,2.41807673374656,58.697416710967));
#25267=CARTESIAN_POINT('Ctrl Pts',(3.82002025724725,-1.43018934999676,58.4999060877841));
#25268=CARTESIAN_POINT('Ctrl Pts',(0.889189347303573,-3.98087403476363,
58.3023954646013));
#25269=CARTESIAN_POINT('Ctrl Pts',(-2.84839555142724,-2.91969343049402,
58.1048848414183));
#25270=CARTESIAN_POINT('Ctrl Pts',(-4.00163312192405,0.790519558188566,
57.9073742182355));
#25271=CARTESIAN_POINT('Ctrl Pts',(-1.52418389354541,3.78349739903745,57.7098635950526));
#25272=CARTESIAN_POINT('Ctrl Pts',(2.33615749785601,3.34370327548005,57.5123529718697));
#25273=CARTESIAN_POINT('Ctrl Pts',(4.07690195003213,-0.129834380408526,
57.3148423486869));
#25274=CARTESIAN_POINT('Ctrl Pts',(2.11866993535222,-3.48557368967409,57.117331725504));
#25275=CARTESIAN_POINT('Ctrl Pts',(-1.76183277630091,-3.6788491240155,56.9198211023211));
#25276=CARTESIAN_POINT('Ctrl Pts',(-4.04382334916498,-0.534302101112215,
56.7223104791382));
#25277=CARTESIAN_POINT('Ctrl Pts',(-2.6568499211277,3.09501768134366,56.5247998559553));
#25278=CARTESIAN_POINT('Ctrl Pts',(1.14068542359885,3.9162255614689,56.3272892327724));
#25279=CARTESIAN_POINT('Ctrl Pts',(3.90327603319866,1.1842390575404,56.1297786095896));
#25280=CARTESIAN_POINT('Ctrl Pts',(3.1244213559956,-2.62220844229581,55.9322679864067));
#25281=CARTESIAN_POINT('Ctrl Pts',(-0.489223166952141,-4.04952424500823,
55.7347573632238));
#25282=CARTESIAN_POINT('Ctrl Pts',(-3.65899514342298,-1.80270365434495,
55.5372467400409));
#25283=CARTESIAN_POINT('Ctrl Pts',(-3.50895807171802,2.07971131965516,55.3397361168581));
#25284=CARTESIAN_POINT('Ctrl Pts',(-0.175240701114049,4.07520264758084,
55.1422254936751));
#25285=CARTESIAN_POINT('Ctrl Pts',(3.31747269018585,2.37325954645769,54.9447148704923));
#25286=CARTESIAN_POINT('Ctrl Pts',(3.80024061166555,-1.4819437274876,54.7472042473094));
#25287=CARTESIAN_POINT('Ctrl Pts',(0.835047368213682,-3.99257834206022,
54.5496936241266));
#25288=CARTESIAN_POINT('Ctrl Pts',(-2.88778498530066,-2.88074362195241,
54.3521830009436));
#25289=CARTESIAN_POINT('Ctrl Pts',(-3.99052783946013,0.844791954511317,
54.1546723777608));
#25290=CARTESIAN_POINT('Ctrl Pts',(-1.47266179888568,3.80384715483272,53.9571617545778));
#25291=CARTESIAN_POINT('Ctrl Pts',(2.38135143493212,3.31166896863973,53.7596511313951));
#25292=CARTESIAN_POINT('Ctrl Pts',(4.074762650275,-0.185188965226226,53.5621405082121));
#25293=CARTESIAN_POINT('Ctrl Pts',(2.07113878435583,-3.51402481167261,53.3646298850293));
#25294=CARTESIAN_POINT('Ctrl Pts',(-1.81163113491682,-3.65458330148761,
53.1671192618463));
#25295=CARTESIAN_POINT('Ctrl Pts',(-4.05070621257184,-0.479335611734573,
52.9696086386635));
#25296=CARTESIAN_POINT('Ctrl Pts',(-2.61457359052401,3.13081364019015,52.7720980154806));
#25297=CARTESIAN_POINT('Ctrl Pts',(1.19376580308377,3.90037331825376,52.5745873922978));
#25298=CARTESIAN_POINT('Ctrl Pts',(3.91899622749745,1.13112135260593,52.3770767691148));
#25299=CARTESIAN_POINT('Ctrl Pts',(3.08852711531516,-2.66439787456312,52.179566145932));
#25300=CARTESIAN_POINT('Ctrl Pts',(-0.544182303682422,-4.04250689090106,
51.9820555227491));
#25301=CARTESIAN_POINT('Ctrl Pts',(-3.68312014722769,-1.75284639034888,
51.7845448995661));
#25302=CARTESIAN_POINT('Ctrl Pts',(-3.48042923450254,2.12717301477798,51.5870342763833));
#25303=CARTESIAN_POINT('Ctrl Pts',(-0.119804802211798,4.07720663223984,
51.3895236532005));
#25304=CARTESIAN_POINT('Ctrl Pts',(3.34924449343556,2.32798782340666,51.1920130300175));
#25305=CARTESIAN_POINT('Ctrl Pts',(3.78006842460215,-1.53341652389258,50.9945024068347));
#25306=CARTESIAN_POINT('Ctrl Pts',(0.780143076243845,-4.00355009270407,
50.7969917836518));
#25307=CARTESIAN_POINT('Ctrl Pts',(-2.92543071680569,-2.84126058289429,
50.5994811604689));
#25308=CARTESIAN_POINT('Ctrl Pts',(-3.98111802931833,0.89889955452203,50.401970537286));
#25309=CARTESIAN_POINT('Ctrl Pts',(-1.41523130310019,3.82425480839735,50.2044159988222));
#25310=CARTESIAN_POINT('Ctrl Pts',(1.13805318451675,3.45879401613092,50.0726983347526));
#25311=CARTESIAN_POINT('Ctrl Pts',(2.05774275266322,2.77731071842175,50.0068175450773));
#25312=CARTESIAN_POINT('Ctrl Pts',(-3.65733224398648,-0.533866881536543,
60.3367148073341));
#25313=CARTESIAN_POINT('Ctrl Pts',(-3.83400599920978,0.67646221732912,60.2708779329399));
#25314=CARTESIAN_POINT('Ctrl Pts',(-2.8883133804815,3.26589500907783,60.1392041841513));
#25315=CARTESIAN_POINT('Ctrl Pts',(1.1639876319452,4.20608449885579,59.9416935609684));
#25316=CARTESIAN_POINT('Ctrl Pts',(4.15557912152994,1.3217313209343,59.7441829377855));
#25317=CARTESIAN_POINT('Ctrl Pts',(3.37901941967257,-2.75772520730928,59.5466723146026));
#25318=CARTESIAN_POINT('Ctrl Pts',(-0.46442549763987,-4.33714676974401,
59.3491616914197));
#25319=CARTESIAN_POINT('Ctrl Pts',(-3.88594676068467,-1.98044379564081,
59.1516510682369));
#25320=CARTESIAN_POINT('Ctrl Pts',(-3.78202136416876,2.17260188470443,58.954140445054));
#25321=CARTESIAN_POINT('Ctrl Pts',(-0.246526864776077,4.3547026976008,58.7566298218711));
#25322=CARTESIAN_POINT('Ctrl Pts',(3.51257230980675,2.58564887533937,58.5591191986882));
#25323=CARTESIAN_POINT('Ctrl Pts',(4.08474675103516,-1.52930113123906,58.3616085755053));
#25324=CARTESIAN_POINT('Ctrl Pts',(0.950809957241094,-4.25674765701341,
58.1640979523225));
#25325=CARTESIAN_POINT('Ctrl Pts',(-3.04578868457094,-3.12202748967183,
57.9665873291396));
#25326=CARTESIAN_POINT('Ctrl Pts',(-4.27894534396861,0.845302375246406,
57.7690767059567));
#25327=CARTESIAN_POINT('Ctrl Pts',(-1.62980947426342,4.04569286745222,57.5715660827738));
#25328=CARTESIAN_POINT('Ctrl Pts',(2.49805265591715,3.57542111590398,57.3740554595909));
#25329=CARTESIAN_POINT('Ctrl Pts',(4.35943028393339,-0.138831872040531,
57.1765448364081));
#25330=CARTESIAN_POINT('Ctrl Pts',(2.26549325714367,-3.72712311600402,56.9790342132252));
#25331=CARTESIAN_POINT('Ctrl Pts',(-1.88392736797904,-3.9337924919015,56.7815235900423));
#25332=CARTESIAN_POINT('Ctrl Pts',(-4.32405934390643,-0.571329109433077,
56.5840129668594));
#25333=CARTESIAN_POINT('Ctrl Pts',(-2.84096898772335,3.30950166933803,56.3865023436765));
#25334=CARTESIAN_POINT('Ctrl Pts',(1.21973465170998,4.18761905992049,56.1889917204937));
#25335=CARTESIAN_POINT('Ctrl Pts',(4.17377213242608,1.26630654210795,55.9914810973108));
#25336=CARTESIAN_POINT('Ctrl Pts',(3.34094301163854,-2.80392686266102,55.7939704741279));
#25337=CARTESIAN_POINT('Ctrl Pts',(-0.52312621587481,-4.33015531047348,
55.596459850945));
#25338=CARTESIAN_POINT('Ctrl Pts',(-3.91256263518371,-1.92763058813491,
55.3989492277621));
#25339=CARTESIAN_POINT('Ctrl Pts',(-3.75212803015276,2.22383481865987,55.2014386045793));
#25340=CARTESIAN_POINT('Ctrl Pts',(-0.187384839953852,4.35761322022704,
55.0039279813963));
#25341=CARTESIAN_POINT('Ctrl Pts',(3.54737275729779,2.53772586764813,54.8064173582136));
#25342=CARTESIAN_POINT('Ctrl Pts',(4.06359638072673,-1.58464207476064,54.6089067350305));
#25343=CARTESIAN_POINT('Ctrl Pts',(0.892915951898455,-4.26926307001734,
54.4113961118479));
#25344=CARTESIAN_POINT('Ctrl Pts',(-3.08790779682808,-3.08037846867725,
54.2138854886648));
#25345=CARTESIAN_POINT('Ctrl Pts',(-4.26707046807556,0.903335835705069,
54.0163748654821));
#25346=CARTESIAN_POINT('Ctrl Pts',(-1.57471691071782,4.0674528564762,53.8188642422991));
#25347=CARTESIAN_POINT('Ctrl Pts',(2.54637852206613,3.54116683923112,53.6213536191163));
#25348=CARTESIAN_POINT('Ctrl Pts',(4.35714273121273,-0.198022516399034,
53.4238429959333));
#25349=CARTESIAN_POINT('Ctrl Pts',(2.21466820870652,-3.75754589397916,53.2263323727505));
#25350=CARTESIAN_POINT('Ctrl Pts',(-1.93717674098361,-3.90784505365324,
53.0288217495676));
#25351=CARTESIAN_POINT('Ctrl Pts',(-4.33141918810767,-0.51255345543617,
52.8313111263847));
#25352=CARTESIAN_POINT('Ctrl Pts',(-2.79576291748028,3.34777827960495,52.6338005032018));
#25353=CARTESIAN_POINT('Ctrl Pts',(1.27649348884792,4.170668260027,52.436289880019));
#25354=CARTESIAN_POINT('Ctrl Pts',(4.19058173244477,1.2095077928757,52.238779256836));
#25355=CARTESIAN_POINT('Ctrl Pts',(3.30256130863,-2.8490400125337,52.0412686336532));
#25356=CARTESIAN_POINT('Ctrl Pts',(-0.581894007687646,-4.32265165539842,
51.8437580104704));
#25357=CARTESIAN_POINT('Ctrl Pts',(-3.93835949600481,-1.87431822762135,
51.6462473872874));
#25358=CARTESIAN_POINT('Ctrl Pts',(-3.72162215131465,2.27458559794796,51.4487367641046));
#25359=CARTESIAN_POINT('Ctrl Pts',(-0.128107246464106,4.3597560805455,51.2512261409216));
#25360=CARTESIAN_POINT('Ctrl Pts',(3.58134633894373,2.4893168249747,51.0537155177388));
#25361=CARTESIAN_POINT('Ctrl Pts',(4.04202626590543,-1.63968192369417,50.8562048945559));
#25362=CARTESIAN_POINT('Ctrl Pts',(0.834206805574899,-4.28099516036702,
50.658694271373));
#25363=CARTESIAN_POINT('Ctrl Pts',(-3.12816236855811,-3.03815926441841,
50.4611836481901));
#25364=CARTESIAN_POINT('Ctrl Pts',(-4.25700856033262,0.961193079506533,
50.2636730250073));
#25365=CARTESIAN_POINT('Ctrl Pts',(-1.513306495256,4.08927475557118,50.0661184865434));
#25366=CARTESIAN_POINT('Ctrl Pts',(1.21691999908657,3.69848761746401,49.9344008224738));
#25367=CARTESIAN_POINT('Ctrl Pts',(2.20034383520893,2.96977768957263,49.8685200327985));
#25368=CARTESIAN_POINT('Ctrl Pts',(-3.89435862544394,-0.568466017373507,
60.1984172950554));
#25369=CARTESIAN_POINT('Ctrl Pts',(-4.08248234968987,0.720302749408164,
60.1325804206611));
#25370=CARTESIAN_POINT('Ctrl Pts',(-3.07550076828757,3.47755291286672,60.0009066718726));
#25371=CARTESIAN_POINT('Ctrl Pts',(1.23942397681511,4.47867471553828,59.8033960486895));
#25372=CARTESIAN_POINT('Ctrl Pts',(4.42489615819129,1.4073908047767,59.6058854255068));
#25373=CARTESIAN_POINT('Ctrl Pts',(3.59800875192051,-2.93644936561273,59.4083748023238));
#25374=CARTESIAN_POINT('Ctrl Pts',(-0.494524238420983,-4.61823094151229,
59.2108641791409));
#25375=CARTESIAN_POINT('Ctrl Pts',(-4.13778931634418,-2.10879347656808,
59.0133535559581));
#25376=CARTESIAN_POINT('Ctrl Pts',(-4.02712866608745,2.3134050518014,58.8158429327752));
#25377=CARTESIAN_POINT('Ctrl Pts',(-0.262503912195272,4.63692464351029,
58.6183323095923));
#25378=CARTESIAN_POINT('Ctrl Pts',(3.74021701055006,2.75322101693219,58.4208216864095));
#25379=CARTESIAN_POINT('Ctrl Pts',(4.34947324482307,-1.62841291248137,58.2233110632265));
#25380=CARTESIAN_POINT('Ctrl Pts',(1.01243056717861,-4.53262127926318,58.0258004400437));
#25381=CARTESIAN_POINT('Ctrl Pts',(-3.24318181771463,-3.32436154884964,
57.8282898168608));
#25382=CARTESIAN_POINT('Ctrl Pts',(-4.55625756601319,0.900085192304248,
57.6307791936779));
#25383=CARTESIAN_POINT('Ctrl Pts',(-1.73543505498141,4.307888335867,57.4332685704951));
#25384=CARTESIAN_POINT('Ctrl Pts',(2.65994781397828,3.80713895632791,57.2357579473121));
#25385=CARTESIAN_POINT('Ctrl Pts',(4.64195861783464,-0.147829363672537,
57.0382473241294));
#25386=CARTESIAN_POINT('Ctrl Pts',(2.41231657893511,-3.96867254233396,56.8407367009463));
#25387=CARTESIAN_POINT('Ctrl Pts',(-2.00602195965716,-4.18873585978749,
56.6432260777636));
#25388=CARTESIAN_POINT('Ctrl Pts',(-4.60429533864786,-0.608356117753937,
56.4457154545806));
#25389=CARTESIAN_POINT('Ctrl Pts',(-3.025088054319,3.52398565733241,56.2482048313978));
#25390=CARTESIAN_POINT('Ctrl Pts',(1.29878387982112,4.45901255837208,56.0506942082149));
#25391=CARTESIAN_POINT('Ctrl Pts',(4.44426823165348,1.3483740266755,55.853183585032));
#25392=CARTESIAN_POINT('Ctrl Pts',(3.55746466728151,-2.98564528302621,55.6556729618491));
#25393=CARTESIAN_POINT('Ctrl Pts',(-0.557029264797485,-4.61078637593874,
55.4581623386663));
#25394=CARTESIAN_POINT('Ctrl Pts',(-4.16613012694443,-2.05255752192486,
55.2606517154833));
#25395=CARTESIAN_POINT('Ctrl Pts',(-3.9952979885875,2.36795831766459,55.0631410923005));
#25396=CARTESIAN_POINT('Ctrl Pts',(-0.199528978793653,4.64002379287325,
54.8656304691176));
#25397=CARTESIAN_POINT('Ctrl Pts',(3.77727282440971,2.70219218883858,54.6681198459347));
#25398=CARTESIAN_POINT('Ctrl Pts',(4.32695214978791,-1.68734042203366,54.4706092227519));
#25399=CARTESIAN_POINT('Ctrl Pts',(0.950784535583229,-4.54594779797445,
54.273098599569));
#25400=CARTESIAN_POINT('Ctrl Pts',(-3.2880306083555,-3.2800133154021,54.0755879763861));
#25401=CARTESIAN_POINT('Ctrl Pts',(-4.54361309669097,0.961879716898822,
53.8780773532032));
#25402=CARTESIAN_POINT('Ctrl Pts',(-1.67677202254996,4.33105855811969,53.6805667300203));
#25403=CARTESIAN_POINT('Ctrl Pts',(2.71140560920012,3.77066470982251,53.4830561068375));
#25404=CARTESIAN_POINT('Ctrl Pts',(4.63952281215046,-0.210856067571843,
53.2855454836546));
#25405=CARTESIAN_POINT('Ctrl Pts',(2.35819763305721,-4.00106697628572,53.0880348604717));
#25406=CARTESIAN_POINT('Ctrl Pts',(-2.06272234705041,-4.16110680581888,
52.8905242372888));
#25407=CARTESIAN_POINT('Ctrl Pts',(-4.61213216364352,-0.545771299137771,
52.693013614106));
#25408=CARTESIAN_POINT('Ctrl Pts',(-2.97695224443653,3.56474291901975,52.495502990923));
#25409=CARTESIAN_POINT('Ctrl Pts',(1.35922117461208,4.44096320180024,52.2979923677402));
#25410=CARTESIAN_POINT('Ctrl Pts',(4.46216723739208,1.28789423314547,52.1004817445573));
#25411=CARTESIAN_POINT('Ctrl Pts',(3.51659550194484,-3.03368215050428,51.9029711213744));
#25412=CARTESIAN_POINT('Ctrl Pts',(-0.619605711692866,-4.60279641989579,
51.7054604981916));
#25413=CARTESIAN_POINT('Ctrl Pts',(-4.19359884478193,-1.9957900648938,51.5079498750086));
#25414=CARTESIAN_POINT('Ctrl Pts',(-3.96281506812675,2.42199818111792,51.3104392518258));
#25415=CARTESIAN_POINT('Ctrl Pts',(-0.136409690716418,4.64230552885116,
51.1129286286429));
#25416=CARTESIAN_POINT('Ctrl Pts',(3.8134481844519,2.65064582654275,50.91541800546));
#25417=CARTESIAN_POINT('Ctrl Pts',(4.30398410720872,-1.74594732349575,50.7179073822772));
#25418=CARTESIAN_POINT('Ctrl Pts',(0.888270534905953,-4.55844022802997,
50.5203967590942));
#25419=CARTESIAN_POINT('Ctrl Pts',(-3.33089402031053,-3.23505794594252,
50.3228861359114));
#25420=CARTESIAN_POINT('Ctrl Pts',(-4.5328990913469,1.02348660449103,50.1253755127285));
#25421=CARTESIAN_POINT('Ctrl Pts',(-1.61138168741181,4.35429470274499,49.9278209742646));
#25422=CARTESIAN_POINT('Ctrl Pts',(1.29578681365639,3.9381812187971,49.7961033101951));
#25423=CARTESIAN_POINT('Ctrl Pts',(2.34294491775465,3.1622446607235,49.7302225205197));
#25424=CARTESIAN_POINT('Ctrl Pts',(-3.89612849629295,0.579535085171301,
50.1419356690201));
#25425=CARTESIAN_POINT('Ctrl Pts',(-3.87378467426801,0.674953501696104,
50.1419356690201));
#25426=CARTESIAN_POINT('Ctrl Pts',(-3.84767496861433,0.769312903700949,
50.1419356690201));
#25427=CARTESIAN_POINT('Ctrl Pts',(-3.81772557524066,0.862409043007997,
50.1419356690201));
#25428=CARTESIAN_POINT('Ctrl Pts',(-3.78035729159179,0.978566418779723,
50.1419356690201));
#25429=CARTESIAN_POINT('Ctrl Pts',(-3.73701237818807,1.09275838157917,50.1419356690201));
#25430=CARTESIAN_POINT('Ctrl Pts',(-3.68803000615501,1.20468203541671,50.1419356690201));
#25431=CARTESIAN_POINT('Ctrl Pts',(-3.63914263045098,1.31638862471031,50.1419356690201));
#25432=CARTESIAN_POINT('Ctrl Pts',(-3.5846388856755,1.42583629348278,50.1419356690201));
#25433=CARTESIAN_POINT('Ctrl Pts',(-3.52481692824774,1.53268991237077,50.1419356690201));
#25434=CARTESIAN_POINT('Ctrl Pts',(-3.51432549294881,1.55142965070804,50.1419356690201));
#25435=CARTESIAN_POINT('Ctrl Pts',(-3.50367040283234,1.57008950539708,50.1419356690201));
#25436=CARTESIAN_POINT('Ctrl Pts',(-3.49285316887854,1.58866753931983,50.1419356690201));
#25437=CARTESIAN_POINT('Ctrl Pts',(-3.48296828602639,1.60564430895741,50.1419356690201));
#25438=CARTESIAN_POINT('Ctrl Pts',(-3.47295262127336,1.62254480368252,50.1419356690201));
#25439=CARTESIAN_POINT('Ctrl Pts',(-3.46280887008029,1.63936581395016,50.1419356690201));
#25440=CARTESIAN_POINT('Ctrl Pts',(-3.40044038534557,1.74278918289247,50.1419356690201));
#25441=CARTESIAN_POINT('Ctrl Pts',(-3.33321848428269,1.84323554294225,50.1419356690201));
#25442=CARTESIAN_POINT('Ctrl Pts',(-3.26147120928829,1.94041070411502,50.1419356690201));
#25443=CARTESIAN_POINT('Ctrl Pts',(-3.18993639848207,2.03729810186083,50.1419356690201));
#25444=CARTESIAN_POINT('Ctrl Pts',(-3.11390221728981,2.13093420721513,50.1419356690201));
#25445=CARTESIAN_POINT('Ctrl Pts',(-3.03366045198661,2.22098857179085,50.1419356690201));
#25446=CARTESIAN_POINT('Ctrl Pts',(-2.97045908890593,2.29191869865241,50.1419356690201));
#25447=CARTESIAN_POINT('Ctrl Pts',(-2.90464668830478,2.36062614854751,50.1419356690201));
#25448=CARTESIAN_POINT('Ctrl Pts',(-2.83635575923465,2.42692897605195,50.1419356690201));
#25449=CARTESIAN_POINT('Ctrl Pts',(-2.82453123970119,2.43840925739568,50.1419356690201));
#25450=CARTESIAN_POINT('Ctrl Pts',(-2.81263489701748,2.44981492176028,50.1419356690201));
#25451=CARTESIAN_POINT('Ctrl Pts',(-2.80067361886952,2.46113940299019,50.1419356690201));
#25452=CARTESIAN_POINT('Ctrl Pts',(-2.71480504293152,2.54243649051047,50.1419356690201));
#25453=CARTESIAN_POINT('Ctrl Pts',(-2.62550045622586,2.61964271914596,50.1419356690201));
#25454=CARTESIAN_POINT('Ctrl Pts',(-2.53305872915569,2.69247759565464,50.1419356690201));
#25455=CARTESIAN_POINT('Ctrl Pts',(-2.44149007077266,2.7646245809693,50.1419356690201));
#25456=CARTESIAN_POINT('Ctrl Pts',(-2.34684250503465,2.8324828433291,50.1419356690201));
#25457=CARTESIAN_POINT('Ctrl Pts',(-2.24938224755213,2.8957353593087,50.1419356690201));
#25458=CARTESIAN_POINT('Ctrl Pts',(-2.15449925673441,2.95731520783275,50.1419356690201));
#25459=CARTESIAN_POINT('Ctrl Pts',(-2.05694969435008,3.01452992641812,50.1419356690201));
#25460=CARTESIAN_POINT('Ctrl Pts',(-1.95696652726181,3.06703984578374,50.1419356690201));
#25461=CARTESIAN_POINT('Ctrl Pts',(-1.89667591165149,3.09870372937933,50.1419356690201));
#25462=CARTESIAN_POINT('Ctrl Pts',(-1.83550019348387,3.12865593444139,50.1419356690201));
#25463=CARTESIAN_POINT('Ctrl Pts',(-1.77348962752687,3.15681277973307,50.1419356690201));
#25464=CARTESIAN_POINT('Ctrl Pts',(-1.74929795611695,3.16779737790153,50.1419356690201));
#25465=CARTESIAN_POINT('Ctrl Pts',(-1.72497922357456,3.17850865291385,50.1419356690201));
#25466=CARTESIAN_POINT('Ctrl Pts',(-1.70053641711253,3.18894132850405,50.1419356690201));
#25467=CARTESIAN_POINT('Ctrl Pts',(-1.68181840755981,3.19693054699503,50.1419356690201));
#25468=CARTESIAN_POINT('Ctrl Pts',(-1.66302528100851,3.2047573351356,50.1419356690201));
#25469=CARTESIAN_POINT('Ctrl Pts',(-1.64416607327307,3.21241614219289,50.1419356690201));
#25470=CARTESIAN_POINT('Ctrl Pts',(-1.63050764989237,3.21796288789117,50.1419356690201));
#25471=CARTESIAN_POINT('Ctrl Pts',(-1.61681763107548,3.22342028814485,50.1419356690201));
#25472=CARTESIAN_POINT('Ctrl Pts',(-1.60310048450323,3.22878616897892,50.1419356690201));
#25473=CARTESIAN_POINT('Ctrl Pts',(-1.49934935361373,3.26937159261787,50.1419356690201));
#25474=CARTESIAN_POINT('Ctrl Pts',(-1.39396358293742,3.30475931357794,50.1419356690201));
#25475=CARTESIAN_POINT('Ctrl Pts',(-1.28718164270173,3.33466271573062,50.1419356690201));
#25476=CARTESIAN_POINT('Ctrl Pts',(-1.27250705830324,3.33877221212788,50.1419356690201));
#25477=CARTESIAN_POINT('Ctrl Pts',(-1.2578060890262,3.34277805381692,50.1419356690201));
#25478=CARTESIAN_POINT('Ctrl Pts',(-1.24307933955038,3.34667942017771,50.1419356690201));
#25479=CARTESIAN_POINT('Ctrl Pts',(-1.1343142888667,3.37549313162601,50.1419356690201));
#25480=CARTESIAN_POINT('Ctrl Pts',(-1.02414300966639,3.39861243996722,50.1419356690201));
#25481=CARTESIAN_POINT('Ctrl Pts',(-0.912964352790102,3.41614626393955,
50.1419356690201));
#25482=CARTESIAN_POINT('Ctrl Pts',(-0.800839823126348,3.43382926013092,
50.1419356690201));
#25483=CARTESIAN_POINT('Ctrl Pts',(-0.687689772958802,3.44583109383719,
50.1419356690201));
#25484=CARTESIAN_POINT('Ctrl Pts',(-0.57393170863822,3.45221162946615,50.1419356690201));
#25485=CARTESIAN_POINT('Ctrl Pts',(-0.517744174485096,3.45536311209474,
50.1419356690201));
#25486=CARTESIAN_POINT('Ctrl Pts',(-0.461408526409719,3.45714246118396,
50.1419356690201));
#25487=CARTESIAN_POINT('Ctrl Pts',(-0.404976884272194,3.45755255339111,
50.1419356690201));
#25488=CARTESIAN_POINT('Ctrl Pts',(-0.382828817917752,3.45771350474874,
50.1419356690201));
#25489=CARTESIAN_POINT('Ctrl Pts',(-0.360665981431297,3.45766350932293,
50.1419356690201));
#25490=CARTESIAN_POINT('Ctrl Pts',(-0.338491595318107,3.45740262660176,
50.1419356690201));
#25491=CARTESIAN_POINT('Ctrl Pts',(-0.319069607657413,3.45717412598102,
50.1419356690201));
#25492=CARTESIAN_POINT('Ctrl Pts',(-0.29963625765142,3.45678368122754,50.1419356690201));
#25493=CARTESIAN_POINT('Ctrl Pts',(-0.280217211800923,3.45623222480351,
50.1419356690201));
#25494=CARTESIAN_POINT('Ctrl Pts',(-0.169127678463448,3.45307753650039,
50.1419356690201));
#25495=CARTESIAN_POINT('Ctrl Pts',(-0.0583427143113645,3.4446575462879,
50.1419356690201));
#25496=CARTESIAN_POINT('Ctrl Pts',(0.0517566714309187,3.43109029249483,
50.1419356690201));
#25497=CARTESIAN_POINT('Ctrl Pts',(0.1619205923774,3.41751508620058,50.1419356690201));
#25498=CARTESIAN_POINT('Ctrl Pts',(0.271399017497807,3.39878624930298,50.1419356690201));
#25499=CARTESIAN_POINT('Ctrl Pts',(0.379795820539998,3.37497200733603,50.1419356690201));
#25500=CARTESIAN_POINT('Ctrl Pts',(0.486364561209112,3.35155938163876,50.1419356690201));
#25501=CARTESIAN_POINT('Ctrl Pts',(0.591888593020798,3.32323100631305,50.1419356690201));
#25502=CARTESIAN_POINT('Ctrl Pts',(0.695965598027709,3.29000918333453,50.1419356690201));
#25503=CARTESIAN_POINT('Ctrl Pts',(0.752494111669767,3.27196504117911,50.1419356690201));
#25504=CARTESIAN_POINT('Ctrl Pts',(0.808595232251325,3.25247661609081,50.1419356690201));
#25505=CARTESIAN_POINT('Ctrl Pts',(0.864200056320583,3.23154273761965,50.1419356690201));
#25506=CARTESIAN_POINT('Ctrl Pts',(0.895132425874015,3.21989744468158,50.1419356690201));
#25507=CARTESIAN_POINT('Ctrl Pts',(0.925911151271962,3.20780478753332,50.1419356690201));
#25508=CARTESIAN_POINT('Ctrl Pts',(0.95652386930051,3.19526414787022,50.1419356690201));
#25509=CARTESIAN_POINT('Ctrl Pts',(0.971283574996722,3.18921776706545,50.1419356690201));
#25510=CARTESIAN_POINT('Ctrl Pts',(0.986005114395488,3.18306698947413,50.1419356690201));
#25511=CARTESIAN_POINT('Ctrl Pts',(1.0006729614489,3.17681794427023,50.1419356690201));
#25512=CARTESIAN_POINT('Ctrl Pts',(1.09911941328325,3.13487611562723,50.1419356690201));
#25513=CARTESIAN_POINT('Ctrl Pts',(1.19530574259082,3.08844806575148,50.1419356690201));
#25514=CARTESIAN_POINT('Ctrl Pts',(1.2888754082226,3.03759818775854,50.1419356690201));
#25515=CARTESIAN_POINT('Ctrl Pts',(1.38113377414939,2.98746092778726,50.1419356690201));
#25516=CARTESIAN_POINT('Ctrl Pts',(1.47084895575196,2.9330245060841,50.1419356690201));
#25517=CARTESIAN_POINT('Ctrl Pts',(1.55764760760897,2.87431181658939,50.1419356690201));
#25518=CARTESIAN_POINT('Ctrl Pts',(1.6420441453812,2.81722397466285,50.1419356690201));
#25519=CARTESIAN_POINT('Ctrl Pts',(1.72368379584051,2.7560928654494,50.1419356690201));
#25520=CARTESIAN_POINT('Ctrl Pts',(1.8021854173623,2.6909086108042,50.1419356690201));
#25521=CARTESIAN_POINT('Ctrl Pts',(1.84119638382351,2.65851563951943,50.1419356690201));
#25522=CARTESIAN_POINT('Ctrl Pts',(1.87943176375489,2.6251212793804,50.1419356690201));
#25523=CARTESIAN_POINT('Ctrl Pts',(1.91684063918177,2.59072181572648,50.1419356690201));
#25524=CARTESIAN_POINT('',(1.09167700819691,3.03490005447944,60.2013629539769));
#25525=CARTESIAN_POINT('Ctrl Pts',(-3.89175630324294,-0.568086152065643,
60.1999356690201));
#25526=CARTESIAN_POINT('Ctrl Pts',(-3.8987272303941,-0.447109501454028,
60.1999356690201));
#25527=CARTESIAN_POINT('Ctrl Pts',(-3.89963247433286,-0.326050566837215,
60.1999356690201));
#25528=CARTESIAN_POINT('Ctrl Pts',(-3.89469346032466,-0.205273455014232,
60.1999356690201));
#25529=CARTESIAN_POINT('Ctrl Pts',(-3.88967463525396,-0.0825446683014876,
60.1999356690201));
#25530=CARTESIAN_POINT('Ctrl Pts',(-3.87862081872039,0.0398939529422601,
60.1999356690201));
#25531=CARTESIAN_POINT('Ctrl Pts',(-3.86171172561488,0.161648217750859,
60.1999356690201));
#25532=CARTESIAN_POINT('Ctrl Pts',(-3.84497309684275,0.282175050700306,
60.1999356690201));
#25533=CARTESIAN_POINT('Ctrl Pts',(-3.82249613254274,0.402031999762345,
60.1999356690201));
#25534=CARTESIAN_POINT('Ctrl Pts',(-3.79441072525008,0.520813100294654,
60.1999356690201));
#25535=CARTESIAN_POINT('Ctrl Pts',(-3.78992600069583,0.539780264010207,
60.1999356690201));
#25536=CARTESIAN_POINT('Ctrl Pts',(-3.78530028918843,0.558710999976427,
60.1999356690201));
#25537=CARTESIAN_POINT('Ctrl Pts',(-3.78053494608037,0.577601735753827,
60.1999356690201));
#25538=CARTESIAN_POINT('Ctrl Pts',(-3.75095064085873,0.694879606502539,
60.1999356690201));
#25539=CARTESIAN_POINT('Ctrl Pts',(-3.71598243568719,0.810643347701233,
60.1999356690201));
#25540=CARTESIAN_POINT('Ctrl Pts',(-3.67581069153357,0.924515931242179,
60.1999356690201));
#25541=CARTESIAN_POINT('Ctrl Pts',(-3.63593607793549,1.03754625551056,60.1999356690201));
#25542=CARTESIAN_POINT('Ctrl Pts',(-3.59093410589017,1.14871401938861,60.1999356690201));
#25543=CARTESIAN_POINT('Ctrl Pts',(-3.54093868932249,1.25762272055214,60.1999356690201));
#25544=CARTESIAN_POINT('Ctrl Pts',(-3.5082103591865,1.32891725455281,60.1999356690201));
#25545=CARTESIAN_POINT('Ctrl Pts',(-3.47334131077137,1.39924310877329,60.1999356690201));
#25546=CARTESIAN_POINT('Ctrl Pts',(-3.4363606857526,1.46848029561757,60.1999356690201));
#25547=CARTESIAN_POINT('Ctrl Pts',(-3.42737390205831,1.48530585282365,60.1999356690201));
#25548=CARTESIAN_POINT('Ctrl Pts',(-3.41826239001577,1.50206708169468,60.1999356690201));
#25549=CARTESIAN_POINT('Ctrl Pts',(-3.40902651492644,1.51876218737697,60.1999356690201));
#25550=CARTESIAN_POINT('Ctrl Pts',(-3.40039237704251,1.53436957087373,60.1999356690201));
#25551=CARTESIAN_POINT('Ctrl Pts',(-3.39165409022965,1.54991094148913,60.1999356690201));
#25552=CARTESIAN_POINT('Ctrl Pts',(-3.38281350142322,1.56538292504736,60.1999356690201));
#25553=CARTESIAN_POINT('Ctrl Pts',(-3.32466726855337,1.66714510159842,60.1999356690201));
#25554=CARTESIAN_POINT('Ctrl Pts',(-3.2620816872634,1.7659391973382,60.1999356690201));
#25555=CARTESIAN_POINT('Ctrl Pts',(-3.19521186487262,1.8614144002759,60.1999356690201));
#25556=CARTESIAN_POINT('Ctrl Pts',(-3.12913578401535,1.95575631720682,60.1999356690201));
#25557=CARTESIAN_POINT('Ctrl Pts',(-3.05887605633773,2.04685826973845,60.1999356690201));
#25558=CARTESIAN_POINT('Ctrl Pts',(-2.98454669867674,2.13434644657347,60.1999356690201));
#25559=CARTESIAN_POINT('Ctrl Pts',(-2.91228904583423,2.21939615651987,60.1999356690201));
#25560=CARTESIAN_POINT('Ctrl Pts',(-2.83618495656178,2.3010311258843,60.1999356690201));
#25561=CARTESIAN_POINT('Ctrl Pts',(-2.75631280208009,2.37886721205882,60.1999356690201));
#25562=CARTESIAN_POINT('Ctrl Pts',(-2.69729820240156,2.43637743568984,60.1999356690201));
#25563=CARTESIAN_POINT('Ctrl Pts',(-2.63622598358031,2.49181298681209,60.1999356690201));
#25564=CARTESIAN_POINT('Ctrl Pts',(-2.57312038377187,2.54500207854132,60.1999356690201));
#25565=CARTESIAN_POINT('Ctrl Pts',(-2.55330118941283,2.5617068551374,60.1999356690201));
#25566=CARTESIAN_POINT('Ctrl Pts',(-2.53328138931353,2.57818993465074,60.1999356690201));
#25567=CARTESIAN_POINT('Ctrl Pts',(-2.51306162809949,2.59444567022016,60.1999356690201));
#25568=CARTESIAN_POINT('Ctrl Pts',(-2.50195032082291,2.60337863787526,60.1999356690201));
#25569=CARTESIAN_POINT('Ctrl Pts',(-2.49077942647284,2.61224225258535,60.1999356690201));
#25570=CARTESIAN_POINT('Ctrl Pts',(-2.47955702841876,2.62102952177222,60.1999356690201));
#25571=CARTESIAN_POINT('Ctrl Pts',(-2.44671026938688,2.64674891901145,60.1999356690201));
#25572=CARTESIAN_POINT('Ctrl Pts',(-2.413404245263,2.67182898317495,60.1999356690201));
#25573=CARTESIAN_POINT('Ctrl Pts',(-2.37964494215065,2.69625243206787,60.1999356690201));
#25574=CARTESIAN_POINT('Ctrl Pts',(-2.28865280762842,2.76208144932471,60.1999356690201));
#25575=CARTESIAN_POINT('Ctrl Pts',(-2.19436954231683,2.82314381468693,60.1999356690201));
#25576=CARTESIAN_POINT('Ctrl Pts',(-2.09722649760078,2.8794215842726,60.1999356690201));
#25577=CARTESIAN_POINT('Ctrl Pts',(-1.99889796386925,2.93638614186099,60.1999356690201));
#25578=CARTESIAN_POINT('Ctrl Pts',(-1.89763846862526,2.98844876165294,60.1999356690201));
#25579=CARTESIAN_POINT('Ctrl Pts',(-1.79387705421774,3.0355402934247,60.1999356690201));
#25580=CARTESIAN_POINT('Ctrl Pts',(-1.69039303401084,3.08250593140553,60.1999356690201));
#25581=CARTESIAN_POINT('Ctrl Pts',(-1.58441947561242,3.1245270555689,60.1999356690201));
#25582=CARTESIAN_POINT('Ctrl Pts',(-1.47637852350488,3.16148394148629,60.1999356690201));
#25583=CARTESIAN_POINT('Ctrl Pts',(-1.42830734780708,3.17792734485811,60.1999356690201));
#25584=CARTESIAN_POINT('Ctrl Pts',(-1.37982693903537,3.193367516023,60.1999356690201));
#25585=CARTESIAN_POINT('Ctrl Pts',(-1.33097503044475,3.20779061651805,60.1999356690201));
#25586=CARTESIAN_POINT('Ctrl Pts',(-1.31592975202495,3.21223260392212,60.1999356690201));
#25587=CARTESIAN_POINT('Ctrl Pts',(-1.30084698790465,3.21657873798348,60.1999356690201));
#25588=CARTESIAN_POINT('Ctrl Pts',(-1.28573522280096,3.2208265122493,60.1999356690201));
#25589=CARTESIAN_POINT('Ctrl Pts',(-1.17699127245041,3.2513934083526,60.1999356690201));
#25590=CARTESIAN_POINT('Ctrl Pts',(-1.06700275791658,3.27680121139375,60.1999356690201));
#25591=CARTESIAN_POINT('Ctrl Pts',(-0.95619161988832,3.29700942866175,60.1999356690201));
#25592=CARTESIAN_POINT('Ctrl Pts',(-0.847048097392534,3.31691352905487,
60.1999356690201));
#25593=CARTESIAN_POINT('Ctrl Pts',(-0.737105558427078,3.33177324724764,
60.19993566902));
#25594=CARTESIAN_POINT('Ctrl Pts',(-0.626766108775439,3.34149844302225,
60.19993566902));
#25595=CARTESIAN_POINT('Ctrl Pts',(-0.513897826777057,3.35144652725363,
60.19993566902));
#25596=CARTESIAN_POINT('Ctrl Pts',(-0.400613190132631,3.35602226634987,
60.1999356690201));
#25597=CARTESIAN_POINT('Ctrl Pts',(-0.287356666109463,3.35507364513194,
60.1999356690201));
#25598=CARTESIAN_POINT('Ctrl Pts',(-0.230728404097879,3.35459933452298,
60.1999356690201));
#25599=CARTESIAN_POINT('Ctrl Pts',(-0.174107487097954,3.35274305441458,
60.1999356690201));
#25600=CARTESIAN_POINT('Ctrl Pts',(-0.117552012598016,3.34948051185152,
60.1999356690201));
#25601=CARTESIAN_POINT('Ctrl Pts',(-0.088900957870724,3.34782770482708,
60.1999356690201));
#25602=CARTESIAN_POINT('Ctrl Pts',(-0.0602667307051432,3.34581393210833,
60.19993566902));
#25603=CARTESIAN_POINT('Ctrl Pts',(-0.0316571036748412,3.3434356885107,
60.19993566902));
#25604=CARTESIAN_POINT('Ctrl Pts',(-0.0117570385253347,3.34178144805227,
60.19993566902));
#25605=CARTESIAN_POINT('Ctrl Pts',(0.00813420303698488,3.3399505393087,
60.1999356690201));
#25606=CARTESIAN_POINT('Ctrl Pts',(0.0280024783019314,3.33794291627126,
60.1999356690201));
#25607=CARTESIAN_POINT('Ctrl Pts',(0.0359537625046807,3.33713946548705,
60.1999356690201));
#25608=CARTESIAN_POINT('Ctrl Pts',(0.0439007585439898,3.33630777992627,
60.1999356690201));
#25609=CARTESIAN_POINT('Ctrl Pts',(0.051841555696066,3.33544802060429,60.1999356690201));
#25610=CARTESIAN_POINT('Ctrl Pts',(0.157654292629215,3.32399155279385,60.19993566902));
#25611=CARTESIAN_POINT('Ctrl Pts',(0.262528675282593,3.3075376814079,60.19993566902));
#25612=CARTESIAN_POINT('Ctrl Pts',(0.366101449193363,3.28600352068117,60.19993566902));
#25613=CARTESIAN_POINT('Ctrl Pts',(0.466999985779342,3.26502536955233,60.19993566902));
#25614=CARTESIAN_POINT('Ctrl Pts',(0.566663925722094,3.23922566881805,60.1999356690201));
#25615=CARTESIAN_POINT('Ctrl Pts',(0.664738724796578,3.20848274425607,60.1999356690201));
#25616=CARTESIAN_POINT('Ctrl Pts',(0.733222271488591,3.18701561376427,60.1999356690201));
#25617=CARTESIAN_POINT('Ctrl Pts',(0.800930585390643,3.1631372754956,60.19993566902));
#25618=CARTESIAN_POINT('Ctrl Pts',(0.867734791776628,3.13679351929711,60.19993566902));
#25619=CARTESIAN_POINT('Ctrl Pts',(0.943633142286453,3.10686355305895,60.1999356690201));
#25620=CARTESIAN_POINT('Ctrl Pts',(1.01836477737186,3.07375102185424,60.1999356690201));
#25621=CARTESIAN_POINT('Ctrl Pts',(1.09179082753359,3.03758696058814,60.1999356690201));
#25622=CARTESIAN_POINT('Ctrl Pts',(1.09082349994205,3.03252727184343,60.2013629539769));
#25623=CARTESIAN_POINT('Ctrl Pts',(1.10461504357036,3.02756634699704,60.2008871923247));
#25624=CARTESIAN_POINT('Ctrl Pts',(1.11837274419444,3.02251133744672,60.2004114306724));
#25625=CARTESIAN_POINT('Ctrl Pts',(1.13209532136445,3.01736271366979,60.1999356690201));
#25626=CARTESIAN_POINT('Ctrl Pts',(3.93531215953305,-0.0522584680823885,
60.611665739885));
#25627=CARTESIAN_POINT('Ctrl Pts',(3.91807438294499,-1.35546450485723,60.5457849464951));
#25628=CARTESIAN_POINT('Ctrl Pts',(2.48753474466723,-3.92031944802341,60.4140672787108));
#25629=CARTESIAN_POINT('Ctrl Pts',(-1.93244502466786,-4.22618854783819,
60.2165127365322));
#25630=CARTESIAN_POINT('Ctrl Pts',(-4.59187364716804,-0.689556313732268,
60.0190021133494));
#25631=CARTESIAN_POINT('Ctrl Pts',(-3.08810139139498,3.46876832474886,59.8214914901664));
#25632=CARTESIAN_POINT('Ctrl Pts',(1.2190055499893,4.48184773125158,59.6239808669837));
#25633=CARTESIAN_POINT('Ctrl Pts',(4.41935766022409,1.42755566308068,59.4264702438007));
#25634=CARTESIAN_POINT('Ctrl Pts',(3.61039927513463,-2.92146360824966,59.2289596206179));
#25635=CARTESIAN_POINT('Ctrl Pts',(-0.474465609420469,-4.62008497587082,
59.031448997435));
#25636=CARTESIAN_POINT('Ctrl Pts',(-4.12875297584294,-2.12677531987275,
58.8339383742521));
#25637=CARTESIAN_POINT('Ctrl Pts',(-4.03706704399223,2.29609679293635,58.6364277510693));
#25638=CARTESIAN_POINT('Ctrl Pts',(-0.282523388749893,4.63574983727625,
58.4389171278863));
#25639=CARTESIAN_POINT('Ctrl Pts',(3.72834203975631,2.76936788312511,58.2414065047037));
#25640=CARTESIAN_POINT('Ctrl Pts',(4.35648590055403,-1.60965577352385,58.0438958815205));
#25641=CARTESIAN_POINT('Ctrl Pts',(1.03198383136335,-4.52824147705999,57.846385258338));
#25642=CARTESIAN_POINT('Ctrl Pts',(-3.22883644391126,-3.33834830418739,
57.6488746351548));
#25643=CARTESIAN_POINT('Ctrl Pts',(-4.56013173592111,0.880429806891776,
57.4513640119722));
#25644=CARTESIAN_POINT('Ctrl Pts',(-1.75401569458227,4.30039378824156,57.2538533887891));
#25645=CARTESIAN_POINT('Ctrl Pts',(2.64351991746123,3.81860699986849,57.0563427656064));
#25646=CARTESIAN_POINT('Ctrl Pts',(4.64258801360327,-0.127804668657566,
56.8588321424235));
#25647=CARTESIAN_POINT('Ctrl Pts',(2.42943246328811,-3.95825912771161,56.6613215192406));
#25648=CARTESIAN_POINT('Ctrl Pts',(-1.98794896560828,-4.19738206968733,
56.4638108960578));
#25649=CARTESIAN_POINT('Ctrl Pts',(-4.60166281376544,-0.628217116468037,
56.2663002728748));
#25650=CARTESIAN_POINT('Ctrl Pts',(-3.04028452160891,3.51092970722542,56.0687896496921));
#25651=CARTESIAN_POINT('Ctrl Pts',(1.27954620218712,4.46460736115508,55.8712790265091));
#25652=CARTESIAN_POINT('Ctrl Pts',(4.43844369529037,1.36754339805686,55.6737684033263));
#25653=CARTESIAN_POINT('Ctrl Pts',(3.5703378822165,-2.9702937203288,55.4762577801434));
#25654=CARTESIAN_POINT('Ctrl Pts',(-0.537138177867132,-4.61318111026358,
55.2787471569606));
#25655=CARTESIAN_POINT('Ctrl Pts',(-4.15726836571013,-2.07052580696252,
55.0812365337776));
#25656=CARTESIAN_POINT('Ctrl Pts',(-4.0055058351096,2.3507191192728,54.8837259105949));
#25657=CARTESIAN_POINT('Ctrl Pts',(-0.219544848133634,4.6391548196919,54.6862152874118));
#25658=CARTESIAN_POINT('Ctrl Pts',(3.76560934971691,2.7184818598511,54.4887046642291));
#25659=CARTESIAN_POINT('Ctrl Pts',(4.33422334064896,-1.6686717358934,54.2911940410462));
#25660=CARTESIAN_POINT('Ctrl Pts',(0.970393252027999,-4.54183821290554,
54.0936834178634));
#25661=CARTESIAN_POINT('Ctrl Pts',(-3.27387540341237,-3.29419145471466,
53.8961727946805));
#25662=CARTESIAN_POINT('Ctrl Pts',(-4.54775436371161,0.942277677121238,
53.6986621714976));
#25663=CARTESIAN_POINT('Ctrl Pts',(-1.69545252177553,4.3238175883347,53.5011515483147));
#25664=CARTESIAN_POINT('Ctrl Pts',(2.69513497791465,3.78235449748423,53.3036409251319));
#25665=CARTESIAN_POINT('Ctrl Pts',(4.64042386796999,-0.190841576116406,
53.106130301949));
#25666=CARTESIAN_POINT('Ctrl Pts',(2.37545391819541,-3.99088714264033,52.9086196787661));
#25667=CARTESIAN_POINT('Ctrl Pts',(-2.04476960905902,-4.1699974048953,52.7111090555833));
#25668=CARTESIAN_POINT('Ctrl Pts',(-4.60976724491823,-0.56566667320796,
52.5135984324004));
#25669=CARTESIAN_POINT('Ctrl Pts',(-2.99232933597807,3.55189543258844,52.3160878092175));
#25670=CARTESIAN_POINT('Ctrl Pts',(1.34007067120665,4.44681699605373,52.1185771860347));
#25671=CARTESIAN_POINT('Ctrl Pts',(4.45658477518138,1.30714442139082,51.9210665628518));
#25672=CARTESIAN_POINT('Ctrl Pts',(3.52971349926043,-3.0185137753419,51.7235559396689));
#25673=CARTESIAN_POINT('Ctrl Pts',(-0.59982375698502,-4.60544720963951,
51.5260453164861));
#25674=CARTESIAN_POINT('Ctrl Pts',(-4.18483276393422,-2.01390467452604,
51.3285346933032));
#25675=CARTESIAN_POINT('Ctrl Pts',(-3.97355361721659,2.40495431726563,51.1310240701203));
#25676=CARTESIAN_POINT('Ctrl Pts',(-0.155841917726807,4.64159855987091,
50.9335134469375));
#25677=CARTESIAN_POINT('Ctrl Pts',(3.80082132445766,2.66731114812503,50.7360028237546));
#25678=CARTESIAN_POINT('Ctrl Pts',(4.31389481065517,-1.7278093001962,50.5384922005718));
#25679=CARTESIAN_POINT('Ctrl Pts',(0.90291182050654,-4.55380384351974,50.3409815773889));
#25680=CARTESIAN_POINT('Ctrl Pts',(-1.90071216242741,-3.68416167811652,
50.2093078286003));
#25681=CARTESIAN_POINT('Ctrl Pts',(-2.81196449438821,-2.75359200998455,
50.143470954206));
#25682=CARTESIAN_POINT('Ctrl Pts',(3.69578503881393,-0.0490776987086958,
60.4733624971722));
#25683=CARTESIAN_POINT('Ctrl Pts',(3.67959645853517,-1.27296266080429,60.4074817037822));
#25684=CARTESIAN_POINT('Ctrl Pts',(2.33612819521839,-3.68170487524816,60.2757640359979));
#25685=CARTESIAN_POINT('Ctrl Pts',(-1.81482462406369,-3.96895691450318,
60.0782094938193));
#25686=CARTESIAN_POINT('Ctrl Pts',(-4.31238418640244,-0.647585707156146,
59.8806988706365));
#25687=CARTESIAN_POINT('Ctrl Pts',(-2.90014068973178,3.25763790978137,59.6831882474536));
#25688=CARTESIAN_POINT('Ctrl Pts',(1.14480943092864,4.20905511937002,59.4856776242708));
#25689=CARTESIAN_POINT('Ctrl Pts',(4.15036857552919,1.34066591106553,59.2881670010878));
#25690=CARTESIAN_POINT('Ctrl Pts',(3.39064833595576,-2.74364549929111,59.0906563779051));
#25691=CARTESIAN_POINT('Ctrl Pts',(-0.445586736106843,-4.33887840142735,
58.8931457547221));
#25692=CARTESIAN_POINT('Ctrl Pts',(-3.87745186620453,-1.99732679123403,
58.6956351315393));
#25693=CARTESIAN_POINT('Ctrl Pts',(-3.79134649985317,2.15634232584225,58.4981245083564));
#25694=CARTESIAN_POINT('Ctrl Pts',(-0.265327290676925,4.35358980374317,
58.3006138851735));
#25695=CARTESIAN_POINT('Ctrl Pts',(3.50141238395363,2.60080724844964,58.1031032619907));
#25696=CARTESIAN_POINT('Ctrl Pts',(4.09132357494655,-1.51168229717659,57.9055926388077));
#25697=CARTESIAN_POINT('Ctrl Pts',(0.969170995752236,-4.25262505860291,
57.7080820156251));
#25698=CARTESIAN_POINT('Ctrl Pts',(-3.03230974784991,-3.13515604780627,
57.5105713924419));
#25699=CARTESIAN_POINT('Ctrl Pts',(-4.28257428163909,0.82684147435525,57.3130607692593));
#25700=CARTESIAN_POINT('Ctrl Pts',(-1.64725559220977,4.03864557099769,57.1155501460762));
#25701=CARTESIAN_POINT('Ctrl Pts',(2.48261915820144,3.58618326758065,56.9180395228936));
#25702=CARTESIAN_POINT('Ctrl Pts',(4.36001176691602,-0.120025696353209,
56.7205288997105));
#25703=CARTESIAN_POINT('Ctrl Pts',(2.28156237336314,-3.71733531443183,56.5230182765278));
#25704=CARTESIAN_POINT('Ctrl Pts',(-1.86695025634065,-3.94190377445863,
56.3255076533448));
#25705=CARTESIAN_POINT('Ctrl Pts',(-4.3215775245638,-0.589979987875952,
56.127997030162));
#25706=CARTESIAN_POINT('Ctrl Pts',(-2.85523424653382,3.2972330931508,55.9304864069791));
#25707=CARTESIAN_POINT('Ctrl Pts',(1.20166520946979,4.19286410343959,55.7329757837963));
#25708=CARTESIAN_POINT('Ctrl Pts',(4.16829291799269,1.28430635882949,55.5354651606134));
#25709=CARTESIAN_POINT('Ctrl Pts',(3.35302532396108,-2.78950351267095,55.3379545374305));
#25710=CARTESIAN_POINT('Ctrl Pts',(-0.504444669459887,-4.33239474722486,
55.1404439142477));
#25711=CARTESIAN_POINT('Ctrl Pts',(-3.90423163537527,-1.94450096704862,
54.9429332910648));
#25712=CARTESIAN_POINT('Ctrl Pts',(-3.76170629880514,2.20764000396175,54.745422667882));
#25713=CARTESIAN_POINT('Ctrl Pts',(-0.206182008488301,4.35678753814367,
54.5479120446991));
#25714=CARTESIAN_POINT('Ctrl Pts',(3.53641137793574,2.55301845918035,54.3504014215162));
#25715=CARTESIAN_POINT('Ctrl Pts',(4.07041605033671,-1.56710618781973,54.1528907983333));
#25716=CARTESIAN_POINT('Ctrl Pts',(0.911329195048302,-4.26539421410509,
53.9553801751505));
#25717=CARTESIAN_POINT('Ctrl Pts',(-3.07460736134031,-3.09368685374319,
53.7578695519676));
#25718=CARTESIAN_POINT('Ctrl Pts',(-4.27095027185859,0.884924905658877,
53.5603589287848));
#25719=CARTESIAN_POINT('Ctrl Pts',(-1.59225693159265,4.06064365562909,53.3628483056018));
#25720=CARTESIAN_POINT('Ctrl Pts',(2.53109261099707,3.55213731379099,53.165337682419));
#25721=CARTESIAN_POINT('Ctrl Pts',(4.35797934439678,-0.179225792822079,
52.9678270592361));
#25722=CARTESIAN_POINT('Ctrl Pts',(2.23086929203101,-3.74797738919779,52.7703164360533));
#25723=CARTESIAN_POINT('Ctrl Pts',(-1.92031244857547,-3.91618590753258,
52.5728058128704));
#25724=CARTESIAN_POINT('Ctrl Pts',(-4.32918867056402,-0.531236746425136,
52.3752951896875));
#25725=CARTESIAN_POINT('Ctrl Pts',(-2.81019790623775,3.33570539439735,52.1777845665047));
#25726=CARTESIAN_POINT('Ctrl Pts',(1.25850578983969,4.17615656855767,51.9802739433218));
#25727=CARTESIAN_POINT('Ctrl Pts',(4.18532982102126,1.2275836325824,51.782763320139));
#25728=CARTESIAN_POINT('Ctrl Pts',(3.31487358893889,-2.83478860078181,51.5852526969561));
#25729=CARTESIAN_POINT('Ctrl Pts',(-0.563314821575283,-4.32513157900353,
51.3877420737732));
#25730=CARTESIAN_POINT('Ctrl Pts',(-3.93011829605955,-1.89132614236984,
51.1902314505903));
#25731=CARTESIAN_POINT('Ctrl Pts',(-3.73169888794198,2.2585741167318,50.9927208274075));
#25732=CARTESIAN_POINT('Ctrl Pts',(-0.146356427293726,4.35908253737783,
50.7952102042246));
#25733=CARTESIAN_POINT('Ctrl Pts',(3.56948013694607,2.50496230933603,50.5976995810418));
#25734=CARTESIAN_POINT('Ctrl Pts',(4.05132483877166,-1.62264427896017,50.4001889578589));
#25735=CARTESIAN_POINT('Ctrl Pts',(0.847955095382388,-4.2766315433972,50.202678334676));
#25736=CARTESIAN_POINT('Ctrl Pts',(-1.78502321752906,-3.45992110881751,
50.0710045858874));
#25737=CARTESIAN_POINT('Ctrl Pts',(-2.64081116992483,-2.58599159125054,
50.0051677114931));
#25738=CARTESIAN_POINT('Ctrl Pts',(3.45625791809479,-0.045896929335003,
60.3350592544593));
#25739=CARTESIAN_POINT('Ctrl Pts',(3.44111853412534,-1.19046081675135,60.2691784610693));
#25740=CARTESIAN_POINT('Ctrl Pts',(2.18472164576956,-3.4430903024729,60.1374607932851));
#25741=CARTESIAN_POINT('Ctrl Pts',(-1.69720422345953,-3.71172528116816,
59.9399062511065));
#25742=CARTESIAN_POINT('Ctrl Pts',(-4.03289472563685,-0.605615100580024,
59.7423956279237));
#25743=CARTESIAN_POINT('Ctrl Pts',(-2.71217998806857,3.04650749481388,59.5448850047407));
#25744=CARTESIAN_POINT('Ctrl Pts',(1.07061331186798,3.93626250748847,59.3473743815579));
#25745=CARTESIAN_POINT('Ctrl Pts',(3.88137949083429,1.25377615905039,59.149863758375));
#25746=CARTESIAN_POINT('Ctrl Pts',(3.17089739677689,-2.56582739033256,58.9523531351921));
#25747=CARTESIAN_POINT('Ctrl Pts',(-0.416707862793216,-4.05767182698388,
58.7548425120093));
#25748=CARTESIAN_POINT('Ctrl Pts',(-3.62615075656612,-1.8678782625953,58.5573318888264));
#25749=CARTESIAN_POINT('Ctrl Pts',(-3.5456259557141,2.01658785874816,58.3598212656436));
#25750=CARTESIAN_POINT('Ctrl Pts',(-0.248131192603958,4.07142977021011,
58.1623106424607));
#25751=CARTESIAN_POINT('Ctrl Pts',(3.27448272815097,2.43224661377418,57.9648000192779));
#25752=CARTESIAN_POINT('Ctrl Pts',(3.82616124933907,-1.41370882082934,57.7672893960949));
#25753=CARTESIAN_POINT('Ctrl Pts',(0.906358160141125,-3.97700864014582,
57.5697787729122));
#25754=CARTESIAN_POINT('Ctrl Pts',(-2.83578305178858,-2.93196379142515,
57.3722681497291));
#25755=CARTESIAN_POINT('Ctrl Pts',(-4.00501682735706,0.773253141818731,
57.1747575265465));
#25756=CARTESIAN_POINT('Ctrl Pts',(-1.54049548983728,3.77689735375381,56.9772469033634));
#25757=CARTESIAN_POINT('Ctrl Pts',(2.32171839894166,3.35375953529281,56.7797362801807));
#25758=CARTESIAN_POINT('Ctrl Pts',(4.07743552022877,-0.112246724048854,
56.5822256569977));
#25759=CARTESIAN_POINT('Ctrl Pts',(2.13369228343817,-3.47641150115206,56.3847150338149));
#25760=CARTESIAN_POINT('Ctrl Pts',(-1.74595154707302,-3.68642547922993,
56.187204410632));
#25761=CARTESIAN_POINT('Ctrl Pts',(-4.04149223536218,-0.551742859283865,
55.9896937874491));
#25762=CARTESIAN_POINT('Ctrl Pts',(-2.67018397145873,3.08353647907615,55.7921831642663));
#25763=CARTESIAN_POINT('Ctrl Pts',(1.12378421675247,3.9211208457241,55.5946725410834));
#25764=CARTESIAN_POINT('Ctrl Pts',(3.898142140695,1.20106931960212,55.3971619179006));
#25765=CARTESIAN_POINT('Ctrl Pts',(3.13571276570568,-2.60871330501309,55.1996512947176));
#25766=CARTESIAN_POINT('Ctrl Pts',(-0.471751161052643,-4.05160838418615,
55.0021406715349));
#25767=CARTESIAN_POINT('Ctrl Pts',(-3.65119490504041,-1.81847612713471,
54.8046300483519));
#25768=CARTESIAN_POINT('Ctrl Pts',(-3.51790676250068,2.0645608886507,54.6071194251692));
#25769=CARTESIAN_POINT('Ctrl Pts',(-0.192819168842966,4.07442025659543,
54.4096088019862));
#25770=CARTESIAN_POINT('Ctrl Pts',(3.30721340615459,2.38755505850958,54.2120981788034));
#25771=CARTESIAN_POINT('Ctrl Pts',(3.80660876002445,-1.46554063974607,54.0145875556205));
#25772=CARTESIAN_POINT('Ctrl Pts',(0.85226513806861,-3.98895021530463,53.8170769324376));
#25773=CARTESIAN_POINT('Ctrl Pts',(-2.87533931926824,-2.89318225277171,
53.6195663092547));
#25774=CARTESIAN_POINT('Ctrl Pts',(-3.99414618000558,0.827572134196515,
53.4220556860719));
#25775=CARTESIAN_POINT('Ctrl Pts',(-1.48906134140977,3.79746972292347,53.2245450628891));
#25776=CARTESIAN_POINT('Ctrl Pts',(2.3670502440795,3.32192013009776,53.0270344397061));
#25777=CARTESIAN_POINT('Ctrl Pts',(4.07553482082357,-0.167610009527757,
52.8295238165233));
#25778=CARTESIAN_POINT('Ctrl Pts',(2.0862846658666,-3.50506763575524,52.6320131933405));
#25779=CARTESIAN_POINT('Ctrl Pts',(-1.79585528809192,-3.66237441016986,
52.4345025701575));
#25780=CARTESIAN_POINT('Ctrl Pts',(-4.04861009620979,-0.496806819642315,
52.2369919469747));
#25781=CARTESIAN_POINT('Ctrl Pts',(-2.62806647649744,3.11951535620625,52.0394813237918));
#25782=CARTESIAN_POINT('Ctrl Pts',(1.17694090847273,3.90549614106162,51.841970700609));
#25783=CARTESIAN_POINT('Ctrl Pts',(3.91407486686113,1.14802284377398,51.6444600774261));
#25784=CARTESIAN_POINT('Ctrl Pts',(3.10003367861737,-2.65106342622172,51.4469494542432));
#25785=CARTESIAN_POINT('Ctrl Pts',(-0.526805886165546,-4.04481594836757,
51.2494388310604));
#25786=CARTESIAN_POINT('Ctrl Pts',(-3.67540382818486,-1.76874761021364,
51.0519282078775));
#25787=CARTESIAN_POINT('Ctrl Pts',(-3.48984415866736,2.11219391619798,50.8544175846946));
#25788=CARTESIAN_POINT('Ctrl Pts',(-0.136870936860638,4.07656651488476,
50.6569069615117));
#25789=CARTESIAN_POINT('Ctrl Pts',(3.33813894943446,2.34261347054704,50.4593963383289));
#25790=CARTESIAN_POINT('Ctrl Pts',(3.78875486688816,-1.51747925772413,50.261885715146));
#25791=CARTESIAN_POINT('Ctrl Pts',(0.792998370258228,-3.99945924327466,
50.0643750919632));
#25792=CARTESIAN_POINT('Ctrl Pts',(-1.6693342726307,-3.23568053951851,49.9327013431746));
#25793=CARTESIAN_POINT('Ctrl Pts',(-2.46965784546145,-2.41839117251652,
49.8668644687803));
#25794=CARTESIAN_POINT('Ctrl Pts',(3.21673079737567,-0.0427161599613103,
60.1967560117465));
#25795=CARTESIAN_POINT('Ctrl Pts',(3.20264060971551,-1.10795897269841,60.1308752183565));
#25796=CARTESIAN_POINT('Ctrl Pts',(2.03331509632072,-3.20447572969764,59.9991575505722));
#25797=CARTESIAN_POINT('Ctrl Pts',(-1.57958382285538,-3.45449364783315,
59.8016030083936));
#25798=CARTESIAN_POINT('Ctrl Pts',(-3.75340526487125,-0.563644494003902,
59.6040923852108));
#25799=CARTESIAN_POINT('Ctrl Pts',(-2.52421928640537,2.83537707984639,59.4065817620279));
#25800=CARTESIAN_POINT('Ctrl Pts',(0.996417192807324,3.66346989560692,59.2090711388451));
#25801=CARTESIAN_POINT('Ctrl Pts',(3.61239040613939,1.16688640703525,59.0115605156621));
#25802=CARTESIAN_POINT('Ctrl Pts',(2.95114645759801,-2.38800928137401,58.8140498924793));
#25803=CARTESIAN_POINT('Ctrl Pts',(-0.387828989479593,-3.77646525254041,
58.6165392692965));
#25804=CARTESIAN_POINT('Ctrl Pts',(-3.3748496469277,-1.73842973395658,58.4190286461135));
#25805=CARTESIAN_POINT('Ctrl Pts',(-3.29990541157504,1.87683339165406,58.2215180229308));
#25806=CARTESIAN_POINT('Ctrl Pts',(-0.230935094530989,3.78926973667704,
58.0240073997477));
#25807=CARTESIAN_POINT('Ctrl Pts',(3.04755307234829,2.2636859790987,57.826496776565));
#25808=CARTESIAN_POINT('Ctrl Pts',(3.56099892373158,-1.31573534448208,57.628986153382));
#25809=CARTESIAN_POINT('Ctrl Pts',(0.843545324530011,-3.70139222168874,
57.4314755301993));
#25810=CARTESIAN_POINT('Ctrl Pts',(-2.63925635572723,-2.72877153504402,
57.2339649070163));
#25811=CARTESIAN_POINT('Ctrl Pts',(-3.72745937307503,0.719664809282207,
57.0364542838335));
#25812=CARTESIAN_POINT('Ctrl Pts',(-1.43373538746479,3.51514913650993,56.8389436606506));
#25813=CARTESIAN_POINT('Ctrl Pts',(2.16081763968186,3.12133580300496,56.6414330374678));
#25814=CARTESIAN_POINT('Ctrl Pts',(3.79485927354153,-0.104467751744498,
56.4439224142849));
#25815=CARTESIAN_POINT('Ctrl Pts',(1.9858221935132,-3.23548768787228,56.246411791102));
#25816=CARTESIAN_POINT('Ctrl Pts',(-1.62495283780538,-3.43094718400122,
56.0489011679192));
#25817=CARTESIAN_POINT('Ctrl Pts',(-3.76140694616054,-0.513505730691779,
55.8513905447362));
#25818=CARTESIAN_POINT('Ctrl Pts',(-2.48513369638366,2.86983986500152,55.6538799215535));
#25819=CARTESIAN_POINT('Ctrl Pts',(1.04590322403516,3.6493775880086,55.4563692983705));
#25820=CARTESIAN_POINT('Ctrl Pts',(3.62799136339733,1.11783228037474,55.2588586751877));
#25821=CARTESIAN_POINT('Ctrl Pts',(2.91840020745027,-2.42792309735524,55.0613480520048));
#25822=CARTESIAN_POINT('Ctrl Pts',(-0.439057652645399,-3.77082202114744,
54.863837428822));
#25823=CARTESIAN_POINT('Ctrl Pts',(-3.39815817470555,-1.69245128722081,
54.666326805639));
#25824=CARTESIAN_POINT('Ctrl Pts',(-3.27410722619621,1.92148177333965,54.4688161824563));
#25825=CARTESIAN_POINT('Ctrl Pts',(-0.179456329197637,3.79205297504719,
54.2713055592733));
#25826=CARTESIAN_POINT('Ctrl Pts',(3.07801543437343,2.22209165783883,54.0737949360905));
#25827=CARTESIAN_POINT('Ctrl Pts',(3.54280146971219,-1.3639750916724,53.8762843129076));
#25828=CARTESIAN_POINT('Ctrl Pts',(0.793201081088917,-3.71250621650416,
53.6787736897248));
#25829=CARTESIAN_POINT('Ctrl Pts',(-2.67607127719618,-2.69267765180024,
53.4812630665419));
#25830=CARTESIAN_POINT('Ctrl Pts',(-3.71734208815255,0.770219362734153,
53.283752443359));
#25831=CARTESIAN_POINT('Ctrl Pts',(-1.3858657512269,3.53429579021786,53.0862418201761));
#25832=CARTESIAN_POINT('Ctrl Pts',(2.20300787716194,3.09170294640452,52.8887311969933));
#25833=CARTESIAN_POINT('Ctrl Pts',(3.79309029725036,-0.155994226233431,
52.6912205738104));
#25834=CARTESIAN_POINT('Ctrl Pts',(1.9417000397022,-3.26215788231269,52.4937099506275));
#25835=CARTESIAN_POINT('Ctrl Pts',(-1.67139812760836,-3.40856291280714,
52.2961993274447));
#25836=CARTESIAN_POINT('Ctrl Pts',(-3.76803152185558,-0.46237689285949,
52.0986887042618));
#25837=CARTESIAN_POINT('Ctrl Pts',(-2.44593504675712,2.90332531801516,51.901178081079));
#25838=CARTESIAN_POINT('Ctrl Pts',(1.09537602710576,3.63483571356557,51.7036674578961));
#25839=CARTESIAN_POINT('Ctrl Pts',(3.64281991270102,1.06846205496556,51.5061568347132));
#25840=CARTESIAN_POINT('Ctrl Pts',(2.88519376829585,-2.46733825166162,51.3086462115304));
#25841=CARTESIAN_POINT('Ctrl Pts',(-0.49029695075581,-3.76450031773161,
51.1111355883475));
#25842=CARTESIAN_POINT('Ctrl Pts',(-3.42068936031018,-1.64616907805743,
50.9136249651647));
#25843=CARTESIAN_POINT('Ctrl Pts',(-3.24798942939275,1.96581371566414,50.7161143419817));
#25844=CARTESIAN_POINT('Ctrl Pts',(-0.127385446427556,3.79405049239167,
50.518603718799));
#25845=CARTESIAN_POINT('Ctrl Pts',(3.10679776192287,2.18026463175804,50.3210930956159));
#25846=CARTESIAN_POINT('Ctrl Pts',(3.52618489500465,-1.41231423648809,50.1235824724332));
#25847=CARTESIAN_POINT('Ctrl Pts',(0.738041645134074,-3.72228694315212,
49.9260718492503));
#25848=CARTESIAN_POINT('Ctrl Pts',(-1.55364532773234,-3.0114399702195,49.7943981004617));
#25849=CARTESIAN_POINT('Ctrl Pts',(-2.29850452099808,-2.25079075378251,
49.7285612260674));
#25850=CARTESIAN_POINT('',(3.07560303099836,-0.971134045656492,50.1404703033481));
#25851=CARTESIAN_POINT('Ctrl Pts',(3.07800019312434,-0.972037304811885,
50.1419356690201));
#25852=CARTESIAN_POINT('Ctrl Pts',(3.06227520141822,-1.05237632326202,50.1419356690201));
#25853=CARTESIAN_POINT('Ctrl Pts',(3.04333312529428,-1.13189057331352,50.1419356690201));
#25854=CARTESIAN_POINT('Ctrl Pts',(3.02115771737946,-1.21038988389693,50.1419356690201));
#25855=CARTESIAN_POINT('Ctrl Pts',(2.99336557492601,-1.30877202101979,50.1419356690201));
#25856=CARTESIAN_POINT('Ctrl Pts',(2.9604970300754,-1.40556061416761,50.1419356690201));
#25857=CARTESIAN_POINT('Ctrl Pts',(2.9229018831501,-1.50055476344149,50.1419356690201));
#25858=CARTESIAN_POINT('Ctrl Pts',(2.88423982723554,-1.59824474236563,50.1419356690201));
#25859=CARTESIAN_POINT('Ctrl Pts',(2.84057890699813,-1.69403760766469,50.1419356690201));
#25860=CARTESIAN_POINT('Ctrl Pts',(2.79224445502312,-1.78770962551524,50.1419356690202));
#25861=CARTESIAN_POINT('Ctrl Pts',(2.76578616493641,-1.83898570955108,50.1419356690202));
#25862=CARTESIAN_POINT('Ctrl Pts',(2.73792652669981,-1.88962614202262,50.1419356690202));
#25863=CARTESIAN_POINT('Ctrl Pts',(2.70871256304879,-1.93959251956205,50.1419356690202));
#25864=CARTESIAN_POINT('Ctrl Pts',(2.69706069008747,-1.95952141008791,50.1419356690202));
#25865=CARTESIAN_POINT('Ctrl Pts',(2.68519332639328,-1.97934305583239,50.1419356690202));
#25866=CARTESIAN_POINT('Ctrl Pts',(2.67311327275347,-1.99905494404161,50.1419356690202));
#25867=CARTESIAN_POINT('Ctrl Pts',(2.66446129450681,-2.01317299625164,50.1419356690202));
#25868=CARTESIAN_POINT('Ctrl Pts',(2.65570515937501,-2.02722665323309,50.1419356690202));
#25869=CARTESIAN_POINT('Ctrl Pts',(2.64684719817748,-2.04121370216548,50.1419356690202));
#25870=CARTESIAN_POINT('Ctrl Pts',(2.58908448250295,-2.13242317041571,50.1419356690202));
#25871=CARTESIAN_POINT('Ctrl Pts',(2.52698395322515,-2.22082070907395,50.1419356690202));
#25872=CARTESIAN_POINT('Ctrl Pts',(2.460918055731,-2.30618506499463,50.1419356690202));
#25873=CARTESIAN_POINT('Ctrl Pts',(2.39187403139581,-2.39539748609383,50.1419356690202));
#25874=CARTESIAN_POINT('Ctrl Pts',(2.31849891374532,-2.48129793395378,50.1419356690202));
#25875=CARTESIAN_POINT('Ctrl Pts',(2.24116020239773,-2.5636195351057,50.1419356690202));
#25876=CARTESIAN_POINT('Ctrl Pts',(2.16382149105007,-2.64594113625767,50.1419356690202));
#25877=CARTESIAN_POINT('Ctrl Pts',(2.08251855748945,-2.72468469072004,50.1419356690202));
#25878=CARTESIAN_POINT('Ctrl Pts',(1.99756923591343,-2.79955699478053,50.1419356690202));
#25879=CARTESIAN_POINT('Ctrl Pts',(1.97312667799664,-2.82110008181654,50.1419356690202));
#25880=CARTESIAN_POINT('Ctrl Pts',(1.94838195754849,-2.84232246238748,50.1419356690202));
#25881=CARTESIAN_POINT('Ctrl Pts',(1.9233419986283,-2.86321660162443,50.1419356690202));
#25882=CARTESIAN_POINT('Ctrl Pts',(1.91194750369415,-2.87272453110817,50.1419356690202));
#25883=CARTESIAN_POINT('Ctrl Pts',(1.90049372334605,-2.88216289265972,50.1419356690202));
#25884=CARTESIAN_POINT('Ctrl Pts',(1.88898826977189,-2.89152553551587,50.1419356690202));
#25885=CARTESIAN_POINT('Ctrl Pts',(1.80049123610051,-2.96354061208404,50.1419356690202));
#25886=CARTESIAN_POINT('Ctrl Pts',(1.70882666426025,-3.03117349173495,50.1419356690202));
#25887=CARTESIAN_POINT('Ctrl Pts',(1.61437075449497,-3.09417590432581,50.1419356690202));
#25888=CARTESIAN_POINT('Ctrl Pts',(1.51941266904254,-3.15751326980542,50.1419356690202));
#25889=CARTESIAN_POINT('Ctrl Pts',(1.42163289527908,-3.21617156831816,50.1419356690202));
#25890=CARTESIAN_POINT('Ctrl Pts',(1.3213682282809,-3.26987175410814,50.1419356690202));
#25891=CARTESIAN_POINT('Ctrl Pts',(1.2224245598561,-3.32286443374522,50.1419356690202));
#25892=CARTESIAN_POINT('Ctrl Pts',(1.12106035282451,-3.37102943937167,50.1419356690202));
#25893=CARTESIAN_POINT('Ctrl Pts',(1.01756488383265,-3.41406217225391,50.1419356690202));
#25894=CARTESIAN_POINT('Ctrl Pts',(0.966275322332376,-3.43538803338761,
50.1419356690202));
#25895=CARTESIAN_POINT('Ctrl Pts',(0.91446186828967,-3.45545281962562,50.1419356690202));
#25896=CARTESIAN_POINT('Ctrl Pts',(0.862157328497213,-3.47421531578325,
50.1419356690202));
#25897=CARTESIAN_POINT('Ctrl Pts',(0.81733495941787,-3.49029383460712,50.1419356690202));
#25898=CARTESIAN_POINT('Ctrl Pts',(0.772151923918596,-3.50541596154927,
50.1419356690202));
#25899=CARTESIAN_POINT('Ctrl Pts',(0.726628142940982,-3.51955390646554,
50.1419356690202));
#25900=CARTESIAN_POINT('Ctrl Pts',(0.718762362529219,-3.52199671696583,
50.1419356690202));
#25901=CARTESIAN_POINT('Ctrl Pts',(0.710888867590843,-3.52440937617116,
50.1419356690202));
#25902=CARTESIAN_POINT('Ctrl Pts',(0.703008125814777,-3.52679168831568,
50.1419356690202));
#25903=CARTESIAN_POINT('Ctrl Pts',(0.595193612326785,-3.55938352194457,
50.1419356690202));
#25904=CARTESIAN_POINT('Ctrl Pts',(0.486004814809058,-3.58630600421687,
50.1419356690202));
#25905=CARTESIAN_POINT('Ctrl Pts',(0.375834415117319,-3.60778456100658,
50.1419356690202));
#25906=CARTESIAN_POINT('Ctrl Pts',(0.265437021161436,-3.6293073720534,50.1419356690202));
#25907=CARTESIAN_POINT('Ctrl Pts',(0.154053290098907,-3.64536375893427,
50.1419356690202));
#25908=CARTESIAN_POINT('Ctrl Pts',(0.0420494266149386,-3.65613226637667,
50.1419356690202));
#25909=CARTESIAN_POINT('Ctrl Pts',(-0.0727136961382722,-3.66716606023914,
50.1419356690202));
#25910=CARTESIAN_POINT('Ctrl Pts',(-0.188128572258745,-3.67264837361943,
50.1419356690202));
#25911=CARTESIAN_POINT('Ctrl Pts',(-0.303821229732827,-3.67271959388211,
50.1419356690202));
#25912=CARTESIAN_POINT('Ctrl Pts',(-0.413254182712562,-3.67278696067813,
50.1419356690202));
#25913=CARTESIAN_POINT('Ctrl Pts',(-0.522936411188278,-3.66801249049235,
50.1419356690202));
#25914=CARTESIAN_POINT('Ctrl Pts',(-0.632558318696721,-3.65847265496365,
50.1419356690202));
#25915=CARTESIAN_POINT('Ctrl Pts',(-0.656240589624941,-3.65641170770651,
50.1419356690202));
#25916=CARTESIAN_POINT('Ctrl Pts',(-0.679926094463313,-3.65412746565096,
50.1419356690202));
#25917=CARTESIAN_POINT('Ctrl Pts',(-0.703578099800705,-3.65162429841491,
50.1419356690202));
#25918=CARTESIAN_POINT('Ctrl Pts',(-0.822930318687432,-3.63899287204724,
50.1419356690202));
#25919=CARTESIAN_POINT('Ctrl Pts',(-0.941557594243896,-3.62078266779788,
50.1419356690202));
#25920=CARTESIAN_POINT('Ctrl Pts',(-1.05905125671003,-3.59719277930163,
50.1419356690202));
#25921=CARTESIAN_POINT('Ctrl Pts',(-1.17679134286499,-3.57355341488284,
50.1419356690202));
#25922=CARTESIAN_POINT('Ctrl Pts',(-1.29339391787156,-3.54451169179539,
50.1419356690202));
#25923=CARTESIAN_POINT('Ctrl Pts',(-1.40846037353927,-3.51021482329977,
50.1419356690202));
#25924=CARTESIAN_POINT('Ctrl Pts',(-1.52316558732171,-3.47602562706504,
50.1419356690202));
#25925=CARTESIAN_POINT('Ctrl Pts',(-1.63634518520109,-3.43661410589424,
50.1419356690202));
#25926=CARTESIAN_POINT('Ctrl Pts',(-1.74760384492387,-3.39207497720295,
50.1419356690202));
#25927=CARTESIAN_POINT('Ctrl Pts',(-1.8032331747853,-3.36980541285729,50.1419356690202));
#25928=CARTESIAN_POINT('Ctrl Pts',(-1.85838218161433,-3.34625315838058,
50.1419356690202));
#25929=CARTESIAN_POINT('Ctrl Pts',(-1.91300035582,-3.32142538195897,50.1419356690202));
#25930=CARTESIAN_POINT('Ctrl Pts',(-1.94936455815574,-3.30489531118176,
50.1419356690202));
#25931=CARTESIAN_POINT('Ctrl Pts',(-1.98549343725982,-3.28779976900701,
50.1419356690202));
#25932=CARTESIAN_POINT('Ctrl Pts',(-2.02137178270244,-3.27014011787672,
50.1419356690202));
#25933=CARTESIAN_POINT('Ctrl Pts',(-2.03938186587157,-3.26127538953792,
50.1419356690202));
#25934=CARTESIAN_POINT('Ctrl Pts',(-2.05733089912592,-3.252267440223,50.1419356690202));
#25935=CARTESIAN_POINT('Ctrl Pts',(-2.07521052413803,-3.24311966611299,
50.1419356690202));
#25936=CARTESIAN_POINT('Ctrl Pts',(-2.18541124809655,-3.1867375367982,50.1419356690202));
#25937=CARTESIAN_POINT('Ctrl Pts',(-2.29261698285448,-3.12523274643722,
50.1419356690202));
#25938=CARTESIAN_POINT('Ctrl Pts',(-2.3964196822934,-3.05876555109958,50.1419356690202));
#25939=CARTESIAN_POINT('Ctrl Pts',(-2.49996259686187,-2.99246470183795,
50.1419356690201));
#25940=CARTESIAN_POINT('Ctrl Pts',(-2.60012039529287,-2.92122610018819,
50.1419356690201));
#25941=CARTESIAN_POINT('Ctrl Pts',(-2.69648100191037,-2.84515796161608,
50.1419356690201));
#25942=CARTESIAN_POINT('Ctrl Pts',(-2.73495674613104,-2.81478477960966,
50.1419356690201));
#25943=CARTESIAN_POINT('Ctrl Pts',(-2.77282694295787,-2.78364105966542,
50.1419356690201));
#25944=CARTESIAN_POINT('Ctrl Pts',(-2.81006454495679,-2.75173150091943,
50.1419356690201));
#25945=CARTESIAN_POINT('Ctrl Pts',(3.08633327008855,-0.927720059309073,
50.1419356690201));
#25946=CARTESIAN_POINT('Ctrl Pts',(3.08205063481698,-0.941967503448788,
50.1414472137961));
#25947=CARTESIAN_POINT('Ctrl Pts',(3.07766934222995,-0.956185292203961,
50.1409587585721));
#25948=CARTESIAN_POINT('Ctrl Pts',(3.0731898124641,-0.970372062183785,50.1404703033481));
#25949=CARTESIAN_POINT('Ctrl Pts',(3.22243683749933,-0.0449265047301374,
60.1999356690201));
#25950=CARTESIAN_POINT('Ctrl Pts',(3.23190969153617,-0.146959477571174,
60.1999356690201));
#25951=CARTESIAN_POINT('Ctrl Pts',(3.23609830245048,-0.249183173425684,
60.1999356690201));
#25952=CARTESIAN_POINT('Ctrl Pts',(3.23526888419945,-0.351287921296696,
60.1999356690201));
#25953=CARTESIAN_POINT('Ctrl Pts',(3.23441346753709,-0.456593178958777,
60.19993566902));
#25954=CARTESIAN_POINT('Ctrl Pts',(3.22822059903152,-0.561772520799036,
60.19993566902));
#25955=CARTESIAN_POINT('Ctrl Pts',(3.21692873692298,-0.666504456816874,
60.19993566902));
#25956=CARTESIAN_POINT('Ctrl Pts',(3.205645923797,-0.771152463589466,60.1999356690201));
#25957=CARTESIAN_POINT('Ctrl Pts',(3.18927208808766,-0.875354527570815,
60.19993566902));
#25958=CARTESIAN_POINT('Ctrl Pts',(3.16799367544636,-0.978797438385924,
60.19993566902));
#25959=CARTESIAN_POINT('Ctrl Pts',(3.16387062690766,-0.99884123345022,60.19993566902));
#25960=CARTESIAN_POINT('Ctrl Pts',(3.15956328353731,-1.01885652861755,60.19993566902));
#25961=CARTESIAN_POINT('Ctrl Pts',(3.155072787946,-1.03884104070003,60.19993566902));
#25962=CARTESIAN_POINT('Ctrl Pts',(3.15075715067165,-1.05804736291971,60.19993566902));
#25963=CARTESIAN_POINT('Ctrl Pts',(3.1462740972738,-1.0772172541688,60.19993566902));
#25964=CARTESIAN_POINT('Ctrl Pts',(3.14162701596928,-1.09634105452731,60.19993566902));
#25965=CARTESIAN_POINT('Ctrl Pts',(3.11602725935698,-1.20168989664972,60.19993566902));
#25966=CARTESIAN_POINT('Ctrl Pts',(3.08543783388726,-1.30571176782322,60.19993566902));
#25967=CARTESIAN_POINT('Ctrl Pts',(3.0501086657506,-1.40807351735763,60.19993566902));
#25968=CARTESIAN_POINT('Ctrl Pts',(3.01408121476251,-1.51245845221204,60.19993566902));
#25969=CARTESIAN_POINT('Ctrl Pts',(2.97312473432208,-1.61511781792578,60.19993566902));
#25970=CARTESIAN_POINT('Ctrl Pts',(2.92745013565406,-1.71570108022376,60.19993566902));
#25971=CARTESIAN_POINT('Ctrl Pts',(2.89842288396775,-1.77962404299296,60.19993566902));
#25972=CARTESIAN_POINT('Ctrl Pts',(2.86748894951469,-1.84270850865144,60.19993566902));
#25973=CARTESIAN_POINT('Ctrl Pts',(2.83469170847284,-1.90486266936677,60.19993566902));
#25974=CARTESIAN_POINT('Ctrl Pts',(2.81595808148896,-1.94036482824812,60.19993566902));
#25975=CARTESIAN_POINT('Ctrl Pts',(2.79661637492879,-1.97556342443468,60.19993566902));
#25976=CARTESIAN_POINT('Ctrl Pts',(2.77667350924734,-2.01044092927213,60.19993566902));
#25977=CARTESIAN_POINT('Ctrl Pts',(2.76841891872605,-2.02487714548278,60.19993566902));
#25978=CARTESIAN_POINT('Ctrl Pts',(2.76006622223582,-2.03924977505433,60.19993566902));
#25979=CARTESIAN_POINT('Ctrl Pts',(2.7516167194928,-2.053556959919,60.19993566902));
#25980=CARTESIAN_POINT('Ctrl Pts',(2.69392882598369,-2.15123742491092,60.19993566902));
#25981=CARTESIAN_POINT('Ctrl Pts',(2.63172633617838,-2.24587894137787,60.19993566902));
#25982=CARTESIAN_POINT('Ctrl Pts',(2.56525668975559,-2.33712629647658,60.19993566902));
#25983=CARTESIAN_POINT('Ctrl Pts',(2.49866320152646,-2.42854365755376,60.19993566902));
#25984=CARTESIAN_POINT('Ctrl Pts',(2.42778635625904,-2.51655510291817,60.19993566902));
#25985=CARTESIAN_POINT('Ctrl Pts',(2.35282359530363,-2.60079329271395,60.19993566902));
#25986=CARTESIAN_POINT('Ctrl Pts',(2.27928471630906,-2.68343141819332,60.19993566902));
#25987=CARTESIAN_POINT('Ctrl Pts',(2.20181324314207,-2.76243906231675,60.19993566902));
#25988=CARTESIAN_POINT('Ctrl Pts',(2.1205516927396,-2.83744719687121,60.19993566902));
#25989=CARTESIAN_POINT('Ctrl Pts',(2.05269464105882,-2.90008236489019,60.19993566902));
#25990=CARTESIAN_POINT('Ctrl Pts',(1.98219392384327,-2.95992853986898,60.19993566902));
#25991=CARTESIAN_POINT('Ctrl Pts',(1.90911141620034,-3.01675254204845,60.19993566902));
#25992=CARTESIAN_POINT('Ctrl Pts',(1.89622466318962,-3.02677240733202,60.19993566902));
#25993=CARTESIAN_POINT('Ctrl Pts',(1.88325740636086,-3.03669830080153,60.19993566902));
#25994=CARTESIAN_POINT('Ctrl Pts',(1.87022294168935,-3.04652123647435,60.19993566902));
#25995=CARTESIAN_POINT('Ctrl Pts',(1.78116472099078,-3.1136366259517,60.19993566902));
#25996=CARTESIAN_POINT('Ctrl Pts',(1.68883725354168,-3.1760549216553,60.19993566902));
#25997=CARTESIAN_POINT('Ctrl Pts',(1.59369488622457,-3.2338371928481,60.19993566902));
#25998=CARTESIAN_POINT('Ctrl Pts',(1.49780680382872,-3.29207235492567,60.19993566902));
#25999=CARTESIAN_POINT('Ctrl Pts',(1.39905888922488,-3.34559878068317,60.19993566902));
#26000=CARTESIAN_POINT('Ctrl Pts',(1.29787166956309,-3.39444464211518,60.19993566902));
#26001=CARTESIAN_POINT('Ctrl Pts',(1.19409883891314,-3.44453864927613,60.19993566902));
#26002=CARTESIAN_POINT('Ctrl Pts',(1.08775982993701,-3.48971023405494,60.19993566902));
#26003=CARTESIAN_POINT('Ctrl Pts',(0.9792709270014,-3.52994870798746,60.19993566902));
#26004=CARTESIAN_POINT('Ctrl Pts',(0.87865632453916,-3.56726660824138,60.19993566902));
#26005=CARTESIAN_POINT('Ctrl Pts',(0.776191695095459,-3.6003412563449,60.19993566902));
#26006=CARTESIAN_POINT('Ctrl Pts',(0.672189142038902,-3.62912941459683,
60.19993566902));
#26007=CARTESIAN_POINT('Ctrl Pts',(0.650407555589505,-3.63515861041226,
60.19993566902));
#26008=CARTESIAN_POINT('Ctrl Pts',(0.62855355524072,-3.64100084058666,60.19993566902));
#26009=CARTESIAN_POINT('Ctrl Pts',(0.606659738943875,-3.64664810681024,
60.19993566902));
#26010=CARTESIAN_POINT('Ctrl Pts',(0.491699373233907,-3.67630085357315,
60.19993566902));
#26011=CARTESIAN_POINT('Ctrl Pts',(0.375508042115669,-3.70062174153854,
60.19993566902));
#26012=CARTESIAN_POINT('Ctrl Pts',(0.258541788795668,-3.71964227030934,
60.19993566902));
#26013=CARTESIAN_POINT('Ctrl Pts',(0.140091959710903,-3.738904051533,60.19993566902));
#26014=CARTESIAN_POINT('Ctrl Pts',(0.0208466229849164,-3.7527304787693,
60.19993566902));
#26015=CARTESIAN_POINT('Ctrl Pts',(-0.098751394978667,-3.76110953310029,
60.19993566902));
#26016=CARTESIAN_POINT('Ctrl Pts',(-0.218381330657788,-3.76949082359101,
60.19993566902));
#26017=CARTESIAN_POINT('Ctrl Pts',(-0.338365031743393,-3.7724220719954,
60.19993566902));
#26018=CARTESIAN_POINT('Ctrl Pts',(-0.458277031791744,-3.76984273951047,
60.19993566902));
#26019=CARTESIAN_POINT('Ctrl Pts',(-0.557812449297683,-3.76770171162611,
60.19993566902));
#26020=CARTESIAN_POINT('Ctrl Pts',(-0.657299034614091,-3.7617630037591,
60.19993566902));
#26021=CARTESIAN_POINT('Ctrl Pts',(-0.756495963167153,-3.75196478708744,
60.19993566902));
#26022=CARTESIAN_POINT('Ctrl Pts',(-0.775448827008612,-3.7500927103087,
60.19993566902));
#26023=CARTESIAN_POINT('Ctrl Pts',(-0.794391113280761,-3.74807966670157,
60.19993566902));
#26024=CARTESIAN_POINT('Ctrl Pts',(-0.813321133086311,-3.74592511735631,
60.19993566902));
#26025=CARTESIAN_POINT('Ctrl Pts',(-0.828796076691622,-3.74416381282756,
60.19993566902));
#26026=CARTESIAN_POINT('Ctrl Pts',(-0.844252778619867,-3.74230909014765,
60.19993566902));
#26027=CARTESIAN_POINT('Ctrl Pts',(-0.85969142305059,-3.74036085764192,
60.19993566902));
#26028=CARTESIAN_POINT('Ctrl Pts',(-0.982113292440273,-3.72491220433385,
60.19993566902));
#26029=CARTESIAN_POINT('Ctrl Pts',(-1.10337504609058,-3.70359051818525,
60.19993566902));
#26030=CARTESIAN_POINT('Ctrl Pts',(-1.22302031683542,-3.6763861302258,60.19993566902));
#26031=CARTESIAN_POINT('Ctrl Pts',(-1.34198409077688,-3.64933669785562,
60.19993566902));
#26032=CARTESIAN_POINT('Ctrl Pts',(-1.45935068501764,-3.6164715536994,60.1999356690201));
#26033=CARTESIAN_POINT('Ctrl Pts',(-1.57468060825087,-3.57773092054377,
60.19993566902));
#26034=CARTESIAN_POINT('Ctrl Pts',(-1.59224316998028,-3.57183145627502,
60.19993566902));
#26035=CARTESIAN_POINT('Ctrl Pts',(-1.6097585039616,-3.5657956440463,60.19993566902));
#26036=CARTESIAN_POINT('Ctrl Pts',(-1.62722505555305,-3.55962316586745,
60.1999356690201));
#26037=CARTESIAN_POINT('Ctrl Pts',(-1.7202915870815,-3.52673452542617,60.1999356690201));
#26038=CARTESIAN_POINT('Ctrl Pts',(-1.81197361471366,-3.48996787671853,
60.1999356690201));
#26039=CARTESIAN_POINT('Ctrl Pts',(-1.90215316220673,-3.44952007606408,
60.1999356690201));
#26040=CARTESIAN_POINT('Origin',(-1.041818884589E-14,0.,50.1419356690201));
#26041=CARTESIAN_POINT('Origin',(-1.16499385964724E-14,0.,60.1999356690201));
#34390=UNCERTAINTY_MEASURE_WITH_UNIT(LENGTH_MEASURE(0.01),#34404,
'DISTANCE_ACCURACY_VALUE',
'Maximum model space distance between geometric entities at asserted c
onnectivities');
#34393=UNCERTAINTY_MEASURE_WITH_UNIT(LENGTH_MEASURE(0.01),#34404,
'DISTANCE_ACCURACY_VALUE',
'Maximum model space distance between geometric entities at asserted c
onnectivities');
#34400=(
GEOMETRIC_REPRESENTATION_CONTEXT(3)
GLOBAL_UNCERTAINTY_ASSIGNED_CONTEXT((#34390))
GLOBAL_UNIT_ASSIGNED_CONTEXT((#34404,#34406,#34407))
REPRESENTATION_CONTEXT('','3D')
);
#34403=(
GEOMETRIC_REPRESENTATION_CONTEXT(3)
GLOBAL_UNCERTAINTY_ASSIGNED_CONTEXT((#34393))
GLOBAL_UNIT_ASSIGNED_CONTEXT((#34404,#34406,#34407))
REPRESENTATION_CONTEXT('','3D')
);
#34404=(
LENGTH_UNIT()
NAMED_UNIT(*)
SI_UNIT(.MILLI.,.METRE.)
);
#34406=(
NAMED_UNIT(*)
PLANE_ANGLE_UNIT()
SI_UNIT($,.RADIAN.)
);
#34407=(
NAMED_UNIT(*)
SI_UNIT($,.STERADIAN.)
SOLID_ANGLE_UNIT()
);
#34414=SHAPE_DEFINITION_REPRESENTATION(#34423,#34440);
#34423=PRODUCT_DEFINITION_SHAPE('',$,#34450);
#34440=SHAPE_REPRESENTATION('',(#4579),#34400);
#34443=PRODUCT_DEFINITION_CONTEXT('part definition',#34472,'design');
#34450=PRODUCT_DEFINITION('Bushing_02','Bushing_02',#34459,#34443);
#34459=PRODUCT_DEFINITION_FORMATION('',$,#34480);
#34472=APPLICATION_CONTEXT(
'Core Data for Automotive Mechanical Design Process');
#34473=PRODUCT_CONTEXT('part definition',#34472,'mechanical');
#34480=PRODUCT('Bushing_02','Bushing_02',$,(#34473));
#34484=PRESENTATION_STYLE_ASSIGNMENT((#34486));
#34486=SURFACE_STYLE_USAGE(.BOTH.,#34488);
#34488=SURFACE_SIDE_STYLE('',(#34490));
#34490=SURFACE_STYLE_FILL_AREA(#34492);
#34492=FILL_AREA_STYLE('Opaque(160,160,160)',(#34494));
#34494=FILL_AREA_STYLE_COLOUR('Opaque(160,160,160)',#34496);
#34496=COLOUR_RGB('Opaque(160,160,160)', 0.09019608, 0.27058824, 0.51372549);
ENDSEC;
END-ISO-10303-21;
